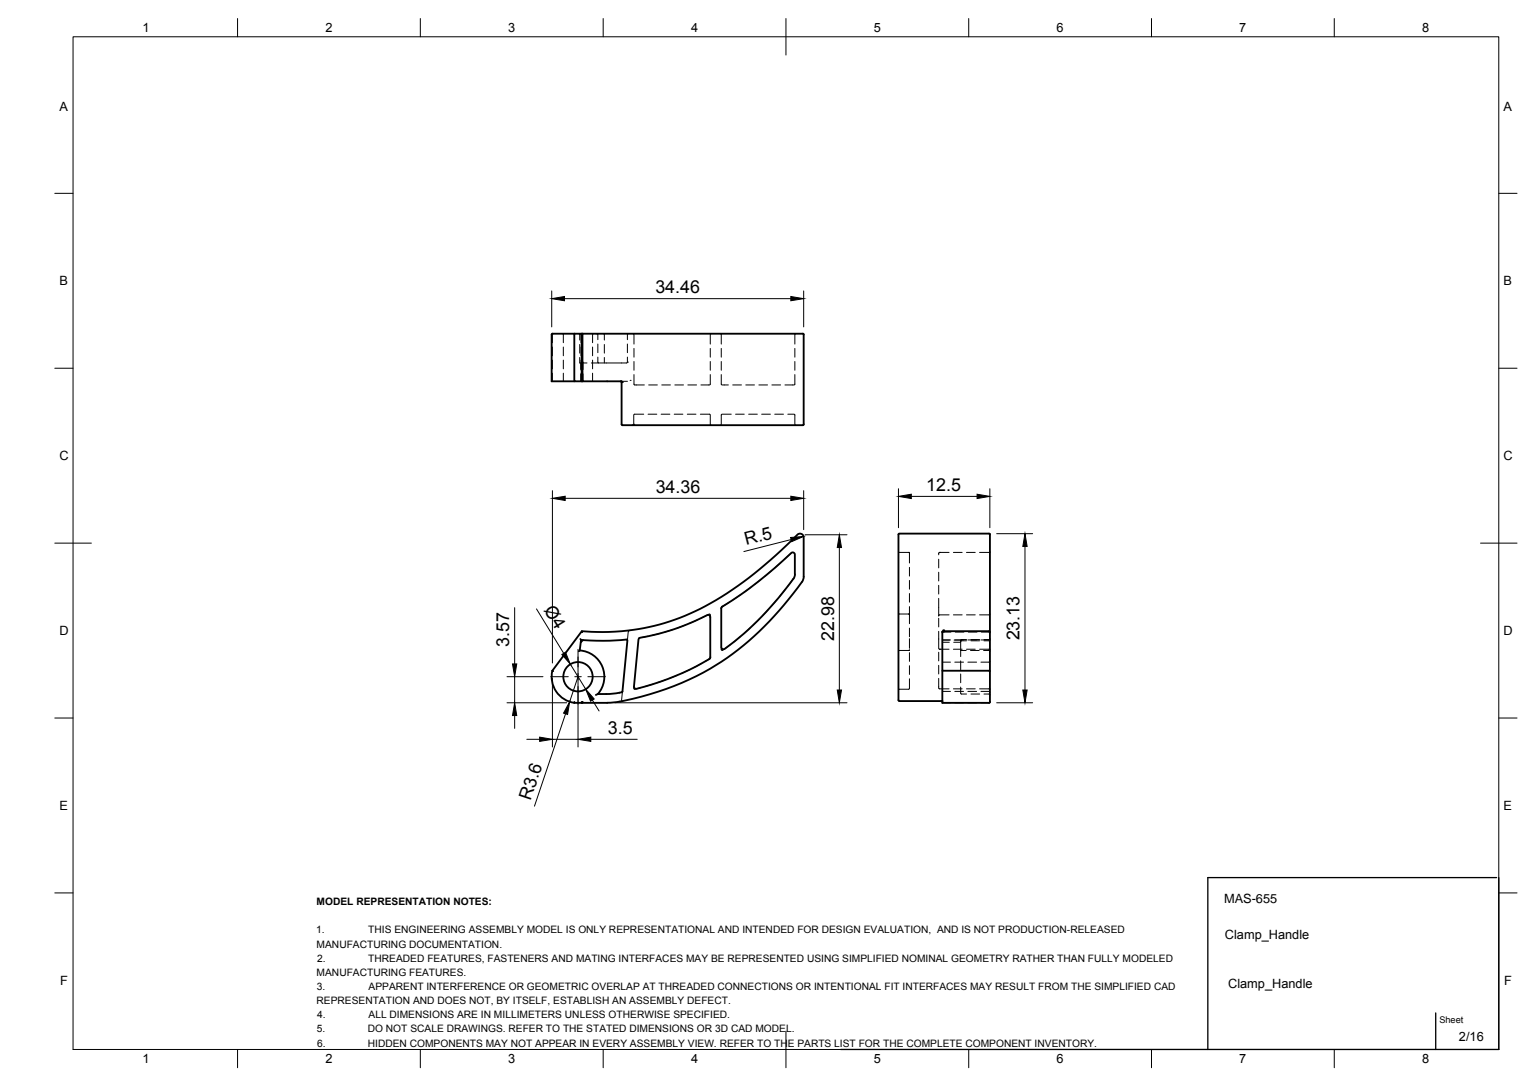
ISO-10303-21;
HEADER;
FILE_DESCRIPTION((''),'2;1');
FILE_NAME('Clamp_Handle.step','2026-10-09T11:34:15-07:00',(''),(''),'','','');
FILE_SCHEMA (('AUTOMOTIVE_DESIGN { 1 0 10303 214 3 1 1 }'));
ENDSEC;
DATA;
#10=MECHANICAL_DESIGN_GEOMETRIC_PRESENTATION_REPRESENTATION('',(#629),#117170);
#103=ELLIPSE('',#49876,30.621208525322,25.4809915026997) ;
#104=ELLIPSE('',#49877,31.5888201684124,25.5766704752798) ;
#105=ELLIPSE('',#49879,31.5675675201038,25.5487669653367) ;
#106=ELLIPSE('',#49885,0.87450775194086,0.752188335062039) ;
#107=ELLIPSE('',#49887,0.979448682193676,0.842450935309832) ;
#108=ELLIPSE('',#49892,0.26650610321202,0.226790790063564) ;
#109=ELLIPSE('',#49893,0.373108544497893,0.31750710609267) ;
#110=ELLIPSE('',#49894,0.874507751946099,0.752188335070988) ;
#111=ELLIPSE('',#49899,104.965032228634,60.1468662540866) ;
#112=ELLIPSE('',#49900,153.912764893179,72.1332927979209) ;
#113=ELLIPSE('',#49901,107.003369056671,53.394874735838) ;
#114=ELLIPSE('',#49903,0.944305135734821,0.812323833839972) ;
#115=ELLIPSE('',#49904,31.6658812357246,25.6468027651175) ;
#116=ELLIPSE('',#49905,33.3290082029849,26.9991094930833) ;
#117=ELLIPSE('',#49908,0.373067574458494,0.317497630618124) ;
#118=ELLIPSE('',#49909,87.539485717233,47.1288613191233) ;
#119=ELLIPSE('',#49910,28.9052201415572,24.2407648329214) ;
#120=ELLIPSE('',#49911,33.8387106683363,27.6581069858551) ;
#121=ELLIPSE('',#49912,32.4705877660237,26.389680540433) ;
#122=ELLIPSE('',#49913,119.941732153885,63.5628286542732) ;
#123=ELLIPSE('',#49920,0.266476838896091,0.226784021864154) ;
#124=ELLIPSE('',#49928,0.266476838896308,0.226784021864664) ;
#125=ELLIPSE('',#49936,0.120304939822837,0.120009764468753) ;
#126=ELLIPSE('',#49937,0.120304939823071,0.120009764469075) ;
#127=ELLIPSE('',#49944,32.9935493519598,26.6864661964081) ;
#128=ELLIPSE('',#49946,31.5675675494409,25.5487669922883) ;
#129=ELLIPSE('',#49953,1.04922792860613,0.902582037621626) ;
#130=ELLIPSE('',#49958,106.937521398911,53.4980353026644) ;
#131=ELLIPSE('',#49960,171.400384709509,76.7143149375333) ;
#132=ELLIPSE('',#49962,112.686599872101,62.8742365573781) ;
#133=ELLIPSE('',#49966,0.124835932303391,0.12) ;
#134=ELLIPSE('',#49972,106.937521398833,53.4980353026422) ;
#135=ELLIPSE('',#49973,26.7718235298462,13.2260955102084) ;
#136=ELLIPSE('',#49974,180.168079206207,78.5747283099703) ;
#137=ELLIPSE('',#49975,26.5629631306412,13.0416514063261) ;
#138=ELLIPSE('',#49997,34.0017819463872,27.818723289359) ;
#139=ELLIPSE('',#49999,33.6804890520093,27.5067870175508) ;
#140=ELLIPSE('',#50000,32.5228044782183,26.4447063399665) ;
#141=ELLIPSE('',#50001,32.6276108313175,26.5480371159551) ;
#142=ELLIPSE('',#50004,33.6121963166486,28.1464718973248) ;
#143=ELLIPSE('',#50007,34.1688903664586,27.9750858992831) ;
#144=ELLIPSE('',#50008,32.5764457907704,26.4940988115262) ;
#145=ELLIPSE('',#50009,121.638689200547,63.8567625922291) ;
#146=ELLIPSE('',#50011,133.068922302088,67.3695526852953) ;
#147=ELLIPSE('',#50017,110.759696058364,60.5332237301847) ;
#148=ELLIPSE('',#50022,26.0480895445502,18.516397692244) ;
#149=ELLIPSE('',#50026,112.783598469003,61.0762817351653) ;
#150=ELLIPSE('',#50031,89.0710500040395,47.3896547267835) ;
#151=ELLIPSE('',#50033,0.159886103339097,0.136070413122481) ;
#152=ELLIPSE('',#50037,29.4480227809696,24.8646228837011) ;
#153=ELLIPSE('',#50046,0.76956682169275,0.66192573483117) ;
#154=ELLIPSE('',#50052,0.159903661928928,0.13607447404265) ;
#155=ELLIPSE('',#50053,0.266506103215596,0.226790790070262) ;
#156=ELLIPSE('',#50061,0.129795981335339,0.124487164214877) ;
#157=ELLIPSE('',#50071,0.769566821716286,0.661925734873078) ;
#158=ELLIPSE('',#50073,0.874507751919452,0.75218833502354) ;
#159=ELLIPSE('',#50077,0.210854308776711,0.181549488975955) ;
#160=ELLIPSE('',#50081,0.874507751937288,0.752188335055131) ;
#161=ELLIPSE('',#50083,0.97944868220323,0.842450935327434) ;
#162=ELLIPSE('',#50090,160.893031132199,73.683653149258) ;
#163=ELLIPSE('',#50091,0.944305135733765,0.812323833838177) ;
#164=ELLIPSE('',#50093,107.003369056713,53.3948747358502) ;
#165=ELLIPSE('',#50103,0.129786651823771,0.12448808595579) ;
#166=ELLIPSE('',#50123,90.0915709695949,47.7382908134221) ;
#167=ELLIPSE('',#50124,89.6335580246405,47.7081104258241) ;
#168=ELLIPSE('',#50133,33.329008202931,26.9991094930345) ;
#169=ELLIPSE('',#50134,32.993549352048,26.6864661964888) ;
#170=ELLIPSE('',#50146,1.04922792859238,0.902582037596269) ;
#587=SHAPE_REPRESENTATION_RELATIONSHIP('SRR','None',#117242,#608) ;
#608=ADVANCED_BREP_SHAPE_REPRESENTATION('',(#650),#117150) ;
#629=STYLED_ITEM('',(#117355),#650) ;
#650=MANIFOLD_SOLID_BREP('Body1',#49058) ;
#671=FACE_BOUND('',#14121,.T.) ;
#672=FACE_BOUND('',#14122,.T.) ;
#673=FACE_BOUND('',#14123,.T.) ;
#674=FACE_BOUND('',#14124,.T.) ;
#675=FACE_BOUND('',#14239,.T.) ;
#676=FACE_BOUND('',#14240,.T.) ;
#677=FACE_BOUND('',#14304,.T.) ;
#678=FACE_BOUND('',#14305,.T.) ;
#895=B_SPLINE_CURVE_WITH_KNOTS('',3,(#75340,#75341,#75342,#75343),
 .UNSPECIFIED.,.F.,.F.,(4,4),(0.,0.0304960917345408),.UNSPECIFIED.) ;
#896=B_SPLINE_CURVE_WITH_KNOTS('',3,(#75345,#75346,#75347,#75348,#75349,
#75350),.UNSPECIFIED.,.F.,.F.,(4,2,4),(0.0304960917345408,0.0307213705840096,
0.0308468428281894),.UNSPECIFIED.) ;
#897=B_SPLINE_CURVE_WITH_KNOTS('',3,(#75351,#75352,#75353,#75354,#75355,
#75356),.UNSPECIFIED.,.F.,.F.,(4,2,4),(-0.0308468428281894,-0.0307213705840096,
0.),.UNSPECIFIED.) ;
#898=B_SPLINE_CURVE_WITH_KNOTS('',3,(#75428,#75429,#75430,#75431,#75432,
#75433,#75434,#75435,#75436,#75437),.UNSPECIFIED.,.F.,.F.,(4,2,2,2,4),(-9.50158063795107E-5,
-3.3802014536195E-10,0.0116383704253253,0.0168222452993766,0.0213033382245776),
 .UNSPECIFIED.) ;
#899=B_SPLINE_CURVE_WITH_KNOTS('',3,(#75438,#75439,#75440,#75441,#75442),
 .UNSPECIFIED.,.F.,.F.,(4,1,4),(0.0251851760390954,0.0320842381312984,0.0449179333838473),
 .UNSPECIFIED.) ;
#900=B_SPLINE_CURVE_WITH_KNOTS('',3,(#75443,#75444,#75445,#75446,#75447,
#75448),.UNSPECIFIED.,.F.,.F.,(4,1,1,4),(0.,0.5,0.714285714285714,1.),
 .UNSPECIFIED.) ;
#901=B_SPLINE_CURVE_WITH_KNOTS('',3,(#75474,#75475,#75476,#75477,#75478),
 .UNSPECIFIED.,.F.,.F.,(4,1,4),(-0.0228171701215865,-0.0097787952834712,
0.),.UNSPECIFIED.) ;
#902=B_SPLINE_CURVE_WITH_KNOTS('',3,(#75479,#75480,#75481,#75482,#75483,
#75484,#75485,#75486,#75487,#75488,#75489,#75490,#75491,#75492,#75493,#75494,
#75495,#75496,#75497),.UNSPECIFIED.,.F.,.F.,(4,3,3,3,3,3,4),(7.84710342600197E-9,
0.00635871960742978,0.00765411709399715,0.0097787952834712,0.0153829015724535,
0.0211032796709813,0.0228171889947661),.UNSPECIFIED.) ;
#903=B_SPLINE_CURVE_WITH_KNOTS('',3,(#75516,#75517,#75518,#75519,#75520),
 .UNSPECIFIED.,.F.,.F.,(4,1,4),(-1.,-0.571428571428571,0.),
 .UNSPECIFIED.) ;
#904=B_SPLINE_CURVE_WITH_KNOTS('',3,(#75589,#75590,#75591,#75592),
 .UNSPECIFIED.,.F.,.F.,(4,4),(-1.19261278278549,0.),.UNSPECIFIED.) ;
#905=B_SPLINE_CURVE_WITH_KNOTS('',3,(#75595,#75596,#75597,#75598),
 .UNSPECIFIED.,.F.,.F.,(4,4),(0.,1.19261278278549),.UNSPECIFIED.) ;
#906=B_SPLINE_CURVE_WITH_KNOTS('',3,(#75630,#75631,#75632,#75633,#75634,
#75635),.UNSPECIFIED.,.F.,.F.,(4,1,1,4),(-0.0977650255444303,-0.0698321611031645,
-0.0418992966618987,0.),.UNSPECIFIED.) ;
#907=B_SPLINE_CURVE_WITH_KNOTS('',3,(#75638,#75639,#75640,#75641,#75642,
#75643),.UNSPECIFIED.,.F.,.F.,(4,1,1,4),(0.,0.0418992966618987,0.0698321611031645,
0.0977650255444303),.UNSPECIFIED.) ;
#908=B_SPLINE_CURVE_WITH_KNOTS('',3,(#75698,#75699,#75700,#75701),
 .UNSPECIFIED.,.F.,.F.,(4,4),(-1.35181237759077,-5.11404103536248E-14),
 .UNSPECIFIED.) ;
#909=B_SPLINE_CURVE_WITH_KNOTS('',3,(#75702,#75703,#75704,#75705),
 .UNSPECIFIED.,.F.,.F.,(4,4),(5.11404103536248E-14,1.35181237759077),
 .UNSPECIFIED.) ;
#910=B_SPLINE_CURVE_WITH_KNOTS('',3,(#75737,#75738,#75739,#75740,#75741,
#75742),.UNSPECIFIED.,.F.,.F.,(4,1,1,4),(-0.0921161357255624,-0.0657972398039731,
-0.0394783438823839,0.),.UNSPECIFIED.) ;
#911=B_SPLINE_CURVE_WITH_KNOTS('',3,(#75745,#75746,#75747,#75748,#75749,
#75750),.UNSPECIFIED.,.F.,.F.,(4,1,1,4),(0.,0.0394783438823839,0.0657972398039731,
0.0921161357255624),.UNSPECIFIED.) ;
#912=B_SPLINE_CURVE_WITH_KNOTS('',3,(#75812,#75813,#75814,#75815,#75816,
#75817,#75818),.UNSPECIFIED.,.F.,.F.,(4,1,1,1,4),(-1.,-0.857142857142857,
-0.571428571428571,-0.285714285714286,0.),.UNSPECIFIED.) ;
#913=B_SPLINE_CURVE_WITH_KNOTS('',3,(#75829,#75830,#75831,#75832),
 .UNSPECIFIED.,.F.,.F.,(4,4),(-1.19778613661182,0.),.UNSPECIFIED.) ;
#914=B_SPLINE_CURVE_WITH_KNOTS('',3,(#75854,#75855,#75856,#75857,#75858),
 .UNSPECIFIED.,.F.,.F.,(4,1,4),(-1.5574419802933,-0.667475134411416,0.),
 .UNSPECIFIED.) ;
#915=B_SPLINE_CURVE_WITH_KNOTS('',3,(#75864,#75865,#75866,#75867,#75868,
#75869,#75870),.UNSPECIFIED.,.F.,.F.,(4,1,1,1,4),(3.75975382637766E-15,
0.0255939875922149,0.051187975184426,0.0639849689805315,0.0895789565727426),
 .UNSPECIFIED.) ;
#916=B_SPLINE_CURVE_WITH_KNOTS('',3,(#75872,#75873,#75874,#75875,#75876),
 .UNSPECIFIED.,.F.,.F.,(4,1,4),(-1.52552518986177,-0.653796509940758,0.),
 .UNSPECIFIED.) ;
#917=B_SPLINE_CURVE_WITH_KNOTS('',3,(#75878,#75879,#75880,#75881,#75882),
 .UNSPECIFIED.,.F.,.F.,(4,1,4),(-1.19232799652366,-0.510997712795854,0.),
 .UNSPECIFIED.) ;
#918=B_SPLINE_CURVE_WITH_KNOTS('',3,(#75900,#75901,#75902,#75903,#75904,
#75905),.UNSPECIFIED.,.F.,.F.,(4,1,1,4),(0.,0.0345437068826219,0.0575728448043699,
0.0806019827261179),.UNSPECIFIED.) ;
#919=B_SPLINE_CURVE_WITH_KNOTS('',3,(#75909,#75910,#75911,#75912,#75913),
 .UNSPECIFIED.,.F.,.F.,(4,1,4),(0.,0.0235485345716834,0.0549465806672613),
 .UNSPECIFIED.) ;
#920=B_SPLINE_CURVE_WITH_KNOTS('',3,(#75916,#75917,#75918,#75919,#75920,
#75921),.UNSPECIFIED.,.F.,.F.,(4,1,1,4),(4.3103929042364E-51,0.0368724376954248,
0.061454062825708,0.0860356879559912),.UNSPECIFIED.) ;
#921=B_SPLINE_CURVE_WITH_KNOTS('',3,(#75924,#75925,#75926,#75927,#75928,
#75929),.UNSPECIFIED.,.F.,.F.,(4,2,4),(-0.0257669909600073,0.,0.011519137396051),
 .UNSPECIFIED.) ;
#922=B_SPLINE_CURVE_WITH_KNOTS('',3,(#75935,#75936,#75937,#75938,#75939,
#75940,#75941),.UNSPECIFIED.,.F.,.F.,(4,1,1,1,4),(-0.0425072330863067,-0.030362309347362,
-0.0212536165431535,-0.00910869280420873,-1.83791533766654E-16),
 .UNSPECIFIED.) ;
#923=B_SPLINE_CURVE_WITH_KNOTS('',3,(#75945,#75946,#75947,#75948,#75949),
 .UNSPECIFIED.,.F.,.F.,(4,1,4),(-0.0304168573334205,-0.0130357960000373,
0.),.UNSPECIFIED.) ;
#924=B_SPLINE_CURVE_WITH_KNOTS('',3,(#76012,#76013,#76014,#76015),
 .UNSPECIFIED.,.F.,.F.,(4,4),(-0.465795144410571,-0.11054487910679),
 .UNSPECIFIED.) ;
#925=B_SPLINE_CURVE_WITH_KNOTS('',3,(#76047,#76048,#76049,#76050,#76051,
#76052),.UNSPECIFIED.,.F.,.F.,(4,1,1,4),(-0.0806019827261179,-0.0575728448043699,
-0.0345437068826219,0.),.UNSPECIFIED.) ;
#926=B_SPLINE_CURVE_WITH_KNOTS('',3,(#76084,#76085,#76086,#76087,#76088),
 .UNSPECIFIED.,.F.,.F.,(4,1,4),(-0.0549465806672613,-0.0235485345716834,
0.),.UNSPECIFIED.) ;
#927=B_SPLINE_CURVE_WITH_KNOTS('',3,(#76112,#76113,#76114,#76115),
 .UNSPECIFIED.,.F.,.F.,(4,4),(0.,0.963640330286854),.UNSPECIFIED.) ;
#928=B_SPLINE_CURVE_WITH_KNOTS('',3,(#76146,#76147,#76148,#76149,#76150,
#76151),.UNSPECIFIED.,.F.,.F.,(4,1,1,4),(-0.0860356879559912,-0.061454062825708,
-0.0368724376954248,-4.3103929042364E-51),.UNSPECIFIED.) ;
#929=B_SPLINE_CURVE_WITH_KNOTS('',3,(#76167,#76168,#76169,#76170,#76171,
#76172),.UNSPECIFIED.,.F.,.F.,(4,1,1,4),(0.,0.285714285714286,0.571428571428571,
1.),.UNSPECIFIED.) ;
#930=B_SPLINE_CURVE_WITH_KNOTS('',3,(#76184,#76185,#76186,#76187),
 .UNSPECIFIED.,.F.,.F.,(4,4),(0.11054487910679,0.465795144410571),
 .UNSPECIFIED.) ;
#931=B_SPLINE_CURVE_WITH_KNOTS('',3,(#76219,#76220,#76221,#76222,#76223,
#76224,#76225,#76226,#76227,#76228,#76229,#76230,#76231,#76232,#76233,#76234),
 .UNSPECIFIED.,.F.,.F.,(4,3,3,3,3,4),(-0.000158808056872058,0.,0.00496233024236406,
0.00971437347025351,0.0143645688442801,0.0189647476919275),
 .UNSPECIFIED.) ;
#932=B_SPLINE_CURVE_WITH_KNOTS('',3,(#76238,#76239,#76240,#76241,#76242,
#76243,#76244,#76245,#76246,#76247,#76248,#76249,#76250,#76251),
 .UNSPECIFIED.,.F.,.F.,(4,2,2,2,2,2,4),(-0.000100608577474137,3.68347560433932E-11,
0.00487642669195541,0.00843616962847088,0.0110941564927162,0.012526922262663,
0.0139424786869335),.UNSPECIFIED.) ;
#933=B_SPLINE_CURVE_WITH_KNOTS('',5,(#76349,#76350,#76351,#76352,#76353,
#76354,#76355,#76356,#76357),.UNSPECIFIED.,.F.,.F.,(6,1,1,1,6),(-0.568009935219888,
-0.5,-0.4,-0.3,-0.202504416334422),.UNSPECIFIED.) ;
#934=B_SPLINE_CURVE_WITH_KNOTS('',5,(#76385,#76386,#76387,#76388,#76389,
#76390,#76391,#76392,#76393,#76394),.UNSPECIFIED.,.F.,.F.,(6,1,1,1,1,6),
(-0.970637147863782,-0.9,-0.8,-0.7,-0.6,-0.568009935219903),
 .UNSPECIFIED.) ;
#935=B_SPLINE_CURVE_WITH_KNOTS('',3,(#76432,#76433,#76434,#76435,#76436,
#76437,#76438),.UNSPECIFIED.,.F.,.F.,(4,1,1,1,4),(-1.,-0.857142857142857,
-0.571428571428571,-0.285714285714286,0.),.UNSPECIFIED.) ;
#936=B_SPLINE_CURVE_WITH_KNOTS('',5,(#76493,#76494,#76495,#76496,#76497,
#76498,#76499,#76500,#76501,#76502),.UNSPECIFIED.,.F.,.F.,(6,1,1,1,1,6),
(0.504846387196225,0.6,0.7,0.8,0.9,0.98854312859838),.UNSPECIFIED.) ;
#937=B_SPLINE_CURVE_WITH_KNOTS('',3,(#76625,#76626,#76627,#76628,#76629,
#76630,#76631,#76632,#76633,#76634,#76635,#76636,#76637,#76638,#76639,#76640,
#76641,#76642,#76643,#76644,#76645,#76646,#76647,#76648,#76649),
 .UNSPECIFIED.,.F.,.F.,(4,3,3,3,3,3,3,3,4),(-0.000166044934212311,0.,0.00279435046699232,
0.00557076822786895,0.00922713992765633,0.0104440756657821,0.014060635831078,
0.0150050171466993,0.0194197313345285),.UNSPECIFIED.) ;
#938=B_SPLINE_CURVE_WITH_KNOTS('',3,(#76675,#76676,#76677,#76678,#76679),
 .UNSPECIFIED.,.F.,.F.,(4,1,4),(0.,0.66747373630185,1.55743871803765),
 .UNSPECIFIED.) ;
#939=B_SPLINE_CURVE_WITH_KNOTS('',3,(#76771,#76772,#76773,#76774,#76775,
#76776),.UNSPECIFIED.,.F.,.F.,(4,2,4),(0.,0.0885040710835739,0.177008142167353),
 .UNSPECIFIED.) ;
#940=B_SPLINE_CURVE_WITH_KNOTS('',3,(#76795,#76796,#76797,#76798,#76799,
#76800,#76801,#76802,#76803,#76804,#76805,#76806,#76807,#76808),
 .UNSPECIFIED.,.F.,.F.,(4,2,2,2,2,2,4),(-0.0904118247922396,-0.0900035304718211,
-0.0717391824762992,-0.0592522695262226,-0.052421636870123,-0.0483060494744438,
-0.0450017652359281),.UNSPECIFIED.) ;
#941=B_SPLINE_CURVE_WITH_KNOTS('',3,(#76811,#76812,#76813,#76814,#76815,
#76816,#76817,#76818,#76819,#76820,#76821,#76822,#76823,#76824),
 .UNSPECIFIED.,.F.,.F.,(4,2,2,2,2,2,4),(-0.000229805914918867,0.,0.0057259760846815,
0.0111063849697663,0.0162643432934294,0.0200672254121506,0.0233750704027966),
 .UNSPECIFIED.) ;
#942=B_SPLINE_CURVE_WITH_KNOTS('',3,(#76853,#76854,#76855,#76856,#76857),
 .UNSPECIFIED.,.F.,.F.,(4,1,4),(0.,0.571428571428571,1.),.UNSPECIFIED.) ;
#943=B_SPLINE_CURVE_WITH_KNOTS('',3,(#76916,#76917,#76918,#76919,#76920,
#76921),.UNSPECIFIED.,.F.,.F.,(4,1,1,4),(0.,0.285714285714286,0.571428571428571,
1.),.UNSPECIFIED.) ;
#944=B_SPLINE_CURVE_WITH_KNOTS('',3,(#77040,#77041,#77042,#77043,#77044,
#77045,#77046,#77047,#77048,#77049,#77050,#77051,#77052,#77053),
 .UNSPECIFIED.,.F.,.F.,(4,2,2,2,2,2,4),(-0.000109725029838064,0.,0.00573281981816143,
0.011229162404333,0.0168245500650057,0.0201739980781553,0.0234334300413515),
 .UNSPECIFIED.) ;
#945=B_SPLINE_CURVE_WITH_KNOTS('',3,(#77151,#77152,#77153,#77154,#77155,
#77156,#77157,#77158,#77159,#77160),.UNSPECIFIED.,.F.,.F.,(4,2,2,2,4),(-0.0827921863495745,
-0.0783024654164144,-0.0738127444832543,-0.0678611473372446,-0.061909550191235),
 .UNSPECIFIED.) ;
#946=B_SPLINE_CURVE_WITH_KNOTS('',3,(#77234,#77235,#77236,#77237,#77238,
#77239,#77240,#77241,#77242,#77243,#77244,#77245),.UNSPECIFIED.,.F.,.F.,
(4,2,2,2,2,4),(0.,0.00262343669493822,0.00608267202291995,0.0109373875288971,
0.016217047415382,0.021823180377612),.UNSPECIFIED.) ;
#947=B_SPLINE_CURVE_WITH_KNOTS('',3,(#77306,#77307,#77308,#77309,#77310),
 .UNSPECIFIED.,.F.,.F.,(4,1,4),(-0.0345437068826239,-0.017271853441312,
0.),.UNSPECIFIED.) ;
#948=B_SPLINE_CURVE_WITH_KNOTS('',3,(#77395,#77396,#77397,#77398,#77399,
#77400),.UNSPECIFIED.,.F.,.F.,(4,1,1,4),(-0.0368724376954292,-0.0263374554967351,
-0.0158024732980411,0.),.UNSPECIFIED.) ;
#949=B_SPLINE_CURVE_WITH_KNOTS('',3,(#77401,#77402,#77403,#77404,#77405,
#77406),.UNSPECIFIED.,.F.,.F.,(4,1,1,4),(0.,0.0158024732980411,0.0263374554967351,
0.0368724376954292),.UNSPECIFIED.) ;
#950=B_SPLINE_CURVE_WITH_KNOTS('',3,(#77431,#77432,#77433,#77434),
 .UNSPECIFIED.,.F.,.F.,(4,4),(0.,0.971129055990219),.UNSPECIFIED.) ;
#951=B_SPLINE_CURVE_WITH_KNOTS('',3,(#77463,#77464,#77465,#77466,#77467),
 .UNSPECIFIED.,.F.,.F.,(4,1,4),(-0.0235485345716821,-0.0100922291021495,
0.),.UNSPECIFIED.) ;
#952=B_SPLINE_CURVE_WITH_KNOTS('',3,(#77468,#77469,#77470,#77471,#77472),
 .UNSPECIFIED.,.F.,.F.,(4,1,4),(0.,0.0100922291021495,0.0235485345716821),
 .UNSPECIFIED.) ;
#953=B_SPLINE_CURVE_WITH_KNOTS('',3,(#77511,#77512,#77513,#77514,#77515,
#77516),.UNSPECIFIED.,.F.,.F.,(4,1,1,4),(-0.0394783438823839,-0.0225590536470765,
-0.0112795268235383,0.),.UNSPECIFIED.) ;
#954=B_SPLINE_CURVE_WITH_KNOTS('',3,(#77519,#77520,#77521,#77522,#77523,
#77524),.UNSPECIFIED.,.F.,.F.,(4,1,1,4),(0.,0.0112795268235383,0.0225590536470765,
0.0394783438823839),.UNSPECIFIED.) ;
#955=B_SPLINE_CURVE_WITH_KNOTS('',3,(#77545,#77546,#77547,#77548),
 .UNSPECIFIED.,.F.,.F.,(4,4),(-1.34425818567182,0.),.UNSPECIFIED.) ;
#956=B_SPLINE_CURVE_WITH_KNOTS('',3,(#77551,#77552,#77553,#77554),
 .UNSPECIFIED.,.F.,.F.,(4,4),(0.,1.34425818567182),.UNSPECIFIED.) ;
#957=B_SPLINE_CURVE_WITH_KNOTS('',3,(#77619,#77620,#77621,#77622,#77623,
#77624,#77625),.UNSPECIFIED.,.F.,.F.,(4,1,1,1,4),(-0.0418992966619001,-0.0359136828530572,
-0.0239424552353715,-0.0119712276176857,0.),.UNSPECIFIED.) ;
#958=B_SPLINE_CURVE_WITH_KNOTS('',3,(#77648,#77649,#77650,#77651),
 .UNSPECIFIED.,.F.,.F.,(4,4),(0.,1.19778613661182),.UNSPECIFIED.) ;
#959=B_SPLINE_CURVE_WITH_KNOTS('',3,(#77748,#77749,#77750,#77751,#77752),
 .UNSPECIFIED.,.F.,.F.,(4,1,4),(-0.0247639318112814,-0.0106131136334063,
0.),.UNSPECIFIED.) ;
#960=B_SPLINE_CURVE_WITH_KNOTS('',3,(#77798,#77799,#77800,#77801),
 .UNSPECIFIED.,.F.,.F.,(4,4),(0.0229372865431325,1.40205259514116),
 .UNSPECIFIED.) ;
#961=B_SPLINE_CURVE_WITH_KNOTS('',3,(#77804,#77805,#77806,#77807,#77808,
#77809,#77810),.UNSPECIFIED.,.F.,.F.,(4,3,4),(-0.978678731718532,-0.545479769376514,
-0.539016918864981),.UNSPECIFIED.) ;
#962=B_SPLINE_CURVE_WITH_KNOTS('',3,(#77878,#77879,#77880,#77881,#77882,
#77883,#77884),.UNSPECIFIED.,.F.,.F.,(4,1,1,1,4),(-0.0418992966619021,-0.0299280690442158,
-0.0179568414265295,-0.00598561380884316,0.),.UNSPECIFIED.) ;
#963=B_SPLINE_CURVE_WITH_KNOTS('',3,(#77887,#77888,#77889,#77890,#77891,
#77892,#77893),.UNSPECIFIED.,.F.,.F.,(4,1,1,1,4),(0.,0.285714285714286,
0.571428571428571,0.857142857142857,1.),.UNSPECIFIED.) ;
#964=B_SPLINE_CURVE_WITH_KNOTS('',3,(#77914,#77915,#77916,#77917),
 .UNSPECIFIED.,.F.,.F.,(4,4),(-1.20789221798527,0.),.UNSPECIFIED.) ;
#965=B_SPLINE_CURVE_WITH_KNOTS('',3,(#77918,#77919,#77920,#77921),
 .UNSPECIFIED.,.F.,.F.,(4,4),(0.,1.20789221798527),.UNSPECIFIED.) ;
#966=B_SPLINE_CURVE_WITH_KNOTS('',3,(#77961,#77962,#77963,#77964,#77965,
#77966),.UNSPECIFIED.,.F.,.F.,(4,1,1,4),(-0.0251311022767196,-0.0224490289603943,
-0.0149660193069295,0.),.UNSPECIFIED.) ;
#967=B_SPLINE_CURVE_WITH_KNOTS('',3,(#77970,#77971,#77972,#77973,#77974,
#77975,#77976),.UNSPECIFIED.,.F.,.F.,(4,1,1,1,4),(-1.,-0.785714285714286,
-0.5,-0.285714285714286,0.),.UNSPECIFIED.) ;
#968=B_SPLINE_CURVE_WITH_KNOTS('',3,(#77979,#77980,#77981,#77982,#77983),
 .UNSPECIFIED.,.F.,.F.,(4,1,4),(-0.0523810675742533,-0.0374150482673238,
-0.027172373910007),.UNSPECIFIED.) ;
#969=B_SPLINE_CURVE_WITH_KNOTS('',3,(#78021,#78022,#78023,#78024),
 .UNSPECIFIED.,.F.,.F.,(4,4),(0.0231068825027873,1.41003451675495),
 .UNSPECIFIED.) ;
#970=B_SPLINE_CURVE_WITH_KNOTS('',3,(#78027,#78028,#78029,#78030),
 .UNSPECIFIED.,.F.,.F.,(4,4),(-1.41003451675495,-0.0231068825027873),
 .UNSPECIFIED.) ;
#971=B_SPLINE_CURVE_WITH_KNOTS('',3,(#78093,#78094,#78095,#78096,#78097,
#78098),.UNSPECIFIED.,.F.,.F.,(4,1,1,4),(-0.0977650255444333,-0.0698321611031666,
-0.0418992966619,0.),.UNSPECIFIED.) ;
#972=B_SPLINE_CURVE_WITH_KNOTS('',3,(#78101,#78102,#78103,#78104,#78105,
#78106),.UNSPECIFIED.,.F.,.F.,(4,1,1,4),(0.,0.0418992966619,0.0698321611031666,
0.0977650255444333),.UNSPECIFIED.) ;
#973=B_SPLINE_CURVE_WITH_KNOTS('',3,(#78127,#78128,#78129,#78130),
 .UNSPECIFIED.,.F.,.F.,(4,4),(-1.20265740584169,0.),.UNSPECIFIED.) ;
#974=B_SPLINE_CURVE_WITH_KNOTS('',3,(#78131,#78132,#78133,#78134),
 .UNSPECIFIED.,.F.,.F.,(4,4),(0.,1.20265740584169),.UNSPECIFIED.) ;
#975=B_SPLINE_CURVE_WITH_KNOTS('',3,(#78186,#78187,#78188,#78189,#78190),
 .UNSPECIFIED.,.F.,.F.,(4,1,4),(0.,0.0104089910116412,0.0242876456938294),
 .UNSPECIFIED.) ;
#976=B_SPLINE_CURVE_WITH_KNOTS('',3,(#78192,#78193,#78194,#78195,#78196),
 .UNSPECIFIED.,.F.,.F.,(4,1,4),(-1.16825744734596,-0.500681763148267,0.),
 .UNSPECIFIED.) ;
#977=B_SPLINE_CURVE_WITH_KNOTS('',3,(#78198,#78199,#78200,#78201,#78202),
 .UNSPECIFIED.,.F.,.F.,(4,1,4),(-1.52552518986177,-0.653796509940757,0.),
 .UNSPECIFIED.) ;
#978=B_SPLINE_CURVE_WITH_KNOTS('',3,(#78204,#78205,#78206,#78207,#78208,
#78209,#78210),.UNSPECIFIED.,.F.,.F.,(4,1,1,1,4),(0.,0.0255939875922127,
0.038390981388319,0.0639849689805316,0.0895789565727443),.UNSPECIFIED.) ;
#979=B_SPLINE_CURVE_WITH_KNOTS('',3,(#78216,#78217,#78218,#78219,#78220),
 .UNSPECIFIED.,.F.,.F.,(4,1,4),(-1.55743871803765,-0.66747373630185,0.),
 .UNSPECIFIED.) ;
#980=B_SPLINE_CURVE_WITH_KNOTS('',3,(#78226,#78227,#78228,#78229,#78230,
#78231,#78232),.UNSPECIFIED.,.F.,.F.,(4,1,1,1,4),(-0.0459218921195416,-0.0328013515139583,
-0.0229609460597708,-0.00984040545418749,0.),.UNSPECIFIED.) ;
#981=B_SPLINE_CURVE_WITH_KNOTS('',3,(#78234,#78235,#78236,#78237),
 .UNSPECIFIED.,.F.,.F.,(4,4),(-1.13243225761785,-0.0170557641123888),
 .UNSPECIFIED.) ;
#982=B_SPLINE_CURVE_WITH_KNOTS('',3,(#78239,#78240,#78241,#78242,#78243),
 .UNSPECIFIED.,.F.,.F.,(4,1,4),(-0.0245704597956453,-0.0105301970552765,
0.),.UNSPECIFIED.) ;
#983=B_SPLINE_CURVE_WITH_KNOTS('',3,(#78247,#78248,#78249,#78250,#78251,
#78252,#78253),.UNSPECIFIED.,.F.,.F.,(4,1,1,1,4),(-0.0493631644051633,-0.0352594031465452,
-0.0211556418879271,-0.0141037612586181,0.),.UNSPECIFIED.) ;
#984=B_SPLINE_CURVE_WITH_KNOTS('',3,(#78255,#78256,#78257,#78258),
 .UNSPECIFIED.,.F.,.F.,(4,4),(-1.02674783308136,-0.019875255616694),
 .UNSPECIFIED.) ;
#985=B_SPLINE_CURVE_WITH_KNOTS('',3,(#78260,#78261,#78262,#78263,#78264),
 .UNSPECIFIED.,.F.,.F.,(4,1,4),(-0.0315062771267664,-0.0180035869295808,
0.),.UNSPECIFIED.) ;
#986=B_SPLINE_CURVE_WITH_KNOTS('',3,(#78306,#78307,#78308,#78309,#78310,
#78311,#78312),.UNSPECIFIED.,.F.,.F.,(4,1,1,1,4),(0.,0.285714285714286,
0.5,0.785714285714286,1.),.UNSPECIFIED.) ;
#987=B_SPLINE_CURVE_WITH_KNOTS('',3,(#78395,#78396,#78397,#78398,#78399),
 .UNSPECIFIED.,.F.,.F.,(4,1,4),(-1.,-0.571428571428571,0.),
 .UNSPECIFIED.) ;
#988=B_SPLINE_CURVE_WITH_KNOTS('',3,(#78445,#78446,#78447,#78448),
 .UNSPECIFIED.,.F.,.F.,(4,4),(-1.03467847166523,-0.020008660331873),
 .UNSPECIFIED.) ;
#989=B_SPLINE_CURVE_WITH_KNOTS('',3,(#78449,#78450,#78451,#78452),
 .UNSPECIFIED.,.F.,.F.,(4,4),(0.020008660331873,1.03467846891799),
 .UNSPECIFIED.) ;
#990=B_SPLINE_CURVE_WITH_KNOTS('',3,(#78491,#78492,#78493,#78494,#78495,
#78496,#78497),.UNSPECIFIED.,.F.,.F.,(4,1,1,1,4),(0.,0.00984040545418749,
0.0229609460597708,0.0328013515139583,0.0459218921195416),.UNSPECIFIED.) ;
#991=B_SPLINE_CURVE_WITH_KNOTS('',3,(#78547,#78548,#78549,#78550),
 .UNSPECIFIED.,.F.,.F.,(4,4),(-1.12511677037933,-0.0169663179244005),
 .UNSPECIFIED.) ;
#992=B_SPLINE_CURVE_WITH_KNOTS('',3,(#78610,#78611,#78612,#78613),
 .UNSPECIFIED.,.F.,.F.,(4,4),(0.019875255616694,1.02674783308136),
 .UNSPECIFIED.) ;
#993=B_SPLINE_CURVE_WITH_KNOTS('',3,(#78678,#78679,#78680,#78681,#78682,
#78683,#78684,#78685,#78686,#78687,#78688,#78689),.UNSPECIFIED.,.F.,.F.,
(4,2,2,2,2,4),(-0.0228953324052163,-0.0161953944372489,-0.0102387878782572,
-0.00528256227931829,-0.00262036469686939,0.),.UNSPECIFIED.) ;
#994=B_SPLINE_CURVE_WITH_KNOTS('',3,(#78694,#78695,#78696,#78697,#78698,
#78699),.UNSPECIFIED.,.F.,.F.,(4,2,4),(-0.129892307653464,0.,0.00748019188171517),
 .UNSPECIFIED.) ;
#995=B_SPLINE_CURVE_WITH_KNOTS('',3,(#78941,#78942,#78943,#78944,#78945,
#78946,#78947),.UNSPECIFIED.,.F.,.F.,(4,1,1,1,4),(0.,0.285714285714286,
0.571428571428571,0.857142857142857,1.),.UNSPECIFIED.) ;
#996=B_SPLINE_CURVE_WITH_KNOTS('',5,(#78975,#78976,#78977,#78978,#78979,
#78980,#78981,#78982,#78983,#78984),.UNSPECIFIED.,.F.,.F.,(6,1,1,1,1,6),
(0.568009935219903,0.6,0.7,0.8,0.9,0.970637147863782),.UNSPECIFIED.) ;
#997=B_SPLINE_CURVE_WITH_KNOTS('',3,(#79011,#79012,#79013,#79014,#79015),
 .UNSPECIFIED.,.F.,.F.,(4,1,4),(0.,0.500681763148267,1.16825744734596),
 .UNSPECIFIED.) ;
#1789=B_SPLINE_SURFACE_WITH_KNOTS('',3,3,((#75312,#75313,#75314,#75315,
#75316,#75317),(#75318,#75319,#75320,#75321,#75322,#75323),(#75324,#75325,
#75326,#75327,#75328,#75329),(#75330,#75331,#75332,#75333,#75334,#75335)),
 .UNSPECIFIED.,.F.,.F.,.F.,(4,4),(4,2,4),(0.,1.),(-0.0308468428281894,-0.0307213705840096,
0.),.UNSPECIFIED.) ;
#1790=B_SPLINE_SURFACE_WITH_KNOTS('',3,3,((#75357,#75358,#75359,#75360),
(#75361,#75362,#75363,#75364),(#75365,#75366,#75367,#75368),(#75369,#75370,
#75371,#75372),(#75373,#75374,#75375,#75376)),.UNSPECIFIED.,.F.,.F.,.F.,
(4,1,4),(4,4),(0.,0.571428571428571,1.),(0.,0.00956620372314311),
 .UNSPECIFIED.) ;
#1791=B_SPLINE_SURFACE_WITH_KNOTS('',3,3,((#75391,#75392,#75393,#75394,
#75395,#75396,#75397),(#75398,#75399,#75400,#75401,#75402,#75403,#75404),
(#75405,#75406,#75407,#75408,#75409,#75410,#75411),(#75412,#75413,#75414,
#75415,#75416,#75417,#75418),(#75419,#75420,#75421,#75422,#75423,#75424,
#75425)),.UNSPECIFIED.,.F.,.F.,.F.,(4,1,4),(4,1,1,1,4),(0.,0.571428571428571,
1.),(-7.39408534400354E-14,0.00962527143933775,0.0224589666918867,0.0320842381312984,
0.0449179333838473),.UNSPECIFIED.) ;
#1792=B_SPLINE_SURFACE_WITH_KNOTS('',3,3,((#75449,#75450,#75451,#75452,
#75453),(#75454,#75455,#75456,#75457,#75458),(#75459,#75460,#75461,#75462,
#75463),(#75464,#75465,#75466,#75467,#75468),(#75469,#75470,#75471,#75472,
#75473)),.UNSPECIFIED.,.F.,.F.,.F.,(4,1,4),(4,1,4),(0.,0.571428571428571,
1.),(0.,0.0097787952834712,0.0228171889947661),.UNSPECIFIED.) ;
#1793=B_SPLINE_SURFACE_WITH_KNOTS('',3,1,((#75504,#75505),(#75506,#75507),
(#75508,#75509),(#75510,#75511),(#75512,#75513)),.UNSPECIFIED.,.F.,.F.,
 .F.,(4,1,4),(2,2),(0.,0.571428571428571,1.),(0.,0.72),.UNSPECIFIED.) ;
#1794=B_SPLINE_SURFACE_WITH_KNOTS('',3,3,((#75521,#75522,#75523,#75524),
(#75525,#75526,#75527,#75528),(#75529,#75530,#75531,#75532),(#75533,#75534,
#75535,#75536)),.UNSPECIFIED.,.F.,.F.,.F.,(4,4),(4,4),(0.,0.520585033056564),
(0.,0.0240718680289287),.UNSPECIFIED.) ;
#1795=B_SPLINE_SURFACE_WITH_KNOTS('',3,3,((#75540,#75541,#75542,#75543),
(#75544,#75545,#75546,#75547),(#75548,#75549,#75550,#75551),(#75552,#75553,
#75554,#75555),(#75556,#75557,#75558,#75559)),.UNSPECIFIED.,.F.,.F.,.F.,
(4,1,4),(4,4),(0.,0.571428571428571,1.),(0.,0.276406121061607),
 .UNSPECIFIED.) ;
#1796=B_SPLINE_SURFACE_WITH_KNOTS('',3,3,((#75565,#75566,#75567,#75568),
(#75569,#75570,#75571,#75572),(#75573,#75574,#75575,#75576),(#75577,#75578,
#75579,#75580),(#75581,#75582,#75583,#75584)),.UNSPECIFIED.,.F.,.F.,.F.,
(4,1,4),(4,4),(0.,0.571428571428571,1.),(0.,1.19261278278549),
 .UNSPECIFIED.) ;
#1797=B_SPLINE_SURFACE_WITH_KNOTS('',3,3,((#75599,#75600,#75601,#75602,
#75603,#75604),(#75605,#75606,#75607,#75608,#75609,#75610),(#75611,#75612,
#75613,#75614,#75615,#75616),(#75617,#75618,#75619,#75620,#75621,#75622),
(#75623,#75624,#75625,#75626,#75627,#75628)),.UNSPECIFIED.,.F.,.F.,.F.,
(4,1,4),(4,1,1,4),(0.,0.571428571428571,1.),(0.,0.0418992966618987,0.0698321611031645,
0.0977650255444303),.UNSPECIFIED.) ;
#1798=B_SPLINE_SURFACE_WITH_KNOTS('',3,3,((#75650,#75651,#75652,#75653),
(#75654,#75655,#75656,#75657),(#75658,#75659,#75660,#75661),(#75662,#75663,
#75664,#75665),(#75666,#75667,#75668,#75669)),.UNSPECIFIED.,.F.,.F.,.F.,
(4,1,4),(4,4),(0.,0.571428571428571,1.),(0.,0.0709441843098362),
 .UNSPECIFIED.) ;
#1799=B_SPLINE_SURFACE_WITH_KNOTS('',3,3,((#75675,#75676,#75677,#75678),
(#75679,#75680,#75681,#75682),(#75683,#75684,#75685,#75686),(#75687,#75688,
#75689,#75690),(#75691,#75692,#75693,#75694)),.UNSPECIFIED.,.F.,.F.,.F.,
(4,1,4),(4,4),(0.,0.571428571428571,1.),(5.11404103536248E-14,1.35181237759077),
 .UNSPECIFIED.) ;
#1800=B_SPLINE_SURFACE_WITH_KNOTS('',3,3,((#75706,#75707,#75708,#75709,
#75710,#75711),(#75712,#75713,#75714,#75715,#75716,#75717),(#75718,#75719,
#75720,#75721,#75722,#75723),(#75724,#75725,#75726,#75727,#75728,#75729),
(#75730,#75731,#75732,#75733,#75734,#75735)),.UNSPECIFIED.,.F.,.F.,.F.,
(4,1,4),(4,1,1,4),(0.,0.571428571428571,1.),(0.,0.0394783438823839,0.0657972398039731,
0.0921161357255624),.UNSPECIFIED.) ;
#1801=B_SPLINE_SURFACE_WITH_KNOTS('',3,3,((#75757,#75758,#75759,#75760),
(#75761,#75762,#75763,#75764),(#75765,#75766,#75767,#75768),(#75769,#75770,
#75771,#75772),(#75773,#75774,#75775,#75776)),.UNSPECIFIED.,.F.,.F.,.F.,
(4,1,4),(4,4),(-8.29172718649439E-5,0.571428571428571,1.),(-8.29172718649439E-5,
0.0433131895212127),.UNSPECIFIED.) ;
#1802=B_SPLINE_SURFACE_WITH_KNOTS('',3,1,((#75779,#75780),(#75781,#75782),
(#75783,#75784),(#75785,#75786)),.UNSPECIFIED.,.F.,.F.,.F.,(4,4),(2,2),
(0.,1.),(0.,0.8112),.UNSPECIFIED.) ;
#1803=B_SPLINE_SURFACE_WITH_KNOTS('',3,1,((#75796,#75797),(#75798,#75799),
(#75800,#75801),(#75802,#75803),(#75804,#75805),(#75806,#75807),(#75808,
#75809)),.UNSPECIFIED.,.F.,.F.,.F.,(4,1,1,1,4),(2,2),(0.,0.285714285714286,
0.571428571428571,0.857142857142857,1.),(0.,0.8112),.UNSPECIFIED.) ;
#1804=B_SPLINE_SURFACE_WITH_KNOTS('',3,1,((#75819,#75820),(#75821,#75822),
(#75823,#75824),(#75825,#75826)),.UNSPECIFIED.,.F.,.F.,.F.,(4,4),(2,2),
(0.597473964327042,0.930240743465184),(0.,1.50203770750399),
 .UNSPECIFIED.) ;
#1805=B_SPLINE_SURFACE_WITH_KNOTS('',3,3,((#75967,#75968,#75969,#75970),
(#75971,#75972,#75973,#75974),(#75975,#75976,#75977,#75978),(#75979,#75980,
#75981,#75982),(#75983,#75984,#75985,#75986)),.UNSPECIFIED.,.F.,.F.,.F.,
(4,1,4),(4,4),(-8.18731696806902E-5,0.571428571428571,1.),(-8.18731696802306E-5,
0.0432139508227142),.UNSPECIFIED.) ;
#1806=B_SPLINE_SURFACE_WITH_KNOTS('',3,3,((#75990,#75991,#75992,#75993),
(#75994,#75995,#75996,#75997),(#75998,#75999,#76000,#76001),(#76002,#76003,
#76004,#76005),(#76006,#76007,#76008,#76009)),.UNSPECIFIED.,.F.,.F.,.F.,
(4,1,4),(4,4),(0.,0.571428571428571,1.),(2.25690506700109E-10,1.07931701789601),
 .UNSPECIFIED.) ;
#1807=B_SPLINE_SURFACE_WITH_KNOTS('',3,3,((#76016,#76017,#76018,#76019,
#76020,#76021),(#76022,#76023,#76024,#76025,#76026,#76027),(#76028,#76029,
#76030,#76031,#76032,#76033),(#76034,#76035,#76036,#76037,#76038,#76039),
(#76040,#76041,#76042,#76043,#76044,#76045)),.UNSPECIFIED.,.F.,.F.,.F.,
(4,1,4),(4,1,1,4),(0.,0.571428571428571,1.),(0.,0.0345437068826219,0.0575728448043699,
0.0806019827261179),.UNSPECIFIED.) ;
#1808=B_SPLINE_SURFACE_WITH_KNOTS('',3,3,((#76058,#76059,#76060,#76061,
#76062),(#76063,#76064,#76065,#76066,#76067),(#76068,#76069,#76070,#76071,
#76072),(#76073,#76074,#76075,#76076,#76077),(#76078,#76079,#76080,#76081,
#76082)),.UNSPECIFIED.,.F.,.F.,.F.,(4,1,4),(4,1,4),(0.,0.571428571428571,
1.),(0.,0.0235485345716834,0.0549465806672613),.UNSPECIFIED.) ;
#1809=B_SPLINE_SURFACE_WITH_KNOTS('',3,3,((#76090,#76091,#76092,#76093),
(#76094,#76095,#76096,#76097),(#76098,#76099,#76100,#76101),(#76102,#76103,
#76104,#76105),(#76106,#76107,#76108,#76109)),.UNSPECIFIED.,.F.,.F.,.F.,
(4,1,4),(4,4),(0.,0.571428571428571,1.),(0.,0.963640330286854),
 .UNSPECIFIED.) ;
#1810=B_SPLINE_SURFACE_WITH_KNOTS('',3,3,((#76116,#76117,#76118,#76119,
#76120,#76121),(#76122,#76123,#76124,#76125,#76126,#76127),(#76128,#76129,
#76130,#76131,#76132,#76133),(#76134,#76135,#76136,#76137,#76138,#76139),
(#76140,#76141,#76142,#76143,#76144,#76145)),.UNSPECIFIED.,.F.,.F.,.F.,
(4,1,4),(4,1,1,4),(0.,0.571428571428571,1.),(4.3103929042364E-51,0.0368724376954248,
0.061454062825708,0.0860356879559912),.UNSPECIFIED.) ;
#1811=B_SPLINE_SURFACE_WITH_KNOTS('',3,1,((#76152,#76153),(#76154,#76155),
(#76156,#76157),(#76158,#76159),(#76160,#76161),(#76162,#76163)),
 .UNSPECIFIED.,.F.,.F.,.F.,(4,1,1,4),(2,2),(0.,0.285714285714286,0.571428571428571,
1.),(0.,0.8112),.UNSPECIFIED.) ;
#1812=B_SPLINE_SURFACE_WITH_KNOTS('',3,1,((#76174,#76175),(#76176,#76177),
(#76178,#76179),(#76180,#76181)),.UNSPECIFIED.,.F.,.F.,.F.,(4,4),(2,2),
(-0.471465822587465,-0.0968327577708928),(0.,1.50198816647678),
 .UNSPECIFIED.) ;
#1813=B_SPLINE_SURFACE_WITH_KNOTS('',3,1,((#76188,#76189),(#76190,#76191),
(#76192,#76193),(#76194,#76195)),.UNSPECIFIED.,.F.,.F.,.F.,(4,4),(2,2),
(0.,1.),(0.,0.8112),.UNSPECIFIED.) ;
#1814=B_SPLINE_SURFACE_WITH_KNOTS('',3,3,((#76253,#76254,#76255,#76256),
(#76257,#76258,#76259,#76260),(#76261,#76262,#76263,#76264),(#76265,#76266,
#76267,#76268),(#76269,#76270,#76271,#76272)),.UNSPECIFIED.,.F.,.F.,.F.,
(4,1,4),(4,4),(0.,0.571428571428571,1.),(0.,0.12989230765349),
 .UNSPECIFIED.) ;
#1815=B_SPLINE_SURFACE_WITH_KNOTS('',3,3,((#76276,#76277,#76278,#76279),
(#76280,#76281,#76282,#76283),(#76284,#76285,#76286,#76287),(#76288,#76289,
#76290,#76291),(#76292,#76293,#76294,#76295)),.UNSPECIFIED.,.F.,.F.,.F.,
(4,1,4),(4,4),(0.,0.571428571428571,1.),(0.,0.233629810933348),
 .UNSPECIFIED.) ;
#1816=B_SPLINE_SURFACE_WITH_KNOTS('',3,3,((#76299,#76300,#76301,#76302),
(#76303,#76304,#76305,#76306),(#76307,#76308,#76309,#76310),(#76311,#76312,
#76313,#76314),(#76315,#76316,#76317,#76318)),.UNSPECIFIED.,.F.,.F.,.F.,
(4,1,4),(4,4),(0.,0.571428571428571,1.),(0.,0.27640612106161),
 .UNSPECIFIED.) ;
#1817=B_SPLINE_SURFACE_WITH_KNOTS('',3,3,((#76322,#76323,#76324,#76325,
#76326),(#76327,#76328,#76329,#76330,#76331),(#76332,#76333,#76334,#76335,
#76336),(#76337,#76338,#76339,#76340,#76341),(#76342,#76343,#76344,#76345,
#76346)),.UNSPECIFIED.,.F.,.F.,.F.,(4,1,4),(4,1,4),(0.,0.571428571428571,
1.),(0.,0.510997712795854,1.19232799652366),.UNSPECIFIED.) ;
#1818=B_SPLINE_SURFACE_WITH_KNOTS('',3,3,((#76358,#76359,#76360,#76361,
#76362),(#76363,#76364,#76365,#76366,#76367),(#76368,#76369,#76370,#76371,
#76372),(#76373,#76374,#76375,#76376,#76377),(#76378,#76379,#76380,#76381,
#76382)),.UNSPECIFIED.,.F.,.F.,.F.,(4,1,4),(4,1,4),(0.,0.571428571428571,
1.),(0.,0.653796509940758,1.52552518986177),.UNSPECIFIED.) ;
#1819=B_SPLINE_SURFACE_WITH_KNOTS('',3,3,((#76395,#76396,#76397,#76398,
#76399,#76400,#76401),(#76402,#76403,#76404,#76405,#76406,#76407,#76408),
(#76409,#76410,#76411,#76412,#76413,#76414,#76415),(#76416,#76417,#76418,
#76419,#76420,#76421,#76422),(#76423,#76424,#76425,#76426,#76427,#76428,
#76429)),.UNSPECIFIED.,.F.,.F.,.F.,(4,1,4),(4,1,1,1,4),(0.,0.571428571428571,
1.),(3.75975382637766E-15,0.0255939875922149,0.051187975184426,0.0639849689805315,
0.0895789565727426),.UNSPECIFIED.) ;
#1820=B_SPLINE_SURFACE_WITH_KNOTS('',3,3,((#76443,#76444,#76445,#76446),
(#76447,#76448,#76449,#76450),(#76451,#76452,#76453,#76454),(#76455,#76456,
#76457,#76458),(#76459,#76460,#76461,#76462)),.UNSPECIFIED.,.F.,.F.,.F.,
(4,1,4),(4,4),(0.,0.571428571428571,1.),(0.,0.0677899888308747),
 .UNSPECIFIED.) ;
#1821=B_SPLINE_SURFACE_WITH_KNOTS('',3,3,((#76466,#76467,#76468,#76469,
#76470),(#76471,#76472,#76473,#76474,#76475),(#76476,#76477,#76478,#76479,
#76480),(#76481,#76482,#76483,#76484,#76485),(#76486,#76487,#76488,#76489,
#76490)),.UNSPECIFIED.,.F.,.F.,.F.,(4,1,4),(4,1,4),(0.,0.571428571428571,
1.),(0.,0.667475134411416,1.5574419802933),.UNSPECIFIED.) ;
#1822=B_SPLINE_SURFACE_WITH_KNOTS('',3,3,((#76503,#76504,#76505,#76506),
(#76507,#76508,#76509,#76510),(#76511,#76512,#76513,#76514),(#76515,#76516,
#76517,#76518),(#76519,#76520,#76521,#76522)),.UNSPECIFIED.,.F.,.F.,.F.,
(4,1,4),(4,4),(0.,0.571428571428571,1.),(0.,0.175732724220852),
 .UNSPECIFIED.) ;
#1823=B_SPLINE_SURFACE_WITH_KNOTS('',3,3,((#76526,#76527,#76528,#76529),
(#76530,#76531,#76532,#76533),(#76534,#76535,#76536,#76537),(#76538,#76539,
#76540,#76541),(#76542,#76543,#76544,#76545)),.UNSPECIFIED.,.F.,.F.,.F.,
(4,1,4),(4,4),(0.,0.571428571428571,1.),(0.,1.13812857775824),
 .UNSPECIFIED.) ;
#1824=B_SPLINE_SURFACE_WITH_KNOTS('',3,3,((#76549,#76550,#76551,#76552),
(#76553,#76554,#76555,#76556),(#76557,#76558,#76559,#76560),(#76561,#76562,
#76563,#76564),(#76565,#76566,#76567,#76568)),.UNSPECIFIED.,.F.,.F.,.F.,
(4,1,4),(4,4),(0.,0.571428571428571,1.),(0.,0.157312634644266),
 .UNSPECIFIED.) ;
#1825=B_SPLINE_SURFACE_WITH_KNOTS('',3,3,((#76572,#76573,#76574,#76575),
(#76576,#76577,#76578,#76579),(#76580,#76581,#76582,#76583),(#76584,#76585,
#76586,#76587),(#76588,#76589,#76590,#76591)),.UNSPECIFIED.,.F.,.F.,.F.,
(4,1,4),(4,4),(0.,0.571428571428571,1.),(0.,0.0204003555763695),
 .UNSPECIFIED.) ;
#1826=B_SPLINE_SURFACE_WITH_KNOTS('',3,3,((#76595,#76596,#76597,#76598),
(#76599,#76600,#76601,#76602),(#76603,#76604,#76605,#76606),(#76607,#76608,
#76609,#76610),(#76611,#76612,#76613,#76614)),.UNSPECIFIED.,.F.,.F.,.F.,
(4,1,4),(4,4),(0.,0.571428571428571,1.),(1.90971081540989E-15,0.17464806736394),
 .UNSPECIFIED.) ;
#1827=B_SPLINE_SURFACE_WITH_KNOTS('',5,1,((#76652,#76653),(#76654,#76655),
(#76656,#76657),(#76658,#76659),(#76660,#76661),(#76662,#76663),(#76664,
#76665),(#76666,#76667),(#76668,#76669),(#76670,#76671)),.UNSPECIFIED.,
 .F.,.F.,.F.,(6,1,1,1,1,6),(2,2),(0.504846387196225,0.6,0.7,0.8,0.9,1.),
(0.,1.5),.UNSPECIFIED.) ;
#1828=B_SPLINE_SURFACE_WITH_KNOTS('',5,1,((#76685,#76686),(#76687,#76688),
(#76689,#76690),(#76691,#76692),(#76693,#76694),(#76695,#76696),(#76697,
#76698),(#76699,#76700),(#76701,#76702),(#76703,#76704)),.UNSPECIFIED.,
 .F.,.F.,.F.,(6,1,1,1,1,6),(2,2),(0.0836762789821565,0.1,0.2,0.3,0.4,0.447897819536537),
(0.,1.5),.UNSPECIFIED.) ;
#1829=B_SPLINE_SURFACE_WITH_KNOTS('',5,1,((#76708,#76709),(#76710,#76711),
(#76712,#76713),(#76714,#76715),(#76716,#76717),(#76718,#76719)),
 .UNSPECIFIED.,.F.,.F.,.F.,(6,6),(2,2),(0.0348574618790549,0.0836762789809161),
(0.,1.5),.UNSPECIFIED.) ;
#1830=B_SPLINE_SURFACE_WITH_KNOTS('',5,1,((#76728,#76729),(#76730,#76731),
(#76732,#76733),(#76734,#76735),(#76736,#76737),(#76738,#76739),(#76740,
#76741),(#76742,#76743),(#76744,#76745),(#76746,#76747),(#76748,#76749),
(#76750,#76751),(#76752,#76753),(#76754,#76755),(#76756,#76757)),
 .UNSPECIFIED.,.F.,.F.,.F.,(6,1,1,1,1,1,1,1,1,1,6),(2,2),(0.,0.1,0.2,0.3,
0.4,0.5,0.6,0.7,0.8,0.9,1.),(0.,0.83184),.UNSPECIFIED.) ;
#1831=B_SPLINE_SURFACE_WITH_KNOTS('',3,1,((#76761,#76762),(#76763,#76764),
(#76765,#76766),(#76767,#76768)),.UNSPECIFIED.,.F.,.F.,.F.,(4,4),(2,2),
(0.,1.),(0.,0.7656),.UNSPECIFIED.) ;
#1832=B_SPLINE_SURFACE_WITH_KNOTS('',3,3,((#76825,#76826,#76827,#76828,
#76829),(#76830,#76831,#76832,#76833,#76834),(#76835,#76836,#76837,#76838,
#76839),(#76840,#76841,#76842,#76843,#76844),(#76845,#76846,#76847,#76848,
#76849)),.UNSPECIFIED.,.F.,.F.,.F.,(4,1,4),(4,1,4),(0.,0.571428571428571,
1.),(0.,0.0130357960000373,0.0304168573334205),.UNSPECIFIED.) ;
#1833=B_SPLINE_SURFACE_WITH_KNOTS('',3,1,((#76866,#76867),(#76868,#76869),
(#76870,#76871),(#76872,#76873),(#76874,#76875)),.UNSPECIFIED.,.F.,.F.,
 .F.,(4,1,4),(2,2),(0.,0.571428571428571,1.),(0.,0.451200000000012),
 .UNSPECIFIED.) ;
#1834=B_SPLINE_SURFACE_WITH_KNOTS('',3,3,((#76878,#76879,#76880,#76881,
#76882,#76883,#76884),(#76885,#76886,#76887,#76888,#76889,#76890,#76891),
(#76892,#76893,#76894,#76895,#76896,#76897,#76898),(#76899,#76900,#76901,
#76902,#76903,#76904,#76905),(#76906,#76907,#76908,#76909,#76910,#76911,
#76912)),.UNSPECIFIED.,.F.,.F.,.F.,(4,1,4),(4,1,1,1,4),(0.,0.571428571428571,
1.),(1.83791533766654E-16,0.00910869280420873,0.0212536165431535,0.030362309347362,
0.0425072330863067),.UNSPECIFIED.) ;
#1835=B_SPLINE_SURFACE_WITH_KNOTS('',3,1,((#76932,#76933),(#76934,#76935),
(#76936,#76937),(#76938,#76939),(#76940,#76941),(#76942,#76943)),
 .UNSPECIFIED.,.F.,.F.,.F.,(4,1,1,4),(2,2),(0.,0.285714285714286,0.571428571428571,
1.),(0.,0.4512),.UNSPECIFIED.) ;
#1836=B_SPLINE_SURFACE_WITH_KNOTS('',3,3,((#76946,#76947,#76948,#76949),
(#76950,#76951,#76952,#76953),(#76954,#76955,#76956,#76957),(#76958,#76959,
#76960,#76961),(#76962,#76963,#76964,#76965)),.UNSPECIFIED.,.F.,.F.,.F.,
(4,1,4),(4,4),(0.,0.571428571428571,1.),(-6.93889390390723E-18,0.369059935722116),
 .UNSPECIFIED.) ;
#1837=B_SPLINE_SURFACE_WITH_KNOTS('',3,3,((#76974,#76975,#76976,#76977),
(#76978,#76979,#76980,#76981),(#76982,#76983,#76984,#76985),(#76986,#76987,
#76988,#76989),(#76990,#76991,#76992,#76993)),.UNSPECIFIED.,.F.,.F.,.F.,
(4,1,4),(4,4),(0.,0.571428571428571,1.),(0.,0.228081359096226),
 .UNSPECIFIED.) ;
#1838=B_SPLINE_SURFACE_WITH_KNOTS('',3,3,((#77001,#77002,#77003,#77004,
#77005,#77006,#77007),(#77008,#77009,#77010,#77011,#77012,#77013,#77014),
(#77015,#77016,#77017,#77018,#77019,#77020,#77021),(#77022,#77023,#77024,
#77025,#77026,#77027,#77028),(#77029,#77030,#77031,#77032,#77033,#77034,
#77035)),.UNSPECIFIED.,.F.,.F.,.F.,(4,1,4),(4,3,4),(0.,0.571428571428571,
1.),(-0.011519137396051,0.,0.0257669909600073),.UNSPECIFIED.) ;
#1839=B_SPLINE_SURFACE_WITH_KNOTS('',3,3,((#77054,#77055,#77056,#77057),
(#77058,#77059,#77060,#77061),(#77062,#77063,#77064,#77065),(#77066,#77067,
#77068,#77069),(#77070,#77071,#77072,#77073)),.UNSPECIFIED.,.F.,.F.,.F.,
(4,1,4),(4,4),(0.,0.571428571428571,1.),(0.,0.366454031313985),
 .UNSPECIFIED.) ;
#1840=B_SPLINE_SURFACE_WITH_KNOTS('',3,3,((#77077,#77078,#77079,#77080),
(#77081,#77082,#77083,#77084),(#77085,#77086,#77087,#77088),(#77089,#77090,
#77091,#77092),(#77093,#77094,#77095,#77096)),.UNSPECIFIED.,.F.,.F.,.F.,
(4,1,4),(4,4),(0.,0.571428571428571,1.),(0.,0.226379744484658),
 .UNSPECIFIED.) ;
#1841=B_SPLINE_SURFACE_WITH_KNOTS('',3,3,((#77098,#77099,#77100,#77101),
(#77102,#77103,#77104,#77105),(#77106,#77107,#77108,#77109),(#77110,#77111,
#77112,#77113),(#77114,#77115,#77116,#77117)),.UNSPECIFIED.,.F.,.F.,.F.,
(4,1,4),(4,4),(0.,0.571428571428571,1.),(0.00879814959602052,0.042272992561856),
 .UNSPECIFIED.) ;
#1842=B_SPLINE_SURFACE_WITH_KNOTS('',3,3,((#77123,#77124,#77125,#77126),
(#77127,#77128,#77129,#77130),(#77131,#77132,#77133,#77134),(#77135,#77136,
#77137,#77138),(#77139,#77140,#77141,#77142)),.UNSPECIFIED.,.F.,.F.,.F.,
(4,1,4),(4,4),(0.,0.571428571428571,1.),(2.80806131699996E-14,0.177284657271612),
 .UNSPECIFIED.) ;
#1843=B_SPLINE_SURFACE_WITH_KNOTS('',3,3,((#77165,#77166,#77167,#77168),
(#77169,#77170,#77171,#77172),(#77173,#77174,#77175,#77176),(#77177,#77178,
#77179,#77180),(#77181,#77182,#77183,#77184)),.UNSPECIFIED.,.F.,.F.,.F.,
(4,1,4),(4,4),(0.,0.571428571428571,1.),(0.0088422414876098,0.0424839045660454),
 .UNSPECIFIED.) ;
#1844=B_SPLINE_SURFACE_WITH_KNOTS('',3,3,((#77188,#77189,#77190,#77191),
(#77192,#77193,#77194,#77195),(#77196,#77197,#77198,#77199),(#77200,#77201,
#77202,#77203),(#77204,#77205,#77206,#77207)),.UNSPECIFIED.,.F.,.F.,.F.,
(4,1,4),(4,4),(0.,0.571428571428571,1.),(0.,0.182076134495141),
 .UNSPECIFIED.) ;
#1845=B_SPLINE_SURFACE_WITH_KNOTS('',3,3,((#77213,#77214,#77215,#77216),
(#77217,#77218,#77219,#77220),(#77221,#77222,#77223,#77224),(#77225,#77226,
#77227,#77228),(#77229,#77230,#77231,#77232)),.UNSPECIFIED.,.F.,.F.,.F.,
(4,1,4),(4,4),(0.,0.571428571428571,1.),(0.,0.0102916147937805),
 .UNSPECIFIED.) ;
#1846=B_SPLINE_SURFACE_WITH_KNOTS('',3,1,((#77253,#77254),(#77255,#77256),
(#77257,#77258),(#77259,#77260)),.UNSPECIFIED.,.F.,.F.,.F.,(4,4),(2,2),
(0.120318448480489,0.194542293717003),(0.,0.78),.UNSPECIFIED.) ;
#1847=B_SPLINE_SURFACE_WITH_KNOTS('',3,1,((#77262,#77263),(#77264,#77265),
(#77266,#77267),(#77268,#77269)),.UNSPECIFIED.,.F.,.F.,.F.,(4,4),(2,2),
(0.00785988716405027,0.120318448346505),(0.,0.78),.UNSPECIFIED.) ;
#1848=B_SPLINE_SURFACE_WITH_KNOTS('',3,3,((#77278,#77279,#77280,#77281,
#77282),(#77283,#77284,#77285,#77286,#77287),(#77288,#77289,#77290,#77291,
#77292),(#77293,#77294,#77295,#77296,#77297),(#77298,#77299,#77300,#77301,
#77302)),.UNSPECIFIED.,.F.,.F.,.F.,(4,1,4),(4,1,4),(0.,0.571428571428571,
1.),(0.,0.017271853441312,0.0345437068826239),.UNSPECIFIED.) ;
#1849=B_SPLINE_SURFACE_WITH_KNOTS('',3,3,((#77312,#77313,#77314,#77315),
(#77316,#77317,#77318,#77319),(#77320,#77321,#77322,#77323),(#77324,#77325,
#77326,#77327),(#77328,#77329,#77330,#77331)),.UNSPECIFIED.,.F.,.F.,.F.,
(4,1,4),(4,4),(0.,0.571428571428571,1.),(0.,1.07230437897721),
 .UNSPECIFIED.) ;
#1850=B_SPLINE_SURFACE_WITH_KNOTS('',3,3,((#77335,#77336,#77337,#77338),
(#77339,#77340,#77341,#77342),(#77343,#77344,#77345,#77346),(#77347,#77348,
#77349,#77350),(#77351,#77352,#77353,#77354)),.UNSPECIFIED.,.F.,.F.,.F.,
(4,1,4),(4,4),(0.,0.571428571428571,1.),(0.,0.0184851761370125),
 .UNSPECIFIED.) ;
#1851=B_SPLINE_SURFACE_WITH_KNOTS('',3,3,((#77362,#77363,#77364,#77365,
#77366,#77367),(#77368,#77369,#77370,#77371,#77372,#77373),(#77374,#77375,
#77376,#77377,#77378,#77379),(#77380,#77381,#77382,#77383,#77384,#77385),
(#77386,#77387,#77388,#77389,#77390,#77391)),.UNSPECIFIED.,.F.,.F.,.F.,
(4,1,4),(4,1,1,4),(0.,0.571428571428571,1.),(0.,0.0158024732980411,0.0263374554967351,
0.0368724376954292),.UNSPECIFIED.) ;
#1852=B_SPLINE_SURFACE_WITH_KNOTS('',3,3,((#77407,#77408,#77409,#77410),
(#77411,#77412,#77413,#77414),(#77415,#77416,#77417,#77418),(#77419,#77420,
#77421,#77422),(#77423,#77424,#77425,#77426)),.UNSPECIFIED.,.F.,.F.,.F.,
(4,1,4),(4,4),(0.,0.571428571428571,1.),(0.,0.971129055990219),
 .UNSPECIFIED.) ;
#1853=B_SPLINE_SURFACE_WITH_KNOTS('',3,3,((#77435,#77436,#77437,#77438,
#77439),(#77440,#77441,#77442,#77443,#77444),(#77445,#77446,#77447,#77448,
#77449),(#77450,#77451,#77452,#77453,#77454),(#77455,#77456,#77457,#77458,
#77459)),.UNSPECIFIED.,.F.,.F.,.F.,(4,1,4),(4,1,4),(0.,0.571428571428571,
1.),(0.,0.0100922291021495,0.0235485345716821),.UNSPECIFIED.) ;
#1854=B_SPLINE_SURFACE_WITH_KNOTS('',3,3,((#77477,#77478,#77479,#77480,
#77481,#77482),(#77483,#77484,#77485,#77486,#77487,#77488),(#77489,#77490,
#77491,#77492,#77493,#77494),(#77495,#77496,#77497,#77498,#77499,#77500),
(#77501,#77502,#77503,#77504,#77505,#77506)),.UNSPECIFIED.,.F.,.F.,.F.,
(4,1,4),(4,1,1,4),(0.,0.571428571428571,1.),(0.,0.0112795268235383,0.0225590536470765,
0.0394783438823839),.UNSPECIFIED.) ;
#1855=B_SPLINE_SURFACE_WITH_KNOTS('',3,3,((#77525,#77526,#77527,#77528),
(#77529,#77530,#77531,#77532),(#77533,#77534,#77535,#77536),(#77537,#77538,
#77539,#77540),(#77541,#77542,#77543,#77544)),.UNSPECIFIED.,.F.,.F.,.F.,
(4,1,4),(4,4),(0.,0.571428571428571,1.),(0.,1.34425818567182),
 .UNSPECIFIED.) ;
#1856=B_SPLINE_SURFACE_WITH_KNOTS('',3,3,((#77555,#77556,#77557,#77558),
(#77559,#77560,#77561,#77562),(#77563,#77564,#77565,#77566),(#77567,#77568,
#77569,#77570),(#77571,#77572,#77573,#77574)),.UNSPECIFIED.,.F.,.F.,.F.,
(4,1,4),(4,4),(0.,0.571428571428571,1.),(0.,0.0557418591005873),
 .UNSPECIFIED.) ;
#1857=B_SPLINE_SURFACE_WITH_KNOTS('',3,3,((#77582,#77583,#77584,#77585,
#77586,#77587,#77588),(#77589,#77590,#77591,#77592,#77593,#77594,#77595),
(#77596,#77597,#77598,#77599,#77600,#77601,#77602),(#77603,#77604,#77605,
#77606,#77607,#77608,#77609),(#77610,#77611,#77612,#77613,#77614,#77615,
#77616)),.UNSPECIFIED.,.F.,.F.,.F.,(4,1,4),(4,1,1,1,4),(0.,0.571428571428571,
1.),(0.,0.0119712276176857,0.0239424552353715,0.0359136828530572,0.0418992966619001),
 .UNSPECIFIED.) ;
#1858=B_SPLINE_SURFACE_WITH_KNOTS('',3,3,((#77626,#77627,#77628,#77629),
(#77630,#77631,#77632,#77633),(#77634,#77635,#77636,#77637),(#77638,#77639,
#77640,#77641),(#77642,#77643,#77644,#77645)),.UNSPECIFIED.,.F.,.F.,.F.,
(4,1,4),(4,4),(0.,0.571428571428571,1.),(0.,1.19778613661182),
 .UNSPECIFIED.) ;
#1859=B_SPLINE_SURFACE_WITH_KNOTS('',3,3,((#77652,#77653,#77654,#77655),
(#77656,#77657,#77658,#77659),(#77660,#77661,#77662,#77663),(#77664,#77665,
#77666,#77667),(#77668,#77669,#77670,#77671)),.UNSPECIFIED.,.F.,.F.,.F.,
(4,1,4),(4,4),(0.,0.571428571428571,1.),(0.,0.0185272595354357),
 .UNSPECIFIED.) ;
#1860=B_SPLINE_SURFACE_WITH_KNOTS('',3,1,((#77680,#77681),(#77682,#77683),
(#77684,#77685),(#77686,#77687),(#77688,#77689),(#77690,#77691),(#77692,
#77693)),.UNSPECIFIED.,.F.,.F.,.F.,(4,3,4),(2,2),(-0.988543128598371,-0.545479769376514,
-0.531340881080732),(0.,1.50198816647678),.UNSPECIFIED.) ;
#1861=B_SPLINE_SURFACE_WITH_KNOTS('',3,1,((#77695,#77696),(#77697,#77698),
(#77699,#77700),(#77701,#77702),(#77703,#77704),(#77705,#77706)),
 .UNSPECIFIED.,.F.,.F.,.F.,(4,1,1,4),(2,2),(0.,0.285714285714286,0.571428571428571,
1.),(0.,0.8112),.UNSPECIFIED.) ;
#1862=B_SPLINE_SURFACE_WITH_KNOTS('',3,3,((#77716,#77717,#77718,#77719,
#77720),(#77721,#77722,#77723,#77724,#77725),(#77726,#77727,#77728,#77729,
#77730),(#77731,#77732,#77733,#77734,#77735),(#77736,#77737,#77738,#77739,
#77740)),.UNSPECIFIED.,.F.,.F.,.F.,(4,1,4),(4,1,4),(0.,0.571428571428571,
1.),(0.,0.0106131136334063,0.0247639318112814),.UNSPECIFIED.) ;
#1863=B_SPLINE_SURFACE_WITH_KNOTS('',3,1,((#77753,#77754),(#77755,#77756),
(#77757,#77758),(#77759,#77760)),.UNSPECIFIED.,.F.,.F.,.F.,(4,4),(2,2),
(0.,1.),(0.,0.1512),.UNSPECIFIED.) ;
#1864=B_SPLINE_SURFACE_WITH_KNOTS('',3,3,((#77777,#77778,#77779,#77780),
(#77781,#77782,#77783,#77784),(#77785,#77786,#77787,#77788),(#77789,#77790,
#77791,#77792),(#77793,#77794,#77795,#77796)),.UNSPECIFIED.,.F.,.F.,.F.,
(4,1,4),(4,4),(0.,0.571428571428571,1.),(0.0229372865431325,1.40205259514116),
 .UNSPECIFIED.) ;
#1865=B_SPLINE_SURFACE_WITH_KNOTS('',3,3,((#77811,#77812,#77813,#77814),
(#77815,#77816,#77817,#77818),(#77819,#77820,#77821,#77822),(#77823,#77824,
#77825,#77826),(#77827,#77828,#77829,#77830)),.UNSPECIFIED.,.F.,.F.,.F.,
(4,1,4),(4,4),(0.,0.571428571428571,1.),(0.,0.0557418591005868),
 .UNSPECIFIED.) ;
#1866=B_SPLINE_SURFACE_WITH_KNOTS('',3,3,((#77842,#77843,#77844,#77845,
#77846,#77847,#77848),(#77849,#77850,#77851,#77852,#77853,#77854,#77855),
(#77856,#77857,#77858,#77859,#77860,#77861,#77862),(#77863,#77864,#77865,
#77866,#77867,#77868,#77869),(#77870,#77871,#77872,#77873,#77874,#77875,
#77876)),.UNSPECIFIED.,.F.,.F.,.F.,(4,1,4),(4,1,1,1,4),(0.,0.571428571428571,
1.),(0.,0.00598561380884316,0.0179568414265295,0.0299280690442158,0.0418992966619021),
 .UNSPECIFIED.) ;
#1867=B_SPLINE_SURFACE_WITH_KNOTS('',3,3,((#77894,#77895,#77896,#77897),
(#77898,#77899,#77900,#77901),(#77902,#77903,#77904,#77905),(#77906,#77907,
#77908,#77909),(#77910,#77911,#77912,#77913)),.UNSPECIFIED.,.F.,.F.,.F.,
(4,1,4),(4,4),(0.,0.571428571428571,1.),(0.,1.20789221798527),
 .UNSPECIFIED.) ;
#1868=B_SPLINE_SURFACE_WITH_KNOTS('',3,3,((#77922,#77923,#77924,#77925,
#77926,#77927,#77928),(#77929,#77930,#77931,#77932,#77933,#77934,#77935),
(#77936,#77937,#77938,#77939,#77940,#77941,#77942),(#77943,#77944,#77945,
#77946,#77947,#77948,#77949),(#77950,#77951,#77952,#77953,#77954,#77955,
#77956)),.UNSPECIFIED.,.F.,.F.,.F.,(4,1,4),(4,1,1,1,4),(0.,0.571428571428571,
1.),(0.,0.0149660193069295,0.0224490289603943,0.0374150482673238,0.0523810675742533),
 .UNSPECIFIED.) ;
#1869=B_SPLINE_SURFACE_WITH_KNOTS('',3,1,((#77984,#77985),(#77986,#77987),
(#77988,#77989),(#77990,#77991),(#77992,#77993),(#77994,#77995),(#77996,
#77997)),.UNSPECIFIED.,.F.,.F.,.F.,(4,1,1,1,4),(2,2),(0.,0.285714285714286,
0.5,0.785714285714286,1.),(0.,0.1512),.UNSPECIFIED.) ;
#1870=B_SPLINE_SURFACE_WITH_KNOTS('',3,3,((#78000,#78001,#78002,#78003),
(#78004,#78005,#78006,#78007),(#78008,#78009,#78010,#78011),(#78012,#78013,
#78014,#78015),(#78016,#78017,#78018,#78019)),.UNSPECIFIED.,.F.,.F.,.F.,
(4,1,4),(4,4),(0.,0.571428571428571,1.),(0.0231068825027873,1.41003451675495),
 .UNSPECIFIED.) ;
#1871=B_SPLINE_SURFACE_WITH_KNOTS('',3,3,((#78031,#78032,#78033,#78034),
(#78035,#78036,#78037,#78038),(#78039,#78040,#78041,#78042),(#78043,#78044,
#78045,#78046),(#78047,#78048,#78049,#78050)),.UNSPECIFIED.,.F.,.F.,.F.,
(4,1,4),(4,4),(0.,0.571428571428571,1.),(0.,0.0709441843098284),
 .UNSPECIFIED.) ;
#1872=B_SPLINE_SURFACE_WITH_KNOTS('',3,3,((#78062,#78063,#78064,#78065,
#78066,#78067),(#78068,#78069,#78070,#78071,#78072,#78073),(#78074,#78075,
#78076,#78077,#78078,#78079),(#78080,#78081,#78082,#78083,#78084,#78085),
(#78086,#78087,#78088,#78089,#78090,#78091)),.UNSPECIFIED.,.F.,.F.,.F.,
(4,1,4),(4,1,1,4),(0.,0.571428571428571,1.),(0.,0.0418992966619,0.0698321611031666,
0.0977650255444333),.UNSPECIFIED.) ;
#1873=B_SPLINE_SURFACE_WITH_KNOTS('',3,3,((#78107,#78108,#78109,#78110),
(#78111,#78112,#78113,#78114),(#78115,#78116,#78117,#78118),(#78119,#78120,
#78121,#78122),(#78123,#78124,#78125,#78126)),.UNSPECIFIED.,.F.,.F.,.F.,
(4,1,4),(4,4),(0.,0.571428571428571,1.),(0.,1.20265740584169),
 .UNSPECIFIED.) ;
#1874=B_SPLINE_SURFACE_WITH_KNOTS('',3,1,((#78138,#78139),(#78140,#78141),
(#78142,#78143),(#78144,#78145),(#78146,#78147),(#78148,#78149),(#78150,
#78151)),.UNSPECIFIED.,.F.,.F.,.F.,(4,1,1,1,4),(2,2),(0.,0.285714285714286,
0.571428571428571,0.857142857142857,1.),(0.,0.1512),.UNSPECIFIED.) ;
#1875=B_SPLINE_SURFACE_WITH_KNOTS('',3,1,((#78154,#78155),(#78156,#78157),
(#78158,#78159),(#78160,#78161),(#78162,#78163),(#78164,#78165),(#78166,
#78167)),.UNSPECIFIED.,.F.,.F.,.F.,(4,3,4),(2,2),(-0.988543128598371,-0.545479769376514,
-0.531340881080732),(0.,1.50198816647678),.UNSPECIFIED.) ;
#1876=B_SPLINE_SURFACE_WITH_KNOTS('',3,1,((#78171,#78172),(#78173,#78174),
(#78175,#78176),(#78177,#78178)),.UNSPECIFIED.,.F.,.F.,.F.,(4,4),(2,2),
(0.,1.),(0.,0.1512),.UNSPECIFIED.) ;
#1877=B_SPLINE_SURFACE_WITH_KNOTS('',3,3,((#78268,#78269,#78270,#78271,
#78272,#78273,#78274),(#78275,#78276,#78277,#78278,#78279,#78280,#78281),
(#78282,#78283,#78284,#78285,#78286,#78287,#78288),(#78289,#78290,#78291,
#78292,#78293,#78294,#78295),(#78296,#78297,#78298,#78299,#78300,#78301,
#78302)),.UNSPECIFIED.,.F.,.F.,.F.,(4,1,4),(4,1,1,1,4),(0.,0.571428571428571,
1.),(0.,0.0141037612586181,0.0211556418879271,0.0352594031465452,0.0493631644051633),
 .UNSPECIFIED.) ;
#1878=B_SPLINE_SURFACE_WITH_KNOTS('',3,1,((#78321,#78322),(#78323,#78324),
(#78325,#78326),(#78327,#78328),(#78329,#78330),(#78331,#78332),(#78333,
#78334)),.UNSPECIFIED.,.F.,.F.,.F.,(4,1,1,1,4),(2,2),(0.,0.285714285714286,
0.5,0.785714285714286,1.),(0.,0.1512),.UNSPECIFIED.) ;
#1879=B_SPLINE_SURFACE_WITH_KNOTS('',3,3,((#78337,#78338,#78339,#78340,
#78341),(#78342,#78343,#78344,#78345,#78346),(#78347,#78348,#78349,#78350,
#78351),(#78352,#78353,#78354,#78355,#78356),(#78357,#78358,#78359,#78360,
#78361)),.UNSPECIFIED.,.F.,.F.,.F.,(4,1,4),(4,1,4),(0.,0.571428571428571,
1.),(0.,0.0105301970552765,0.0245704597956453),.UNSPECIFIED.) ;
#1880=B_SPLINE_SURFACE_WITH_KNOTS('',3,3,((#78367,#78368,#78369,#78370,
#78371),(#78372,#78373,#78374,#78375,#78376),(#78377,#78378,#78379,#78380,
#78381),(#78382,#78383,#78384,#78385,#78386),(#78387,#78388,#78389,#78390,
#78391)),.UNSPECIFIED.,.F.,.F.,.F.,(4,1,4),(4,1,4),(0.,0.571428571428571,
1.),(0.,0.0180035869295808,0.0315062771267664),.UNSPECIFIED.) ;
#1881=B_SPLINE_SURFACE_WITH_KNOTS('',3,1,((#78408,#78409),(#78410,#78411),
(#78412,#78413),(#78414,#78415)),.UNSPECIFIED.,.F.,.F.,.F.,(4,4),(2,2),
(0.,1.),(0.,0.1512),.UNSPECIFIED.) ;
#1882=B_SPLINE_SURFACE_WITH_KNOTS('',3,3,((#78425,#78426,#78427,#78428),
(#78429,#78430,#78431,#78432),(#78433,#78434,#78435,#78436),(#78437,#78438,
#78439,#78440),(#78441,#78442,#78443,#78444)),.UNSPECIFIED.,.F.,.F.,.F.,
(4,1,4),(4,4),(0.,0.571428571428571,1.),(0.020008660331873,1.03467847166523),
 .UNSPECIFIED.) ;
#1883=B_SPLINE_SURFACE_WITH_KNOTS('',3,3,((#78453,#78454,#78455,#78456,
#78457,#78458,#78459),(#78460,#78461,#78462,#78463,#78464,#78465,#78466),
(#78467,#78468,#78469,#78470,#78471,#78472,#78473),(#78474,#78475,#78476,
#78477,#78478,#78479,#78480),(#78481,#78482,#78483,#78484,#78485,#78486,
#78487)),.UNSPECIFIED.,.F.,.F.,.F.,(4,1,4),(4,1,1,1,4),(0.,0.571428571428571,
1.),(0.,0.00984040545418749,0.0229609460597708,0.0328013515139583,0.0459218921195416),
 .UNSPECIFIED.) ;
#1884=B_SPLINE_SURFACE_WITH_KNOTS('',3,1,((#78508,#78509),(#78510,#78511),
(#78512,#78513),(#78514,#78515),(#78516,#78517),(#78518,#78519),(#78520,
#78521)),.UNSPECIFIED.,.F.,.F.,.F.,(4,1,1,1,4),(2,2),(0.,0.285714285714286,
0.5,0.714285714285714,1.),(0.,0.1512),.UNSPECIFIED.) ;
#1885=B_SPLINE_SURFACE_WITH_KNOTS('',3,3,((#78527,#78528,#78529,#78530),
(#78531,#78532,#78533,#78534),(#78535,#78536,#78537,#78538),(#78539,#78540,
#78541,#78542),(#78543,#78544,#78545,#78546)),.UNSPECIFIED.,.F.,.F.,.F.,
(4,1,4),(4,4),(0.,0.571428571428571,1.),(0.0169663179244005,1.12511677037933),
 .UNSPECIFIED.) ;
#1886=B_SPLINE_SURFACE_WITH_KNOTS('',3,3,((#78552,#78553,#78554,#78555),
(#78556,#78557,#78558,#78559),(#78560,#78561,#78562,#78563),(#78564,#78565,
#78566,#78567),(#78568,#78569,#78570,#78571)),.UNSPECIFIED.,.F.,.F.,.F.,
(4,1,4),(4,4),(0.,0.571428571428571,1.),(0.0170557641123888,1.13243225761785),
 .UNSPECIFIED.) ;
#1887=B_SPLINE_SURFACE_WITH_KNOTS('',3,1,((#78575,#78576),(#78577,#78578),
(#78579,#78580),(#78581,#78582),(#78583,#78584)),.UNSPECIFIED.,.F.,.F.,
 .F.,(4,1,4),(2,2),(0.,0.571428571428571,1.),(0.,0.1512),.UNSPECIFIED.) ;
#1888=B_SPLINE_SURFACE_WITH_KNOTS('',3,3,((#78590,#78591,#78592,#78593),
(#78594,#78595,#78596,#78597),(#78598,#78599,#78600,#78601),(#78602,#78603,
#78604,#78605),(#78606,#78607,#78608,#78609)),.UNSPECIFIED.,.F.,.F.,.F.,
(4,1,4),(4,4),(0.,0.571428571428571,1.),(0.019875255616694,1.02674783308136),
 .UNSPECIFIED.) ;
#1889=B_SPLINE_SURFACE_WITH_KNOTS('',3,1,((#78616,#78617),(#78618,#78619),
(#78620,#78621),(#78622,#78623),(#78624,#78625),(#78626,#78627),(#78628,
#78629)),.UNSPECIFIED.,.F.,.F.,.F.,(4,3,4),(2,2),(0.241689284630679,0.500017400470172,
0.549213097360471),(0.,1.50203770750399),.UNSPECIFIED.) ;
#1890=B_SPLINE_SURFACE_WITH_KNOTS('',3,1,((#78632,#78633),(#78634,#78635),
(#78636,#78637),(#78638,#78639)),.UNSPECIFIED.,.F.,.F.,.F.,(4,4),(2,2),
(-0.471465822587465,-0.0968327577708928),(0.,1.50198816647678),
 .UNSPECIFIED.) ;
#1891=B_SPLINE_SURFACE_WITH_KNOTS('',3,3,((#78641,#78642,#78643,#78644,
#78645,#78646,#78647),(#78648,#78649,#78650,#78651,#78652,#78653,#78654),
(#78655,#78656,#78657,#78658,#78659,#78660,#78661),(#78662,#78663,#78664,
#78665,#78666,#78667,#78668),(#78669,#78670,#78671,#78672,#78673,#78674,
#78675)),.UNSPECIFIED.,.F.,.F.,.F.,(4,1,4),(4,3,4),(0.,0.571428571428571,
1.),(-0.00748019188171517,0.,0.129892307653464),.UNSPECIFIED.) ;
#1892=B_SPLINE_SURFACE_WITH_KNOTS('',3,3,((#78700,#78701,#78702,#78703),
(#78704,#78705,#78706,#78707),(#78708,#78709,#78710,#78711),(#78712,#78713,
#78714,#78715),(#78716,#78717,#78718,#78719)),.UNSPECIFIED.,.F.,.F.,.F.,
(4,1,4),(4,4),(0.,0.571428571428571,1.),(0.,0.233629810933348),
 .UNSPECIFIED.) ;
#1893=B_SPLINE_SURFACE_WITH_KNOTS('',5,1,((#78722,#78723),(#78724,#78725),
(#78726,#78727),(#78728,#78729),(#78730,#78731),(#78732,#78733),(#78734,
#78735)),.UNSPECIFIED.,.F.,.F.,.F.,(6,1,6),(2,2),(-0.202504416334417,-0.2,
-0.114745808067944),(0.,0.78),.UNSPECIFIED.) ;
#1894=B_SPLINE_SURFACE_WITH_KNOTS('',5,1,((#78738,#78739),(#78740,#78741),
(#78742,#78743),(#78744,#78745),(#78746,#78747),(#78748,#78749),(#78750,
#78751)),.UNSPECIFIED.,.F.,.F.,.F.,(6,1,6),(2,2),(-0.114745808067916,-0.1,
-0.040837741884948),(0.,0.78),.UNSPECIFIED.) ;
#1895=B_SPLINE_SURFACE_WITH_KNOTS('',5,1,((#78753,#78754),(#78755,#78756),
(#78757,#78758),(#78759,#78760),(#78761,#78762),(#78763,#78764)),
 .UNSPECIFIED.,.F.,.F.,.F.,(6,6),(2,2),(-0.0408377418849424,0.),(0.,0.78),
 .UNSPECIFIED.) ;
#1896=B_SPLINE_SURFACE_WITH_KNOTS('',3,1,((#78776,#78777),(#78778,#78779),
(#78780,#78781),(#78782,#78783),(#78784,#78785),(#78786,#78787)),
 .UNSPECIFIED.,.F.,.F.,.F.,(4,1,1,4),(2,2),(0.,0.5,0.714285714285714,1.),
(0.,0.6912),.UNSPECIFIED.) ;
#1897=B_SPLINE_SURFACE_WITH_KNOTS('',3,3,((#78788,#78789,#78790,#78791),
(#78792,#78793,#78794,#78795),(#78796,#78797,#78798,#78799),(#78800,#78801,
#78802,#78803),(#78804,#78805,#78806,#78807)),.UNSPECIFIED.,.F.,.F.,.F.,
(4,1,4),(4,4),(0.,0.571428571428571,1.),(0.,0.141072567236982),
 .UNSPECIFIED.) ;
#1898=B_SPLINE_SURFACE_WITH_KNOTS('',3,3,((#78809,#78810,#78811,#78812),
(#78813,#78814,#78815,#78816),(#78817,#78818,#78819,#78820),(#78821,#78822,
#78823,#78824),(#78825,#78826,#78827,#78828)),.UNSPECIFIED.,.F.,.F.,.F.,
(4,1,4),(4,4),(0.,0.571428571428571,1.),(0.,1.13812857775824),
 .UNSPECIFIED.) ;
#1899=B_SPLINE_SURFACE_WITH_KNOTS('',3,3,((#78830,#78831,#78832,#78833),
(#78834,#78835,#78836,#78837),(#78838,#78839,#78840,#78841),(#78842,#78843,
#78844,#78845),(#78846,#78847,#78848,#78849)),.UNSPECIFIED.,.F.,.F.,.F.,
(4,1,4),(4,4),(0.,0.571428571428571,1.),(0.,0.175732724220853),
 .UNSPECIFIED.) ;
#1900=B_SPLINE_SURFACE_WITH_KNOTS('',3,3,((#78851,#78852,#78853,#78854,
#78855),(#78856,#78857,#78858,#78859,#78860),(#78861,#78862,#78863,#78864,
#78865),(#78866,#78867,#78868,#78869,#78870),(#78871,#78872,#78873,#78874,
#78875)),.UNSPECIFIED.,.F.,.F.,.F.,(4,1,4),(4,1,4),(0.,0.571428571428571,
1.),(0.,0.66747373630185,1.55743871803765),.UNSPECIFIED.) ;
#1901=B_SPLINE_SURFACE_WITH_KNOTS('',3,3,((#78877,#78878,#78879,#78880),
(#78881,#78882,#78883,#78884),(#78885,#78886,#78887,#78888),(#78889,#78890,
#78891,#78892),(#78893,#78894,#78895,#78896)),.UNSPECIFIED.,.F.,.F.,.F.,
(4,1,4),(4,4),(0.,0.571428571428571,1.),(0.,0.0677899888308747),
 .UNSPECIFIED.) ;
#1902=B_SPLINE_SURFACE_WITH_KNOTS('',3,3,((#78904,#78905,#78906,#78907,
#78908,#78909,#78910),(#78911,#78912,#78913,#78914,#78915,#78916,#78917),
(#78918,#78919,#78920,#78921,#78922,#78923,#78924),(#78925,#78926,#78927,
#78928,#78929,#78930,#78931),(#78932,#78933,#78934,#78935,#78936,#78937,
#78938)),.UNSPECIFIED.,.F.,.F.,.F.,(4,1,4),(4,1,1,1,4),(0.,0.571428571428571,
1.),(0.,0.0255939875922127,0.038390981388319,0.0639849689805316,0.0895789565727443),
 .UNSPECIFIED.) ;
#1903=B_SPLINE_SURFACE_WITH_KNOTS('',3,3,((#78948,#78949,#78950,#78951,
#78952),(#78953,#78954,#78955,#78956,#78957),(#78958,#78959,#78960,#78961,
#78962),(#78963,#78964,#78965,#78966,#78967),(#78968,#78969,#78970,#78971,
#78972)),.UNSPECIFIED.,.F.,.F.,.F.,(4,1,4),(4,1,4),(0.,0.571428571428571,
1.),(0.,0.653796509940757,1.52552518986177),.UNSPECIFIED.) ;
#1904=B_SPLINE_SURFACE_WITH_KNOTS('',3,3,((#78985,#78986,#78987,#78988,
#78989),(#78990,#78991,#78992,#78993,#78994),(#78995,#78996,#78997,#78998,
#78999),(#79000,#79001,#79002,#79003,#79004),(#79005,#79006,#79007,#79008,
#79009)),.UNSPECIFIED.,.F.,.F.,.F.,(4,1,4),(4,1,4),(0.,0.571428571428571,
1.),(0.,0.500681763148267,1.16825744734596),.UNSPECIFIED.) ;
#1905=B_SPLINE_SURFACE_WITH_KNOTS('',3,3,((#79016,#79017,#79018,#79019,
#79020),(#79021,#79022,#79023,#79024,#79025),(#79026,#79027,#79028,#79029,
#79030),(#79031,#79032,#79033,#79034,#79035),(#79036,#79037,#79038,#79039,
#79040)),.UNSPECIFIED.,.F.,.F.,.F.,(4,1,4),(4,1,4),(0.,0.571428571428571,
1.),(0.,0.0104089910116412,0.0242876456938294),.UNSPECIFIED.) ;
#1906=B_SPLINE_SURFACE_WITH_KNOTS('',3,1,((#79046,#79047),(#79048,#79049),
(#79050,#79051),(#79052,#79053),(#79054,#79055),(#79056,#79057),(#79058,
#79059)),.UNSPECIFIED.,.F.,.F.,.F.,(4,1,1,1,4),(2,2),(0.,0.285714285714286,
0.571428571428571,0.857142857142857,1.),(0.,1.4712),.UNSPECIFIED.) ;
#1907=B_SPLINE_SURFACE_WITH_KNOTS('',5,1,((#79061,#79062),(#79063,#79064),
(#79065,#79066),(#79067,#79068),(#79069,#79070),(#79071,#79072),(#79073,
#79074),(#79075,#79076),(#79077,#79078),(#79079,#79080)),.UNSPECIFIED.,
 .F.,.F.,.F.,(6,1,1,1,1,6),(2,2),(-1.,-0.9,-0.8,-0.7,-0.6,-0.568009935219903),
(0.,1.5),.UNSPECIFIED.) ;
#1908=B_SPLINE_SURFACE_WITH_KNOTS('',5,1,((#79082,#79083),(#79084,#79085),
(#79086,#79087),(#79088,#79089),(#79090,#79091),(#79092,#79093),(#79094,
#79095),(#79096,#79097),(#79098,#79099)),.UNSPECIFIED.,.F.,.F.,.F.,(6,1,
1,1,6),(2,2),(-0.568009935219888,-0.5,-0.4,-0.3,-0.202504416334422),(0.,
1.5),.UNSPECIFIED.) ;
#1909=B_SPLINE_SURFACE_WITH_KNOTS('',3,1,((#79104,#79105),(#79106,#79107),
(#79108,#79109),(#79110,#79111)),.UNSPECIFIED.,.F.,.F.,.F.,(4,4),(2,2),
(-0.0465039596324731,-0.00333818885951975),(0.,0.78),.UNSPECIFIED.) ;
#1910=B_SPLINE_SURFACE_WITH_KNOTS('',3,1,((#79113,#79114),(#79115,#79116),
(#79117,#79118),(#79119,#79120)),.UNSPECIFIED.,.F.,.F.,.F.,(4,4),(2,2),
(0.,1.),(0.,0.4512),.UNSPECIFIED.) ;
#1911=B_SPLINE_SURFACE_WITH_KNOTS('',3,1,((#79122,#79123),(#79124,#79125),
(#79126,#79127),(#79128,#79129),(#79130,#79131)),.UNSPECIFIED.,.F.,.F.,
 .F.,(4,1,4),(2,2),(0.,0.571428571428571,1.),(0.,0.8112),.UNSPECIFIED.) ;
#1912=B_SPLINE_SURFACE_WITH_KNOTS('',3,1,((#79135,#79136),(#79137,#79138),
(#79139,#79140),(#79141,#79142),(#79143,#79144),(#79145,#79146)),
 .UNSPECIFIED.,.F.,.F.,.F.,(4,1,1,4),(2,2),(0.,0.285714285714286,0.571428571428571,
1.),(0.,0.8112),.UNSPECIFIED.) ;
#1913=B_SPLINE_SURFACE_WITH_KNOTS('',3,1,((#79148,#79149),(#79150,#79151),
(#79152,#79153),(#79154,#79155)),.UNSPECIFIED.,.F.,.F.,.F.,(4,4),(2,2),
(0.,1.),(0.,0.8112),.UNSPECIFIED.) ;
#1914=B_SPLINE_SURFACE_WITH_KNOTS('',3,1,((#79157,#79158),(#79159,#79160),
(#79161,#79162),(#79163,#79164)),.UNSPECIFIED.,.F.,.F.,.F.,(4,4),(2,2),
(0.,1.),(0.,1.4712),.UNSPECIFIED.) ;
#1915=B_SPLINE_SURFACE_WITH_KNOTS('',3,1,((#79165,#79166),(#79167,#79168),
(#79169,#79170),(#79171,#79172)),.UNSPECIFIED.,.F.,.F.,.F.,(4,4),(2,2),
(0.597473964327042,0.930240743465184),(0.,1.50203770750399),
 .UNSPECIFIED.) ;
#1916=B_SPLINE_SURFACE_WITH_KNOTS('',3,1,((#79174,#79175),(#79176,#79177),
(#79178,#79179),(#79180,#79181),(#79182,#79183),(#79184,#79185),(#79186,
#79187)),.UNSPECIFIED.,.F.,.F.,.F.,(4,3,4),(2,2),(0.241689284630679,0.500017400470172,
0.549213097360471),(0.,1.50203770750399),.UNSPECIFIED.) ;
#2167=SPHERICAL_SURFACE('',#49985,0.119999999999985) ;
#2168=SPHERICAL_SURFACE('',#49991,0.119999999999999) ;
#2169=SPHERICAL_SURFACE('',#50056,0.120000000000007) ;
#2170=SPHERICAL_SURFACE('',#50063,0.12) ;
#2171=SPHERICAL_SURFACE('',#50098,0.120000000000005) ;
#2172=SPHERICAL_SURFACE('',#50107,0.12) ;
#2173=SPHERICAL_SURFACE('',#50111,0.12) ;
#2174=SPHERICAL_SURFACE('',#50117,0.120000000000021) ;
#2175=SPHERICAL_SURFACE('',#50136,0.119999999999985) ;
#2251=PLANE('',#49874) ;
#2252=PLANE('',#49895) ;
#2253=PLANE('',#49896) ;
#2254=PLANE('',#49929) ;
#2255=PLANE('',#49976) ;
#2256=PLANE('',#49977) ;
#2257=PLANE('',#49980) ;
#2258=PLANE('',#50023) ;
#2259=PLANE('',#50027) ;
#2260=PLANE('',#50041) ;
#2261=PLANE('',#50055) ;
#2262=PLANE('',#50088) ;
#2263=PLANE('',#50089) ;
#2264=PLANE('',#50094) ;
#2265=PLANE('',#50095) ;
#2266=PLANE('',#50128) ;
#2267=PLANE('',#50129) ;
#2268=PLANE('',#50130) ;
#2269=PLANE('',#50135) ;
#2270=PLANE('',#50154) ;
#2271=PLANE('',#50155) ;
#2272=PLANE('',#50156) ;
#2273=PLANE('',#50157) ;
#2274=PLANE('',#50158) ;
#2275=PLANE('',#50159) ;
#2276=PLANE('',#50161) ;
#3186=LINE('',#75389,#6400) ;
#3187=LINE('',#75390,#6401) ;
#3188=LINE('',#75500,#6402) ;
#3189=LINE('',#75502,#6403) ;
#3190=LINE('',#75503,#6404) ;
#3191=LINE('',#75515,#6405) ;
#3192=LINE('',#75648,#6406) ;
#3193=LINE('',#75649,#6407) ;
#3194=LINE('',#75755,#6408) ;
#3195=LINE('',#75756,#6409) ;
#3196=LINE('',#75788,#6410) ;
#3197=LINE('',#75791,#6411) ;
#3198=LINE('',#75794,#6412) ;
#3199=LINE('',#75795,#6413) ;
#3200=LINE('',#75811,#6414) ;
#3201=LINE('',#75828,#6415) ;
#3202=LINE('',#75836,#6416) ;
#3203=LINE('',#75840,#6417) ;
#3204=LINE('',#75842,#6418) ;
#3205=LINE('',#75862,#6419) ;
#3206=LINE('',#75890,#6420) ;
#3207=LINE('',#75894,#6421) ;
#3208=LINE('',#75907,#6422) ;
#3209=LINE('',#75943,#6423) ;
#3210=LINE('',#75955,#6424) ;
#3211=LINE('',#75958,#6425) ;
#3212=LINE('',#75965,#6426) ;
#3213=LINE('',#76057,#6427) ;
#3214=LINE('',#76165,#6428) ;
#3215=LINE('',#76173,#6429) ;
#3216=LINE('',#76183,#6430) ;
#3217=LINE('',#76197,#6431) ;
#3218=LINE('',#76201,#6432) ;
#3219=LINE('',#76202,#6433) ;
#3220=LINE('',#76210,#6434) ;
#3221=LINE('',#76215,#6435) ;
#3222=LINE('',#76252,#6436) ;
#3223=LINE('',#76442,#6437) ;
#3224=LINE('',#76620,#6438) ;
#3225=LINE('',#76624,#6439) ;
#3226=LINE('',#76673,#6440) ;
#3227=LINE('',#76680,#6441) ;
#3228=LINE('',#76683,#6442) ;
#3229=LINE('',#76706,#6443) ;
#3230=LINE('',#76721,#6444) ;
#3231=LINE('',#76724,#6445) ;
#3232=LINE('',#76726,#6446) ;
#3233=LINE('',#76759,#6447) ;
#3234=LINE('',#76770,#6448) ;
#3235=LINE('',#76779,#6449) ;
#3236=LINE('',#76780,#6450) ;
#3237=LINE('',#76783,#6451) ;
#3238=LINE('',#76784,#6452) ;
#3239=LINE('',#76787,#6453) ;
#3240=LINE('',#76791,#6454) ;
#3241=LINE('',#76792,#6455) ;
#3242=LINE('',#76876,#6456) ;
#3243=LINE('',#76877,#6457) ;
#3244=LINE('',#76944,#6458) ;
#3245=LINE('',#76945,#6459) ;
#3246=LINE('',#76997,#6460) ;
#3247=LINE('',#76998,#6461) ;
#3248=LINE('',#77000,#6462) ;
#3249=LINE('',#77161,#6463) ;
#3250=LINE('',#77162,#6464) ;
#3251=LINE('',#77164,#6465) ;
#3252=LINE('',#77212,#6466) ;
#3253=LINE('',#77249,#6467) ;
#3254=LINE('',#77251,#6468) ;
#3255=LINE('',#77261,#6469) ;
#3256=LINE('',#77270,#6470) ;
#3257=LINE('',#77273,#6471) ;
#3258=LINE('',#77276,#6472) ;
#3259=LINE('',#77361,#6473) ;
#3260=LINE('',#77474,#6474) ;
#3261=LINE('',#77475,#6475) ;
#3262=LINE('',#77581,#6476) ;
#3263=LINE('',#77678,#6477) ;
#3264=LINE('',#77679,#6478) ;
#3265=LINE('',#77694,#6479) ;
#3266=LINE('',#77707,#6480) ;
#3267=LINE('',#77761,#6481) ;
#3268=LINE('',#77762,#6482) ;
#3269=LINE('',#77775,#6483) ;
#3270=LINE('',#77776,#6484) ;
#3271=LINE('',#77840,#6485) ;
#3272=LINE('',#77841,#6486) ;
#3273=LINE('',#77998,#6487) ;
#3274=LINE('',#77999,#6488) ;
#3275=LINE('',#78060,#6489) ;
#3276=LINE('',#78061,#6490) ;
#3277=LINE('',#78136,#6491) ;
#3278=LINE('',#78137,#6492) ;
#3279=LINE('',#78152,#6493) ;
#3280=LINE('',#78153,#6494) ;
#3281=LINE('',#78168,#6495) ;
#3282=LINE('',#78170,#6496) ;
#3283=LINE('',#78184,#6497) ;
#3284=LINE('',#78212,#6498) ;
#3285=LINE('',#78245,#6499) ;
#3286=LINE('',#78265,#6500) ;
#3287=LINE('',#78335,#6501) ;
#3288=LINE('',#78336,#6502) ;
#3289=LINE('',#78416,#6503) ;
#3290=LINE('',#78417,#6504) ;
#3291=LINE('',#78522,#6505) ;
#3292=LINE('',#78523,#6506) ;
#3293=LINE('',#78525,#6507) ;
#3294=LINE('',#78526,#6508) ;
#3295=LINE('',#78574,#6509) ;
#3296=LINE('',#78585,#6510) ;
#3297=LINE('',#78586,#6511) ;
#3298=LINE('',#78588,#6512) ;
#3299=LINE('',#78589,#6513) ;
#3300=LINE('',#78615,#6514) ;
#3301=LINE('',#78736,#6515) ;
#3302=LINE('',#78737,#6516) ;
#3303=LINE('',#78752,#6517) ;
#3304=LINE('',#78765,#6518) ;
#3305=LINE('',#78768,#6519) ;
#3306=LINE('',#78769,#6520) ;
#3307=LINE('',#78903,#6521) ;
#3308=LINE('',#79044,#6522) ;
#3309=LINE('',#79045,#6523) ;
#3310=LINE('',#79060,#6524) ;
#3311=LINE('',#79081,#6525) ;
#3312=LINE('',#79102,#6526) ;
#3313=LINE('',#79103,#6527) ;
#3314=LINE('',#79112,#6528) ;
#3315=LINE('',#79121,#6529) ;
#3316=LINE('',#79132,#6530) ;
#3317=LINE('',#79133,#6531) ;
#3318=LINE('',#79147,#6532) ;
#3319=LINE('',#79156,#6533) ;
#3320=LINE('',#79189,#6534) ;
#3321=LINE('',#79192,#6535) ;
#3322=LINE('',#79194,#6536) ;
#6400=VECTOR('',#56379,10.) ;
#6401=VECTOR('',#56380,10.) ;
#6402=VECTOR('',#56383,10.) ;
#6403=VECTOR('',#56384,10.) ;
#6404=VECTOR('',#56385,10.) ;
#6405=VECTOR('',#56386,10.) ;
#6406=VECTOR('',#56407,10.) ;
#6407=VECTOR('',#56408,10.) ;
#6408=VECTOR('',#56423,10.) ;
#6409=VECTOR('',#56424,10.) ;
#6410=VECTOR('',#56429,10.) ;
#6411=VECTOR('',#56432,10.) ;
#6412=VECTOR('',#56435,10.) ;
#6413=VECTOR('',#56436,10.) ;
#6414=VECTOR('',#56437,10.) ;
#6415=VECTOR('',#56438,10.) ;
#6416=VECTOR('',#56441,10.) ;
#6417=VECTOR('',#56444,10.) ;
#6418=VECTOR('',#56445,10.) ;
#6419=VECTOR('',#56458,10.) ;
#6420=VECTOR('',#56465,10.) ;
#6421=VECTOR('',#56468,10.) ;
#6422=VECTOR('',#56473,10.) ;
#6423=VECTOR('',#56480,10.) ;
#6424=VECTOR('',#56485,10.) ;
#6425=VECTOR('',#56488,10.) ;
#6426=VECTOR('',#56495,10.) ;
#6427=VECTOR('',#56510,10.) ;
#6428=VECTOR('',#56515,10.) ;
#6429=VECTOR('',#56516,10.) ;
#6430=VECTOR('',#56517,10.) ;
#6431=VECTOR('',#56518,10.) ;
#6432=VECTOR('',#56523,10.) ;
#6433=VECTOR('',#56524,10.) ;
#6434=VECTOR('',#56535,2.) ;
#6435=VECTOR('',#56540,10.) ;
#6436=VECTOR('',#56549,10.) ;
#6437=VECTOR('',#56572,10.) ;
#6438=VECTOR('',#56601,10.) ;
#6439=VECTOR('',#56606,10.) ;
#6440=VECTOR('',#56611,10.) ;
#6441=VECTOR('',#56612,10.) ;
#6442=VECTOR('',#56615,10.) ;
#6443=VECTOR('',#56618,10.) ;
#6444=VECTOR('',#56621,10.) ;
#6445=VECTOR('',#56624,10.) ;
#6446=VECTOR('',#56625,10.) ;
#6447=VECTOR('',#56628,10.) ;
#6448=VECTOR('',#56631,10.) ;
#6449=VECTOR('',#56634,10.) ;
#6450=VECTOR('',#56635,10.) ;
#6451=VECTOR('',#56638,10.) ;
#6452=VECTOR('',#56639,10.) ;
#6453=VECTOR('',#56642,10.) ;
#6454=VECTOR('',#56647,10.) ;
#6455=VECTOR('',#56648,10.) ;
#6456=VECTOR('',#56665,10.) ;
#6457=VECTOR('',#56666,10.) ;
#6458=VECTOR('',#56681,10.) ;
#6459=VECTOR('',#56682,10.) ;
#6460=VECTOR('',#56697,10.) ;
#6461=VECTOR('',#56698,10.) ;
#6462=VECTOR('',#56701,10.) ;
#6463=VECTOR('',#56726,10.) ;
#6464=VECTOR('',#56727,10.) ;
#6465=VECTOR('',#56730,10.) ;
#6466=VECTOR('',#56741,10.) ;
#6467=VECTOR('',#56746,10.) ;
#6468=VECTOR('',#56747,10.) ;
#6469=VECTOR('',#56750,10.) ;
#6470=VECTOR('',#56751,10.) ;
#6471=VECTOR('',#56754,10.) ;
#6472=VECTOR('',#56757,10.) ;
#6473=VECTOR('',#56776,10.) ;
#6474=VECTOR('',#56787,10.) ;
#6475=VECTOR('',#56788,10.) ;
#6476=VECTOR('',#56805,10.) ;
#6477=VECTOR('',#56818,10.) ;
#6478=VECTOR('',#56819,10.) ;
#6479=VECTOR('',#56820,10.) ;
#6480=VECTOR('',#56821,10.) ;
#6481=VECTOR('',#56838,10.) ;
#6482=VECTOR('',#56839,10.) ;
#6483=VECTOR('',#56854,10.) ;
#6484=VECTOR('',#56855,10.) ;
#6485=VECTOR('',#56868,10.) ;
#6486=VECTOR('',#56869,10.) ;
#6487=VECTOR('',#56878,10.) ;
#6488=VECTOR('',#56879,10.) ;
#6489=VECTOR('',#56892,10.) ;
#6490=VECTOR('',#56893,10.) ;
#6491=VECTOR('',#56898,10.) ;
#6492=VECTOR('',#56899,10.) ;
#6493=VECTOR('',#56900,10.) ;
#6494=VECTOR('',#56901,10.) ;
#6495=VECTOR('',#56902,10.) ;
#6496=VECTOR('',#56905,10.) ;
#6497=VECTOR('',#56910,10.) ;
#6498=VECTOR('',#56911,10.) ;
#6499=VECTOR('',#56918,10.) ;
#6500=VECTOR('',#56919,10.) ;
#6501=VECTOR('',#56936,10.) ;
#6502=VECTOR('',#56937,10.) ;
#6503=VECTOR('',#56956,10.) ;
#6504=VECTOR('',#56957,10.) ;
#6505=VECTOR('',#56980,10.) ;
#6506=VECTOR('',#56981,10.) ;
#6507=VECTOR('',#56984,10.) ;
#6508=VECTOR('',#56985,10.) ;
#6509=VECTOR('',#56992,10.) ;
#6510=VECTOR('',#56993,10.) ;
#6511=VECTOR('',#56994,10.) ;
#6512=VECTOR('',#56997,10.) ;
#6513=VECTOR('',#56998,10.) ;
#6514=VECTOR('',#57001,10.) ;
#6515=VECTOR('',#57016,10.) ;
#6516=VECTOR('',#57017,10.) ;
#6517=VECTOR('',#57018,10.) ;
#6518=VECTOR('',#57019,10.) ;
#6519=VECTOR('',#57022,10.) ;
#6520=VECTOR('',#57023,10.) ;
#6521=VECTOR('',#57050,10.) ;
#6522=VECTOR('',#57063,10.) ;
#6523=VECTOR('',#57064,10.) ;
#6524=VECTOR('',#57065,10.) ;
#6525=VECTOR('',#57066,10.) ;
#6526=VECTOR('',#57069,10.) ;
#6527=VECTOR('',#57070,10.) ;
#6528=VECTOR('',#57071,10.) ;
#6529=VECTOR('',#57072,10.) ;
#6530=VECTOR('',#57073,10.) ;
#6531=VECTOR('',#57074,10.) ;
#6532=VECTOR('',#57077,10.) ;
#6533=VECTOR('',#57078,10.) ;
#6534=VECTOR('',#57083,10.) ;
#6535=VECTOR('',#57088,10.) ;
#6536=VECTOR('',#57091,10.) ;
#9557=CYLINDRICAL_SURFACE('',#49872,0.12) ;
#9558=CYLINDRICAL_SURFACE('',#49883,0.12) ;
#9559=CYLINDRICAL_SURFACE('',#49890,0.12) ;
#9560=CYLINDRICAL_SURFACE('',#49917,0.12) ;
#9561=CYLINDRICAL_SURFACE('',#49924,0.12) ;
#9562=CYLINDRICAL_SURFACE('',#49933,2.) ;
#9563=CYLINDRICAL_SURFACE('',#49935,0.12) ;
#9564=CYLINDRICAL_SURFACE('',#49940,0.12) ;
#9565=CYLINDRICAL_SURFACE('',#49950,0.12) ;
#9566=CYLINDRICAL_SURFACE('',#49965,0.12) ;
#9567=CYLINDRICAL_SURFACE('',#49967,0.12) ;
#9568=CYLINDRICAL_SURFACE('',#49970,33.2107853000911) ;
#9569=CYLINDRICAL_SURFACE('',#49978,3.6) ;
#9570=CYLINDRICAL_SURFACE('',#50002,0.12) ;
#9571=CYLINDRICAL_SURFACE('',#50003,0.12) ;
#9572=CYLINDRICAL_SURFACE('',#50015,0.12) ;
#9573=CYLINDRICAL_SURFACE('',#50016,0.12) ;
#9574=CYLINDRICAL_SURFACE('',#50021,0.12) ;
#9575=CYLINDRICAL_SURFACE('',#50025,34.9868507372267) ;
#9576=CYLINDRICAL_SURFACE('',#50034,0.12) ;
#9577=CYLINDRICAL_SURFACE('',#50040,0.12) ;
#9578=CYLINDRICAL_SURFACE('',#50047,0.12) ;
#9579=CYLINDRICAL_SURFACE('',#50054,0.12) ;
#9580=CYLINDRICAL_SURFACE('',#50069,0.12) ;
#9581=CYLINDRICAL_SURFACE('',#50074,0.12) ;
#9582=CYLINDRICAL_SURFACE('',#50084,0.12) ;
#9583=CYLINDRICAL_SURFACE('',#50087,0.12) ;
#9584=CYLINDRICAL_SURFACE('',#50122,0.12) ;
#9585=CYLINDRICAL_SURFACE('',#50125,0.12) ;
#9586=CYLINDRICAL_SURFACE('',#50126,0.12) ;
#9587=CYLINDRICAL_SURFACE('',#50127,0.12) ;
#9588=CYLINDRICAL_SURFACE('',#50147,0.12) ;
#9589=CYLINDRICAL_SURFACE('',#50153,0.12) ;
#9590=CYLINDRICAL_SURFACE('',#50162,3.6) ;
#9591=CYLINDRICAL_SURFACE('',#50163,3.6) ;
#11006=FACE_OUTER_BOUND('',#14099,.T.) ;
#11007=FACE_OUTER_BOUND('',#14100,.T.) ;
#11008=FACE_OUTER_BOUND('',#14101,.T.) ;
#11009=FACE_OUTER_BOUND('',#14102,.T.) ;
#11010=FACE_OUTER_BOUND('',#14103,.T.) ;
#11011=FACE_OUTER_BOUND('',#14104,.T.) ;
#11012=FACE_OUTER_BOUND('',#14105,.T.) ;
#11013=FACE_OUTER_BOUND('',#14106,.T.) ;
#11014=FACE_OUTER_BOUND('',#14107,.T.) ;
#11015=FACE_OUTER_BOUND('',#14108,.T.) ;
#11016=FACE_OUTER_BOUND('',#14109,.T.) ;
#11017=FACE_OUTER_BOUND('',#14110,.T.) ;
#11018=FACE_OUTER_BOUND('',#14111,.T.) ;
#11019=FACE_OUTER_BOUND('',#14112,.T.) ;
#11020=FACE_OUTER_BOUND('',#14113,.T.) ;
#11021=FACE_OUTER_BOUND('',#14114,.T.) ;
#11022=FACE_OUTER_BOUND('',#14115,.T.) ;
#11023=FACE_OUTER_BOUND('',#14116,.T.) ;
#11024=FACE_OUTER_BOUND('',#14117,.T.) ;
#11025=FACE_OUTER_BOUND('',#14118,.T.) ;
#11026=FACE_OUTER_BOUND('',#14119,.T.) ;
#11027=FACE_OUTER_BOUND('',#14120,.T.) ;
#11028=FACE_OUTER_BOUND('',#14125,.T.) ;
#11029=FACE_OUTER_BOUND('',#14126,.T.) ;
#11030=FACE_OUTER_BOUND('',#14127,.T.) ;
#11031=FACE_OUTER_BOUND('',#14128,.T.) ;
#11032=FACE_OUTER_BOUND('',#14129,.T.) ;
#11033=FACE_OUTER_BOUND('',#14130,.T.) ;
#11034=FACE_OUTER_BOUND('',#14131,.T.) ;
#11035=FACE_OUTER_BOUND('',#14132,.T.) ;
#11036=FACE_OUTER_BOUND('',#14133,.T.) ;
#11037=FACE_OUTER_BOUND('',#14134,.T.) ;
#11038=FACE_OUTER_BOUND('',#14135,.T.) ;
#11039=FACE_OUTER_BOUND('',#14136,.T.) ;
#11040=FACE_OUTER_BOUND('',#14137,.T.) ;
#11041=FACE_OUTER_BOUND('',#14138,.T.) ;
#11042=FACE_OUTER_BOUND('',#14139,.T.) ;
#11043=FACE_OUTER_BOUND('',#14140,.T.) ;
#11044=FACE_OUTER_BOUND('',#14141,.T.) ;
#11045=FACE_OUTER_BOUND('',#14142,.T.) ;
#11046=FACE_OUTER_BOUND('',#14143,.T.) ;
#11047=FACE_OUTER_BOUND('',#14144,.T.) ;
#11048=FACE_OUTER_BOUND('',#14145,.T.) ;
#11049=FACE_OUTER_BOUND('',#14146,.T.) ;
#11050=FACE_OUTER_BOUND('',#14147,.T.) ;
#11051=FACE_OUTER_BOUND('',#14148,.T.) ;
#11052=FACE_OUTER_BOUND('',#14149,.T.) ;
#11053=FACE_OUTER_BOUND('',#14150,.T.) ;
#11054=FACE_OUTER_BOUND('',#14151,.T.) ;
#11055=FACE_OUTER_BOUND('',#14152,.T.) ;
#11056=FACE_OUTER_BOUND('',#14153,.T.) ;
#11057=FACE_OUTER_BOUND('',#14154,.T.) ;
#11058=FACE_OUTER_BOUND('',#14155,.T.) ;
#11059=FACE_OUTER_BOUND('',#14156,.T.) ;
#11060=FACE_OUTER_BOUND('',#14157,.T.) ;
#11061=FACE_OUTER_BOUND('',#14158,.T.) ;
#11062=FACE_OUTER_BOUND('',#14159,.T.) ;
#11063=FACE_OUTER_BOUND('',#14160,.T.) ;
#11064=FACE_OUTER_BOUND('',#14161,.T.) ;
#11065=FACE_OUTER_BOUND('',#14162,.T.) ;
#11066=FACE_OUTER_BOUND('',#14163,.T.) ;
#11067=FACE_OUTER_BOUND('',#14164,.T.) ;
#11068=FACE_OUTER_BOUND('',#14165,.T.) ;
#11069=FACE_OUTER_BOUND('',#14166,.T.) ;
#11070=FACE_OUTER_BOUND('',#14167,.T.) ;
#11071=FACE_OUTER_BOUND('',#14168,.T.) ;
#11072=FACE_OUTER_BOUND('',#14169,.T.) ;
#11073=FACE_OUTER_BOUND('',#14170,.T.) ;
#11074=FACE_OUTER_BOUND('',#14171,.T.) ;
#11075=FACE_OUTER_BOUND('',#14172,.T.) ;
#11076=FACE_OUTER_BOUND('',#14173,.T.) ;
#11077=FACE_OUTER_BOUND('',#14174,.T.) ;
#11078=FACE_OUTER_BOUND('',#14175,.T.) ;
#11079=FACE_OUTER_BOUND('',#14176,.T.) ;
#11080=FACE_OUTER_BOUND('',#14177,.T.) ;
#11081=FACE_OUTER_BOUND('',#14178,.T.) ;
#11082=FACE_OUTER_BOUND('',#14179,.T.) ;
#11083=FACE_OUTER_BOUND('',#14180,.T.) ;
#11084=FACE_OUTER_BOUND('',#14181,.T.) ;
#11085=FACE_OUTER_BOUND('',#14182,.T.) ;
#11086=FACE_OUTER_BOUND('',#14183,.T.) ;
#11087=FACE_OUTER_BOUND('',#14184,.T.) ;
#11088=FACE_OUTER_BOUND('',#14185,.T.) ;
#11089=FACE_OUTER_BOUND('',#14186,.T.) ;
#11090=FACE_OUTER_BOUND('',#14187,.T.) ;
#11091=FACE_OUTER_BOUND('',#14188,.T.) ;
#11092=FACE_OUTER_BOUND('',#14189,.T.) ;
#11093=FACE_OUTER_BOUND('',#14190,.T.) ;
#11094=FACE_OUTER_BOUND('',#14191,.T.) ;
#11095=FACE_OUTER_BOUND('',#14192,.T.) ;
#11096=FACE_OUTER_BOUND('',#14193,.T.) ;
#11097=FACE_OUTER_BOUND('',#14194,.T.) ;
#11098=FACE_OUTER_BOUND('',#14195,.T.) ;
#11099=FACE_OUTER_BOUND('',#14196,.T.) ;
#11100=FACE_OUTER_BOUND('',#14197,.T.) ;
#11101=FACE_OUTER_BOUND('',#14198,.T.) ;
#11102=FACE_OUTER_BOUND('',#14199,.T.) ;
#11103=FACE_OUTER_BOUND('',#14200,.T.) ;
#11104=FACE_OUTER_BOUND('',#14201,.T.) ;
#11105=FACE_OUTER_BOUND('',#14202,.T.) ;
#11106=FACE_OUTER_BOUND('',#14203,.T.) ;
#11107=FACE_OUTER_BOUND('',#14204,.T.) ;
#11108=FACE_OUTER_BOUND('',#14205,.T.) ;
#11109=FACE_OUTER_BOUND('',#14206,.T.) ;
#11110=FACE_OUTER_BOUND('',#14207,.T.) ;
#11111=FACE_OUTER_BOUND('',#14208,.T.) ;
#11112=FACE_OUTER_BOUND('',#14209,.T.) ;
#11113=FACE_OUTER_BOUND('',#14210,.T.) ;
#11114=FACE_OUTER_BOUND('',#14211,.T.) ;
#11115=FACE_OUTER_BOUND('',#14212,.T.) ;
#11116=FACE_OUTER_BOUND('',#14213,.T.) ;
#11117=FACE_OUTER_BOUND('',#14214,.T.) ;
#11118=FACE_OUTER_BOUND('',#14215,.T.) ;
#11119=FACE_OUTER_BOUND('',#14216,.T.) ;
#11120=FACE_OUTER_BOUND('',#14217,.T.) ;
#11121=FACE_OUTER_BOUND('',#14218,.T.) ;
#11122=FACE_OUTER_BOUND('',#14219,.T.) ;
#11123=FACE_OUTER_BOUND('',#14220,.T.) ;
#11124=FACE_OUTER_BOUND('',#14221,.T.) ;
#11125=FACE_OUTER_BOUND('',#14222,.T.) ;
#11126=FACE_OUTER_BOUND('',#14223,.T.) ;
#11127=FACE_OUTER_BOUND('',#14224,.T.) ;
#11128=FACE_OUTER_BOUND('',#14225,.T.) ;
#11129=FACE_OUTER_BOUND('',#14226,.T.) ;
#11130=FACE_OUTER_BOUND('',#14227,.T.) ;
#11131=FACE_OUTER_BOUND('',#14228,.T.) ;
#11132=FACE_OUTER_BOUND('',#14229,.T.) ;
#11133=FACE_OUTER_BOUND('',#14230,.T.) ;
#11134=FACE_OUTER_BOUND('',#14231,.T.) ;
#11135=FACE_OUTER_BOUND('',#14232,.T.) ;
#11136=FACE_OUTER_BOUND('',#14233,.T.) ;
#11137=FACE_OUTER_BOUND('',#14234,.T.) ;
#11138=FACE_OUTER_BOUND('',#14235,.T.) ;
#11139=FACE_OUTER_BOUND('',#14236,.T.) ;
#11140=FACE_OUTER_BOUND('',#14237,.T.) ;
#11141=FACE_OUTER_BOUND('',#14238,.T.) ;
#11142=FACE_OUTER_BOUND('',#14241,.T.) ;
#11143=FACE_OUTER_BOUND('',#14242,.T.) ;
#11144=FACE_OUTER_BOUND('',#14243,.T.) ;
#11145=FACE_OUTER_BOUND('',#14244,.T.) ;
#11146=FACE_OUTER_BOUND('',#14245,.T.) ;
#11147=FACE_OUTER_BOUND('',#14246,.T.) ;
#11148=FACE_OUTER_BOUND('',#14247,.T.) ;
#11149=FACE_OUTER_BOUND('',#14248,.T.) ;
#11150=FACE_OUTER_BOUND('',#14249,.T.) ;
#11151=FACE_OUTER_BOUND('',#14250,.T.) ;
#11152=FACE_OUTER_BOUND('',#14251,.T.) ;
#11153=FACE_OUTER_BOUND('',#14252,.T.) ;
#11154=FACE_OUTER_BOUND('',#14253,.T.) ;
#11155=FACE_OUTER_BOUND('',#14254,.T.) ;
#11156=FACE_OUTER_BOUND('',#14255,.T.) ;
#11157=FACE_OUTER_BOUND('',#14256,.T.) ;
#11158=FACE_OUTER_BOUND('',#14257,.T.) ;
#11159=FACE_OUTER_BOUND('',#14258,.T.) ;
#11160=FACE_OUTER_BOUND('',#14259,.T.) ;
#11161=FACE_OUTER_BOUND('',#14260,.T.) ;
#11162=FACE_OUTER_BOUND('',#14261,.T.) ;
#11163=FACE_OUTER_BOUND('',#14262,.T.) ;
#11164=FACE_OUTER_BOUND('',#14263,.T.) ;
#11165=FACE_OUTER_BOUND('',#14264,.T.) ;
#11166=FACE_OUTER_BOUND('',#14265,.T.) ;
#11167=FACE_OUTER_BOUND('',#14266,.T.) ;
#11168=FACE_OUTER_BOUND('',#14267,.T.) ;
#11169=FACE_OUTER_BOUND('',#14268,.T.) ;
#11170=FACE_OUTER_BOUND('',#14269,.T.) ;
#11171=FACE_OUTER_BOUND('',#14270,.T.) ;
#11172=FACE_OUTER_BOUND('',#14271,.T.) ;
#11173=FACE_OUTER_BOUND('',#14272,.T.) ;
#11174=FACE_OUTER_BOUND('',#14273,.T.) ;
#11175=FACE_OUTER_BOUND('',#14274,.T.) ;
#11176=FACE_OUTER_BOUND('',#14275,.T.) ;
#11177=FACE_OUTER_BOUND('',#14276,.T.) ;
#11178=FACE_OUTER_BOUND('',#14277,.T.) ;
#11179=FACE_OUTER_BOUND('',#14278,.T.) ;
#11180=FACE_OUTER_BOUND('',#14279,.T.) ;
#11181=FACE_OUTER_BOUND('',#14280,.T.) ;
#11182=FACE_OUTER_BOUND('',#14281,.T.) ;
#11183=FACE_OUTER_BOUND('',#14282,.T.) ;
#11184=FACE_OUTER_BOUND('',#14283,.T.) ;
#11185=FACE_OUTER_BOUND('',#14284,.T.) ;
#11186=FACE_OUTER_BOUND('',#14285,.T.) ;
#11187=FACE_OUTER_BOUND('',#14286,.T.) ;
#11188=FACE_OUTER_BOUND('',#14287,.T.) ;
#11189=FACE_OUTER_BOUND('',#14288,.T.) ;
#11190=FACE_OUTER_BOUND('',#14289,.T.) ;
#11191=FACE_OUTER_BOUND('',#14290,.T.) ;
#11192=FACE_OUTER_BOUND('',#14291,.T.) ;
#11193=FACE_OUTER_BOUND('',#14292,.T.) ;
#11194=FACE_OUTER_BOUND('',#14293,.T.) ;
#11195=FACE_OUTER_BOUND('',#14294,.T.) ;
#11196=FACE_OUTER_BOUND('',#14295,.T.) ;
#11197=FACE_OUTER_BOUND('',#14296,.T.) ;
#11198=FACE_OUTER_BOUND('',#14297,.T.) ;
#11199=FACE_OUTER_BOUND('',#14298,.T.) ;
#11200=FACE_OUTER_BOUND('',#14299,.T.) ;
#11201=FACE_OUTER_BOUND('',#14300,.T.) ;
#11202=FACE_OUTER_BOUND('',#14301,.T.) ;
#11203=FACE_OUTER_BOUND('',#14302,.T.) ;
#11204=FACE_OUTER_BOUND('',#14303,.T.) ;
#11205=FACE_OUTER_BOUND('',#14306,.T.) ;
#11206=FACE_OUTER_BOUND('',#14307,.T.) ;
#11207=FACE_OUTER_BOUND('',#14308,.T.) ;
#14099=EDGE_LOOP('',(#32174,#32175,#32176,#32177)) ;
#14100=EDGE_LOOP('',(#32178,#32179,#32180,#32181)) ;
#14101=EDGE_LOOP('',(#32182,#32183,#32184,#32185)) ;
#14102=EDGE_LOOP('',(#32186,#32187,#32188,#32189)) ;
#14103=EDGE_LOOP('',(#32190,#32191,#32192,#32193)) ;
#14104=EDGE_LOOP('',(#32194,#32195,#32196,#32197)) ;
#14105=EDGE_LOOP('',(#32198,#32199,#32200,#32201,#32202,#32203)) ;
#14106=EDGE_LOOP('',(#32204,#32205,#32206,#32207)) ;
#14107=EDGE_LOOP('',(#32208,#32209,#32210,#32211,#32212)) ;
#14108=EDGE_LOOP('',(#32213,#32214,#32215,#32216)) ;
#14109=EDGE_LOOP('',(#32217,#32218,#32219,#32220)) ;
#14110=EDGE_LOOP('',(#32221,#32222,#32223,#32224)) ;
#14111=EDGE_LOOP('',(#32225,#32226,#32227,#32228)) ;
#14112=EDGE_LOOP('',(#32229,#32230,#32231,#32232)) ;
#14113=EDGE_LOOP('',(#32233,#32234,#32235,#32236)) ;
#14114=EDGE_LOOP('',(#32237,#32238,#32239,#32240)) ;
#14115=EDGE_LOOP('',(#32241,#32242,#32243,#32244)) ;
#14116=EDGE_LOOP('',(#32245,#32246,#32247,#32248)) ;
#14117=EDGE_LOOP('',(#32249,#32250,#32251,#32252)) ;
#14118=EDGE_LOOP('',(#32253,#32254,#32255,#32256)) ;
#14119=EDGE_LOOP('',(#32257,#32258,#32259,#32260)) ;
#14120=EDGE_LOOP('',(#32261,#32262,#32263,#32264,#32265,#32266,#32267,#32268,
#32269,#32270,#32271,#32272,#32273,#32274,#32275,#32276,#32277,#32278,#32279,
#32280)) ;
#14121=EDGE_LOOP('',(#32281,#32282,#32283,#32284,#32285,#32286,#32287,#32288)) ;
#14122=EDGE_LOOP('',(#32289,#32290,#32291,#32292,#32293,#32294,#32295,#32296,
#32297,#32298,#32299)) ;
#14123=EDGE_LOOP('',(#32300)) ;
#14124=EDGE_LOOP('',(#32301,#32302,#32303,#32304,#32305,#32306,#32307,#32308)) ;
#14125=EDGE_LOOP('',(#32309,#32310,#32311,#32312)) ;
#14126=EDGE_LOOP('',(#32313,#32314,#32315,#32316)) ;
#14127=EDGE_LOOP('',(#32317,#32318,#32319,#32320)) ;
#14128=EDGE_LOOP('',(#32321,#32322,#32323,#32324)) ;
#14129=EDGE_LOOP('',(#32325,#32326,#32327,#32328)) ;
#14130=EDGE_LOOP('',(#32329,#32330,#32331,#32332)) ;
#14131=EDGE_LOOP('',(#32333,#32334,#32335,#32336)) ;
#14132=EDGE_LOOP('',(#32337,#32338,#32339,#32340)) ;
#14133=EDGE_LOOP('',(#32341,#32342,#32343,#32344)) ;
#14134=EDGE_LOOP('',(#32345,#32346,#32347,#32348)) ;
#14135=EDGE_LOOP('',(#32349,#32350,#32351,#32352)) ;
#14136=EDGE_LOOP('',(#32353,#32354,#32355,#32356)) ;
#14137=EDGE_LOOP('',(#32357,#32358,#32359,#32360)) ;
#14138=EDGE_LOOP('',(#32361,#32362,#32363,#32364)) ;
#14139=EDGE_LOOP('',(#32365,#32366,#32367,#32368)) ;
#14140=EDGE_LOOP('',(#32369,#32370,#32371,#32372)) ;
#14141=EDGE_LOOP('',(#32373,#32374,#32375,#32376)) ;
#14142=EDGE_LOOP('',(#32377,#32378,#32379,#32380)) ;
#14143=EDGE_LOOP('',(#32381,#32382,#32383,#32384)) ;
#14144=EDGE_LOOP('',(#32385,#32386,#32387,#32388)) ;
#14145=EDGE_LOOP('',(#32389,#32390,#32391,#32392)) ;
#14146=EDGE_LOOP('',(#32393,#32394,#32395,#32396)) ;
#14147=EDGE_LOOP('',(#32397,#32398,#32399,#32400)) ;
#14148=EDGE_LOOP('',(#32401,#32402,#32403,#32404)) ;
#14149=EDGE_LOOP('',(#32405,#32406,#32407,#32408)) ;
#14150=EDGE_LOOP('',(#32409,#32410,#32411,#32412)) ;
#14151=EDGE_LOOP('',(#32413,#32414,#32415,#32416)) ;
#14152=EDGE_LOOP('',(#32417,#32418,#32419,#32420)) ;
#14153=EDGE_LOOP('',(#32421,#32422,#32423,#32424)) ;
#14154=EDGE_LOOP('',(#32425,#32426,#32427,#32428)) ;
#14155=EDGE_LOOP('',(#32429,#32430,#32431,#32432)) ;
#14156=EDGE_LOOP('',(#32433,#32434,#32435,#32436)) ;
#14157=EDGE_LOOP('',(#32437,#32438,#32439,#32440)) ;
#14158=EDGE_LOOP('',(#32441,#32442,#32443,#32444)) ;
#14159=EDGE_LOOP('',(#32445,#32446,#32447,#32448)) ;
#14160=EDGE_LOOP('',(#32449,#32450,#32451,#32452)) ;
#14161=EDGE_LOOP('',(#32453,#32454,#32455,#32456)) ;
#14162=EDGE_LOOP('',(#32457,#32458,#32459,#32460,#32461,#32462,#32463)) ;
#14163=EDGE_LOOP('',(#32464,#32465,#32466,#32467,#32468,#32469,#32470)) ;
#14164=EDGE_LOOP('',(#32471,#32472,#32473,#32474)) ;
#14165=EDGE_LOOP('',(#32475,#32476,#32477,#32478)) ;
#14166=EDGE_LOOP('',(#32479,#32480,#32481,#32482)) ;
#14167=EDGE_LOOP('',(#32483,#32484,#32485,#32486)) ;
#14168=EDGE_LOOP('',(#32487,#32488,#32489,#32490)) ;
#14169=EDGE_LOOP('',(#32491,#32492,#32493,#32494)) ;
#14170=EDGE_LOOP('',(#32495,#32496,#32497,#32498)) ;
#14171=EDGE_LOOP('',(#32499,#32500,#32501)) ;
#14172=EDGE_LOOP('',(#32502,#32503,#32504,#32505)) ;
#14173=EDGE_LOOP('',(#32506,#32507,#32508,#32509)) ;
#14174=EDGE_LOOP('',(#32510,#32511,#32512,#32513)) ;
#14175=EDGE_LOOP('',(#32514,#32515,#32516,#32517,#32518)) ;
#14176=EDGE_LOOP('',(#32519,#32520,#32521,#32522)) ;
#14177=EDGE_LOOP('',(#32523,#32524,#32525,#32526)) ;
#14178=EDGE_LOOP('',(#32527,#32528,#32529,#32530)) ;
#14179=EDGE_LOOP('',(#32531,#32532,#32533,#32534)) ;
#14180=EDGE_LOOP('',(#32535,#32536,#32537,#32538)) ;
#14181=EDGE_LOOP('',(#32539,#32540,#32541,#32542)) ;
#14182=EDGE_LOOP('',(#32543,#32544,#32545,#32546)) ;
#14183=EDGE_LOOP('',(#32547,#32548,#32549,#32550)) ;
#14184=EDGE_LOOP('',(#32551,#32552,#32553,#32554)) ;
#14185=EDGE_LOOP('',(#32555,#32556,#32557,#32558)) ;
#14186=EDGE_LOOP('',(#32559,#32560,#32561,#32562)) ;
#14187=EDGE_LOOP('',(#32563,#32564,#32565,#32566)) ;
#14188=EDGE_LOOP('',(#32567,#32568,#32569,#32570)) ;
#14189=EDGE_LOOP('',(#32571,#32572,#32573,#32574)) ;
#14190=EDGE_LOOP('',(#32575,#32576,#32577)) ;
#14191=EDGE_LOOP('',(#32578,#32579,#32580,#32581,#32582,#32583,#32584,#32585,
#32586,#32587)) ;
#14192=EDGE_LOOP('',(#32588,#32589,#32590,#32591)) ;
#14193=EDGE_LOOP('',(#32592,#32593,#32594,#32595)) ;
#14194=EDGE_LOOP('',(#32596,#32597,#32598,#32599,#32600)) ;
#14195=EDGE_LOOP('',(#32601,#32602,#32603,#32604)) ;
#14196=EDGE_LOOP('',(#32605,#32606,#32607,#32608)) ;
#14197=EDGE_LOOP('',(#32609,#32610,#32611,#32612)) ;
#14198=EDGE_LOOP('',(#32613,#32614,#32615,#32616)) ;
#14199=EDGE_LOOP('',(#32617,#32618,#32619,#32620)) ;
#14200=EDGE_LOOP('',(#32621,#32622,#32623,#32624)) ;
#14201=EDGE_LOOP('',(#32625,#32626,#32627,#32628)) ;
#14202=EDGE_LOOP('',(#32629,#32630,#32631,#32632)) ;
#14203=EDGE_LOOP('',(#32633,#32634,#32635,#32636)) ;
#14204=EDGE_LOOP('',(#32637,#32638,#32639,#32640,#32641,#32642,#32643,#32644)) ;
#14205=EDGE_LOOP('',(#32645,#32646,#32647,#32648)) ;
#14206=EDGE_LOOP('',(#32649,#32650,#32651,#32652)) ;
#14207=EDGE_LOOP('',(#32653,#32654,#32655,#32656)) ;
#14208=EDGE_LOOP('',(#32657,#32658,#32659,#32660)) ;
#14209=EDGE_LOOP('',(#32661,#32662,#32663,#32664)) ;
#14210=EDGE_LOOP('',(#32665,#32666,#32667,#32668)) ;
#14211=EDGE_LOOP('',(#32669,#32670,#32671,#32672)) ;
#14212=EDGE_LOOP('',(#32673,#32674,#32675,#32676)) ;
#14213=EDGE_LOOP('',(#32677,#32678,#32679,#32680)) ;
#14214=EDGE_LOOP('',(#32681,#32682,#32683,#32684)) ;
#14215=EDGE_LOOP('',(#32685,#32686,#32687,#32688,#32689,#32690,#32691,#32692)) ;
#14216=EDGE_LOOP('',(#32693,#32694,#32695)) ;
#14217=EDGE_LOOP('',(#32696,#32697,#32698,#32699)) ;
#14218=EDGE_LOOP('',(#32700,#32701,#32702,#32703)) ;
#14219=EDGE_LOOP('',(#32704,#32705,#32706,#32707,#32708)) ;
#14220=EDGE_LOOP('',(#32709,#32710,#32711,#32712)) ;
#14221=EDGE_LOOP('',(#32713,#32714,#32715,#32716)) ;
#14222=EDGE_LOOP('',(#32717,#32718,#32719,#32720)) ;
#14223=EDGE_LOOP('',(#32721,#32722,#32723,#32724)) ;
#14224=EDGE_LOOP('',(#32725,#32726,#32727,#32728)) ;
#14225=EDGE_LOOP('',(#32729,#32730,#32731,#32732)) ;
#14226=EDGE_LOOP('',(#32733,#32734,#32735,#32736,#32737,#32738)) ;
#14227=EDGE_LOOP('',(#32739,#32740,#32741,#32742,#32743,#32744)) ;
#14228=EDGE_LOOP('',(#32745,#32746,#32747,#32748)) ;
#14229=EDGE_LOOP('',(#32749,#32750,#32751,#32752)) ;
#14230=EDGE_LOOP('',(#32753,#32754,#32755,#32756)) ;
#14231=EDGE_LOOP('',(#32757,#32758,#32759,#32760)) ;
#14232=EDGE_LOOP('',(#32761,#32762,#32763,#32764)) ;
#14233=EDGE_LOOP('',(#32765,#32766,#32767,#32768)) ;
#14234=EDGE_LOOP('',(#32769,#32770,#32771,#32772)) ;
#14235=EDGE_LOOP('',(#32773,#32774,#32775,#32776)) ;
#14236=EDGE_LOOP('',(#32777,#32778,#32779,#32780)) ;
#14237=EDGE_LOOP('',(#32781,#32782,#32783,#32784)) ;
#14238=EDGE_LOOP('',(#32785,#32786,#32787,#32788,#32789,#32790,#32791,#32792,
#32793,#32794,#32795)) ;
#14239=EDGE_LOOP('',(#32796,#32797,#32798,#32799,#32800,#32801,#32802,#32803)) ;
#14240=EDGE_LOOP('',(#32804,#32805,#32806,#32807,#32808,#32809,#32810,#32811,
#32812,#32813)) ;
#14241=EDGE_LOOP('',(#32814,#32815,#32816,#32817)) ;
#14242=EDGE_LOOP('',(#32818,#32819,#32820,#32821,#32822,#32823)) ;
#14243=EDGE_LOOP('',(#32824,#32825,#32826,#32827)) ;
#14244=EDGE_LOOP('',(#32828,#32829,#32830)) ;
#14245=EDGE_LOOP('',(#32831,#32832,#32833,#32834)) ;
#14246=EDGE_LOOP('',(#32835,#32836,#32837,#32838)) ;
#14247=EDGE_LOOP('',(#32839,#32840,#32841,#32842)) ;
#14248=EDGE_LOOP('',(#32843,#32844,#32845)) ;
#14249=EDGE_LOOP('',(#32846,#32847,#32848,#32849)) ;
#14250=EDGE_LOOP('',(#32850,#32851,#32852)) ;
#14251=EDGE_LOOP('',(#32853,#32854,#32855,#32856)) ;
#14252=EDGE_LOOP('',(#32857,#32858,#32859,#32860)) ;
#14253=EDGE_LOOP('',(#32861,#32862,#32863,#32864)) ;
#14254=EDGE_LOOP('',(#32865,#32866,#32867,#32868,#32869)) ;
#14255=EDGE_LOOP('',(#32870,#32871,#32872,#32873)) ;
#14256=EDGE_LOOP('',(#32874,#32875,#32876,#32877)) ;
#14257=EDGE_LOOP('',(#32878,#32879,#32880,#32881)) ;
#14258=EDGE_LOOP('',(#32882,#32883,#32884,#32885)) ;
#14259=EDGE_LOOP('',(#32886,#32887,#32888,#32889)) ;
#14260=EDGE_LOOP('',(#32890,#32891,#32892,#32893)) ;
#14261=EDGE_LOOP('',(#32894,#32895,#32896,#32897)) ;
#14262=EDGE_LOOP('',(#32898,#32899,#32900,#32901)) ;
#14263=EDGE_LOOP('',(#32902,#32903,#32904,#32905)) ;
#14264=EDGE_LOOP('',(#32906,#32907,#32908,#32909)) ;
#14265=EDGE_LOOP('',(#32910,#32911,#32912,#32913)) ;
#14266=EDGE_LOOP('',(#32914,#32915,#32916,#32917)) ;
#14267=EDGE_LOOP('',(#32918,#32919,#32920,#32921)) ;
#14268=EDGE_LOOP('',(#32922,#32923,#32924,#32925)) ;
#14269=EDGE_LOOP('',(#32926,#32927,#32928,#32929)) ;
#14270=EDGE_LOOP('',(#32930,#32931,#32932,#32933)) ;
#14271=EDGE_LOOP('',(#32934,#32935,#32936,#32937)) ;
#14272=EDGE_LOOP('',(#32938,#32939,#32940,#32941)) ;
#14273=EDGE_LOOP('',(#32942,#32943,#32944,#32945,#32946)) ;
#14274=EDGE_LOOP('',(#32947,#32948,#32949,#32950)) ;
#14275=EDGE_LOOP('',(#32951,#32952,#32953,#32954,#32955)) ;
#14276=EDGE_LOOP('',(#32956,#32957,#32958,#32959)) ;
#14277=EDGE_LOOP('',(#32960,#32961,#32962,#32963)) ;
#14278=EDGE_LOOP('',(#32964,#32965,#32966,#32967)) ;
#14279=EDGE_LOOP('',(#32968,#32969,#32970,#32971)) ;
#14280=EDGE_LOOP('',(#32972,#32973,#32974,#32975)) ;
#14281=EDGE_LOOP('',(#32976,#32977,#32978,#32979)) ;
#14282=EDGE_LOOP('',(#32980,#32981,#32982,#32983)) ;
#14283=EDGE_LOOP('',(#32984,#32985,#32986,#32987)) ;
#14284=EDGE_LOOP('',(#32988,#32989,#32990,#32991)) ;
#14285=EDGE_LOOP('',(#32992,#32993,#32994,#32995)) ;
#14286=EDGE_LOOP('',(#32996,#32997,#32998,#32999)) ;
#14287=EDGE_LOOP('',(#33000,#33001,#33002,#33003)) ;
#14288=EDGE_LOOP('',(#33004,#33005,#33006,#33007)) ;
#14289=EDGE_LOOP('',(#33008,#33009,#33010,#33011)) ;
#14290=EDGE_LOOP('',(#33012,#33013,#33014,#33015,#33016,#33017)) ;
#14291=EDGE_LOOP('',(#33018,#33019,#33020,#33021,#33022)) ;
#14292=EDGE_LOOP('',(#33023,#33024,#33025,#33026)) ;
#14293=EDGE_LOOP('',(#33027,#33028,#33029,#33030)) ;
#14294=EDGE_LOOP('',(#33031,#33032,#33033,#33034)) ;
#14295=EDGE_LOOP('',(#33035,#33036,#33037,#33038)) ;
#14296=EDGE_LOOP('',(#33039,#33040,#33041,#33042)) ;
#14297=EDGE_LOOP('',(#33043,#33044,#33045,#33046)) ;
#14298=EDGE_LOOP('',(#33047,#33048,#33049,#33050)) ;
#14299=EDGE_LOOP('',(#33051,#33052,#33053,#33054)) ;
#14300=EDGE_LOOP('',(#33055,#33056,#33057,#33058)) ;
#14301=EDGE_LOOP('',(#33059,#33060,#33061,#33062)) ;
#14302=EDGE_LOOP('',(#33063,#33064,#33065,#33066)) ;
#14303=EDGE_LOOP('',(#33067,#33068,#33069,#33070,#33071,#33072,#33073,#33074,
#33075,#33076,#33077,#33078,#33079,#33080)) ;
#14304=EDGE_LOOP('',(#33081,#33082,#33083)) ;
#14305=EDGE_LOOP('',(#33084)) ;
#14306=EDGE_LOOP('',(#33085,#33086,#33087,#33088,#33089,#33090)) ;
#14307=EDGE_LOOP('',(#33091,#33092,#33093,#33094,#33095)) ;
#14308=EDGE_LOOP('',(#33096,#33097,#33098,#33099)) ;
#17349=CIRCLE('',#49867,0.119999999999978) ;
#17350=CIRCLE('',#49868,0.119999999999985) ;
#17351=CIRCLE('',#49869,0.420453920364715) ;
#17352=CIRCLE('',#49870,0.12) ;
#17353=CIRCLE('',#49871,0.300324228815928) ;
#17354=CIRCLE('',#49873,0.119999999999985) ;
#17355=CIRCLE('',#49875,0.12000000000001) ;
#17356=CIRCLE('',#49878,0.120000000000005) ;
#17357=CIRCLE('',#49880,0.120000000000011) ;
#17358=CIRCLE('',#49881,0.12) ;
#17359=CIRCLE('',#49882,0.120000000000005) ;
#17360=CIRCLE('',#49884,0.120000000000005) ;
#17361=CIRCLE('',#49886,0.120000000000023) ;
#17362=CIRCLE('',#49888,0.120000000000006) ;
#17363=CIRCLE('',#49889,0.12000000000004) ;
#17364=CIRCLE('',#49891,0.120000000000005) ;
#17365=CIRCLE('',#49897,3.48) ;
#17366=CIRCLE('',#49898,8.88713010990353) ;
#17367=CIRCLE('',#49902,33.1299448717372) ;
#17368=CIRCLE('',#49906,33.6004676577322) ;
#17369=CIRCLE('',#49907,3.48) ;
#17370=CIRCLE('',#49914,9.12754474878259) ;
#17371=CIRCLE('',#49915,3.48) ;
#17372=CIRCLE('',#49916,2.12) ;
#17373=CIRCLE('',#49918,0.12) ;
#17374=CIRCLE('',#49919,0.120000000000005) ;
#17375=CIRCLE('',#49921,0.119999999999995) ;
#17376=CIRCLE('',#49922,0.120000000000007) ;
#17377=CIRCLE('',#49923,0.119999999999985) ;
#17378=CIRCLE('',#49925,0.119999999999985) ;
#17379=CIRCLE('',#49926,0.11999999999998) ;
#17380=CIRCLE('',#49927,0.120000000000006) ;
#17381=CIRCLE('',#49931,0.12) ;
#17382=CIRCLE('',#49932,2.) ;
#17383=CIRCLE('',#49934,2.) ;
#17384=CIRCLE('',#49939,3.6) ;
#17385=CIRCLE('',#49941,0.12) ;
#17386=CIRCLE('',#49942,33.4983398799233) ;
#17387=CIRCLE('',#49943,0.12) ;
#17388=CIRCLE('',#49945,0.12) ;
#17389=CIRCLE('',#49947,0.12) ;
#17390=CIRCLE('',#49948,0.12) ;
#17391=CIRCLE('',#49949,0.12) ;
#17392=CIRCLE('',#49951,0.12) ;
#17393=CIRCLE('',#49952,0.12) ;
#17394=CIRCLE('',#49954,0.12) ;
#17395=CIRCLE('',#49955,0.12) ;
#17396=CIRCLE('',#49956,33.2502644468207) ;
#17397=CIRCLE('',#49957,0.12) ;
#17398=CIRCLE('',#49959,0.12) ;
#17399=CIRCLE('',#49961,0.12) ;
#17400=CIRCLE('',#49963,0.12) ;
#17401=CIRCLE('',#49964,9.00722646272021) ;
#17402=CIRCLE('',#49969,3.6) ;
#17403=CIRCLE('',#49971,33.2502644469926) ;
#17404=CIRCLE('',#49979,3.6) ;
#17405=CIRCLE('',#49982,3.6) ;
#17406=CIRCLE('',#49983,0.119999999999985) ;
#17407=CIRCLE('',#49984,0.12) ;
#17408=CIRCLE('',#49986,0.120000000000048) ;
#17409=CIRCLE('',#49987,0.119999999999985) ;
#17410=CIRCLE('',#49988,0.12) ;
#17411=CIRCLE('',#49989,0.119999999999999) ;
#17412=CIRCLE('',#49990,0.12) ;
#17413=CIRCLE('',#49992,0.119999999999985) ;
#17414=CIRCLE('',#49993,0.119999999999999) ;
#17415=CIRCLE('',#49994,0.119999999999999) ;
#17416=CIRCLE('',#49995,0.12) ;
#17417=CIRCLE('',#49996,0.120000000000005) ;
#17418=CIRCLE('',#49998,0.12) ;
#17419=CIRCLE('',#50005,0.119999999999992) ;
#17420=CIRCLE('',#50006,0.120000000000003) ;
#17421=CIRCLE('',#50010,0.12) ;
#17422=CIRCLE('',#50012,0.12) ;
#17423=CIRCLE('',#50013,9.00744547576183) ;
#17424=CIRCLE('',#50014,8.88734620275781) ;
#17425=CIRCLE('',#50018,0.120000000000011) ;
#17426=CIRCLE('',#50019,9.00744547576355) ;
#17427=CIRCLE('',#50020,0.120000000000005) ;
#17428=CIRCLE('',#50024,3.6) ;
#17429=CIRCLE('',#50028,0.11999999999999) ;
#17430=CIRCLE('',#50029,0.120000000000005) ;
#17431=CIRCLE('',#50030,0.120000000000003) ;
#17432=CIRCLE('',#50032,0.119999999999969) ;
#17433=CIRCLE('',#50035,0.120000000000005) ;
#17434=CIRCLE('',#50036,0.120000000000038) ;
#17435=CIRCLE('',#50038,0.119999999999997) ;
#17436=CIRCLE('',#50039,0.119999999999985) ;
#17437=CIRCLE('',#50042,0.120000000000006) ;
#17438=CIRCLE('',#50043,0.12) ;
#17439=CIRCLE('',#50044,0.120000000000007) ;
#17440=CIRCLE('',#50045,0.120000000000005) ;
#17441=CIRCLE('',#50048,0.120000000000005) ;
#17442=CIRCLE('',#50049,0.119999999999998) ;
#17443=CIRCLE('',#50050,0.120000000000008) ;
#17444=CIRCLE('',#50051,0.119999999999969) ;
#17445=CIRCLE('',#50057,0.120000000000005) ;
#17446=CIRCLE('',#50058,0.120000000000007) ;
#17447=CIRCLE('',#50059,0.12) ;
#17448=CIRCLE('',#50060,0.119999999999989) ;
#17449=CIRCLE('',#50062,0.12) ;
#17450=CIRCLE('',#50064,0.120000000000005) ;
#17451=CIRCLE('',#50065,0.12) ;
#17452=CIRCLE('',#50066,0.11999999999999) ;
#17453=CIRCLE('',#50067,0.120000000000005) ;
#17454=CIRCLE('',#50068,0.120000000000005) ;
#17455=CIRCLE('',#50070,0.12) ;
#17456=CIRCLE('',#50072,0.12) ;
#17457=CIRCLE('',#50075,0.12) ;
#17458=CIRCLE('',#50076,0.12) ;
#17459=CIRCLE('',#50078,0.120000000000005) ;
#17460=CIRCLE('',#50079,0.12) ;
#17461=CIRCLE('',#50080,0.120000000000002) ;
#17462=CIRCLE('',#50082,0.120000000000005) ;
#17463=CIRCLE('',#50085,0.120000000000005) ;
#17464=CIRCLE('',#50086,0.119999999999998) ;
#17465=CIRCLE('',#50092,33.129944871325) ;
#17466=CIRCLE('',#50096,0.120000000000005) ;
#17467=CIRCLE('',#50097,0.12) ;
#17468=CIRCLE('',#50099,0.120000000000001) ;
#17469=CIRCLE('',#50100,0.120000000000005) ;
#17470=CIRCLE('',#50101,0.12) ;
#17471=CIRCLE('',#50102,0.12) ;
#17472=CIRCLE('',#50104,0.12) ;
#17473=CIRCLE('',#50105,0.119999999999996) ;
#17474=CIRCLE('',#50106,0.12) ;
#17475=CIRCLE('',#50108,0.120000000000005) ;
#17476=CIRCLE('',#50109,0.12) ;
#17477=CIRCLE('',#50110,0.12) ;
#17478=CIRCLE('',#50112,0.119999999999996) ;
#17479=CIRCLE('',#50113,0.12) ;
#17480=CIRCLE('',#50114,0.119999999999985) ;
#17481=CIRCLE('',#50115,0.119999999999985) ;
#17482=CIRCLE('',#50116,0.12) ;
#17483=CIRCLE('',#50118,0.120000000000003) ;
#17484=CIRCLE('',#50119,0.120000000000021) ;
#17485=CIRCLE('',#50120,0.120000000000021) ;
#17486=CIRCLE('',#50121,0.12) ;
#17487=CIRCLE('',#50131,33.4983398800573) ;
#17488=CIRCLE('',#50132,0.120000000000003) ;
#17489=CIRCLE('',#50137,0.119999999999997) ;
#17490=CIRCLE('',#50138,0.119999999999985) ;
#17491=CIRCLE('',#50139,0.119999999999985) ;
#17492=CIRCLE('',#50140,0.12) ;
#17493=CIRCLE('',#50141,0.12) ;
#17494=CIRCLE('',#50142,0.12) ;
#17495=CIRCLE('',#50143,0.12) ;
#17496=CIRCLE('',#50144,0.12) ;
#17497=CIRCLE('',#50145,0.12) ;
#17498=CIRCLE('',#50148,0.12) ;
#17499=CIRCLE('',#50149,0.12) ;
#17500=CIRCLE('',#50150,0.12) ;
#17501=CIRCLE('',#50151,0.12) ;
#17502=CIRCLE('',#50152,0.12) ;
#17503=CIRCLE('',#50160,3.6) ;
#19895=VERTEX_POINT('',#75336) ;
#19896=VERTEX_POINT('',#75337) ;
#19897=VERTEX_POINT('',#75339) ;
#19898=VERTEX_POINT('',#75344) ;
#19899=VERTEX_POINT('',#75377) ;
#19900=VERTEX_POINT('',#75378) ;
#19901=VERTEX_POINT('',#75380) ;
#19902=VERTEX_POINT('',#75382) ;
#19903=VERTEX_POINT('',#75386) ;
#19904=VERTEX_POINT('',#75387) ;
#19905=VERTEX_POINT('',#75426) ;
#19906=VERTEX_POINT('',#75427) ;
#19907=VERTEX_POINT('',#75499) ;
#19908=VERTEX_POINT('',#75501) ;
#19909=VERTEX_POINT('',#75514) ;
#19910=VERTEX_POINT('',#75537) ;
#19911=VERTEX_POINT('',#75560) ;
#19912=VERTEX_POINT('',#75562) ;
#19913=VERTEX_POINT('',#75585) ;
#19914=VERTEX_POINT('',#75586) ;
#19915=VERTEX_POINT('',#75588) ;
#19916=VERTEX_POINT('',#75593) ;
#19917=VERTEX_POINT('',#75629) ;
#19918=VERTEX_POINT('',#75636) ;
#19919=VERTEX_POINT('',#75645) ;
#19920=VERTEX_POINT('',#75646) ;
#19921=VERTEX_POINT('',#75670) ;
#19922=VERTEX_POINT('',#75672) ;
#19923=VERTEX_POINT('',#75695) ;
#19924=VERTEX_POINT('',#75696) ;
#19925=VERTEX_POINT('',#75736) ;
#19926=VERTEX_POINT('',#75743) ;
#19927=VERTEX_POINT('',#75752) ;
#19928=VERTEX_POINT('',#75753) ;
#19929=VERTEX_POINT('',#75787) ;
#19930=VERTEX_POINT('',#75789) ;
#19931=VERTEX_POINT('',#75793) ;
#19932=VERTEX_POINT('',#75810) ;
#19933=VERTEX_POINT('',#75827) ;
#19934=VERTEX_POINT('',#75834) ;
#19935=VERTEX_POINT('',#75835) ;
#19936=VERTEX_POINT('',#75837) ;
#19937=VERTEX_POINT('',#75839) ;
#19938=VERTEX_POINT('',#75841) ;
#19939=VERTEX_POINT('',#75843) ;
#19940=VERTEX_POINT('',#75845) ;
#19941=VERTEX_POINT('',#75847) ;
#19942=VERTEX_POINT('',#75849) ;
#19943=VERTEX_POINT('',#75851) ;
#19944=VERTEX_POINT('',#75853) ;
#19945=VERTEX_POINT('',#75859) ;
#19946=VERTEX_POINT('',#75861) ;
#19947=VERTEX_POINT('',#75863) ;
#19948=VERTEX_POINT('',#75871) ;
#19949=VERTEX_POINT('',#75877) ;
#19950=VERTEX_POINT('',#75883) ;
#19951=VERTEX_POINT('',#75885) ;
#19952=VERTEX_POINT('',#75887) ;
#19953=VERTEX_POINT('',#75889) ;
#19954=VERTEX_POINT('',#75892) ;
#19955=VERTEX_POINT('',#75893) ;
#19956=VERTEX_POINT('',#75895) ;
#19957=VERTEX_POINT('',#75897) ;
#19958=VERTEX_POINT('',#75899) ;
#19959=VERTEX_POINT('',#75906) ;
#19960=VERTEX_POINT('',#75908) ;
#19961=VERTEX_POINT('',#75914) ;
#19962=VERTEX_POINT('',#75922) ;
#19963=VERTEX_POINT('',#75923) ;
#19964=VERTEX_POINT('',#75930) ;
#19965=VERTEX_POINT('',#75932) ;
#19966=VERTEX_POINT('',#75934) ;
#19967=VERTEX_POINT('',#75942) ;
#19968=VERTEX_POINT('',#75944) ;
#19969=VERTEX_POINT('',#75950) ;
#19970=VERTEX_POINT('',#75952) ;
#19971=VERTEX_POINT('',#75954) ;
#19972=VERTEX_POINT('',#75956) ;
#19973=VERTEX_POINT('',#75959) ;
#19974=VERTEX_POINT('',#75962) ;
#19975=VERTEX_POINT('',#75964) ;
#19976=VERTEX_POINT('',#75987) ;
#19977=VERTEX_POINT('',#76010) ;
#19978=VERTEX_POINT('',#76046) ;
#19979=VERTEX_POINT('',#76055) ;
#19980=VERTEX_POINT('',#76083) ;
#19981=VERTEX_POINT('',#76110) ;
#19982=VERTEX_POINT('',#76164) ;
#19983=VERTEX_POINT('',#76166) ;
#19984=VERTEX_POINT('',#76182) ;
#19985=VERTEX_POINT('',#76196) ;
#19986=VERTEX_POINT('',#76200) ;
#19987=VERTEX_POINT('',#76204) ;
#19988=VERTEX_POINT('',#76208) ;
#19989=VERTEX_POINT('',#76212) ;
#19990=VERTEX_POINT('',#76214) ;
#19991=VERTEX_POINT('',#76218) ;
#19992=VERTEX_POINT('',#76237) ;
#19993=VERTEX_POINT('',#76273) ;
#19994=VERTEX_POINT('',#76296) ;
#19995=VERTEX_POINT('',#76319) ;
#19996=VERTEX_POINT('',#76347) ;
#19997=VERTEX_POINT('',#76383) ;
#19998=VERTEX_POINT('',#76430) ;
#19999=VERTEX_POINT('',#76440) ;
#20000=VERTEX_POINT('',#76463) ;
#20001=VERTEX_POINT('',#76491) ;
#20002=VERTEX_POINT('',#76523) ;
#20003=VERTEX_POINT('',#76546) ;
#20004=VERTEX_POINT('',#76569) ;
#20005=VERTEX_POINT('',#76592) ;
#20006=VERTEX_POINT('',#76615) ;
#20007=VERTEX_POINT('',#76619) ;
#20008=VERTEX_POINT('',#76623) ;
#20009=VERTEX_POINT('',#76672) ;
#20010=VERTEX_POINT('',#76674) ;
#20011=VERTEX_POINT('',#76682) ;
#20012=VERTEX_POINT('',#76705) ;
#20013=VERTEX_POINT('',#76720) ;
#20014=VERTEX_POINT('',#76722) ;
#20015=VERTEX_POINT('',#76725) ;
#20016=VERTEX_POINT('',#76758) ;
#20017=VERTEX_POINT('',#76769) ;
#20018=VERTEX_POINT('',#76778) ;
#20019=VERTEX_POINT('',#76782) ;
#20020=VERTEX_POINT('',#76786) ;
#20021=VERTEX_POINT('',#76790) ;
#20022=VERTEX_POINT('',#76794) ;
#20023=VERTEX_POINT('',#76809) ;
#20024=VERTEX_POINT('',#76850) ;
#20025=VERTEX_POINT('',#76852) ;
#20026=VERTEX_POINT('',#76860) ;
#20027=VERTEX_POINT('',#76861) ;
#20028=VERTEX_POINT('',#76863) ;
#20029=VERTEX_POINT('',#76913) ;
#20030=VERTEX_POINT('',#76915) ;
#20031=VERTEX_POINT('',#76924) ;
#20032=VERTEX_POINT('',#76925) ;
#20033=VERTEX_POINT('',#76927) ;
#20034=VERTEX_POINT('',#76929) ;
#20035=VERTEX_POINT('',#76966) ;
#20036=VERTEX_POINT('',#76967) ;
#20037=VERTEX_POINT('',#76969) ;
#20038=VERTEX_POINT('',#76971) ;
#20039=VERTEX_POINT('',#77036) ;
#20040=VERTEX_POINT('',#77037) ;
#20041=VERTEX_POINT('',#77074) ;
#20042=VERTEX_POINT('',#77118) ;
#20043=VERTEX_POINT('',#77120) ;
#20044=VERTEX_POINT('',#77143) ;
#20045=VERTEX_POINT('',#77144) ;
#20046=VERTEX_POINT('',#77149) ;
#20047=VERTEX_POINT('',#77150) ;
#20048=VERTEX_POINT('',#77185) ;
#20049=VERTEX_POINT('',#77208) ;
#20050=VERTEX_POINT('',#77233) ;
#20051=VERTEX_POINT('',#77248) ;
#20052=VERTEX_POINT('',#77250) ;
#20053=VERTEX_POINT('',#77272) ;
#20054=VERTEX_POINT('',#77274) ;
#20055=VERTEX_POINT('',#77303) ;
#20056=VERTEX_POINT('',#77305) ;
#20057=VERTEX_POINT('',#77332) ;
#20058=VERTEX_POINT('',#77355) ;
#20059=VERTEX_POINT('',#77359) ;
#20060=VERTEX_POINT('',#77392) ;
#20061=VERTEX_POINT('',#77393) ;
#20062=VERTEX_POINT('',#77427) ;
#20063=VERTEX_POINT('',#77429) ;
#20064=VERTEX_POINT('',#77460) ;
#20065=VERTEX_POINT('',#77461) ;
#20066=VERTEX_POINT('',#77507) ;
#20067=VERTEX_POINT('',#77508) ;
#20068=VERTEX_POINT('',#77510) ;
#20069=VERTEX_POINT('',#77517) ;
#20070=VERTEX_POINT('',#77549) ;
#20071=VERTEX_POINT('',#77575) ;
#20072=VERTEX_POINT('',#77579) ;
#20073=VERTEX_POINT('',#77617) ;
#20074=VERTEX_POINT('',#77646) ;
#20075=VERTEX_POINT('',#77672) ;
#20076=VERTEX_POINT('',#77673) ;
#20077=VERTEX_POINT('',#77710) ;
#20078=VERTEX_POINT('',#77711) ;
#20079=VERTEX_POINT('',#77713) ;
#20080=VERTEX_POINT('',#77741) ;
#20081=VERTEX_POINT('',#77742) ;
#20082=VERTEX_POINT('',#77744) ;
#20083=VERTEX_POINT('',#77746) ;
#20084=VERTEX_POINT('',#77764) ;
#20085=VERTEX_POINT('',#77765) ;
#20086=VERTEX_POINT('',#77767) ;
#20087=VERTEX_POINT('',#77769) ;
#20088=VERTEX_POINT('',#77771) ;
#20089=VERTEX_POINT('',#77797) ;
#20090=VERTEX_POINT('',#77802) ;
#20091=VERTEX_POINT('',#77831) ;
#20092=VERTEX_POINT('',#77833) ;
#20093=VERTEX_POINT('',#77837) ;
#20094=VERTEX_POINT('',#77838) ;
#20095=VERTEX_POINT('',#77877) ;
#20096=VERTEX_POINT('',#77885) ;
#20097=VERTEX_POINT('',#77957) ;
#20098=VERTEX_POINT('',#77958) ;
#20099=VERTEX_POINT('',#77960) ;
#20100=VERTEX_POINT('',#77967) ;
#20101=VERTEX_POINT('',#77969) ;
#20102=VERTEX_POINT('',#77977) ;
#20103=VERTEX_POINT('',#78020) ;
#20104=VERTEX_POINT('',#78025) ;
#20105=VERTEX_POINT('',#78051) ;
#20106=VERTEX_POINT('',#78053) ;
#20107=VERTEX_POINT('',#78057) ;
#20108=VERTEX_POINT('',#78058) ;
#20109=VERTEX_POINT('',#78092) ;
#20110=VERTEX_POINT('',#78099) ;
#20111=VERTEX_POINT('',#78180) ;
#20112=VERTEX_POINT('',#78181) ;
#20113=VERTEX_POINT('',#78183) ;
#20114=VERTEX_POINT('',#78185) ;
#20115=VERTEX_POINT('',#78191) ;
#20116=VERTEX_POINT('',#78197) ;
#20117=VERTEX_POINT('',#78203) ;
#20118=VERTEX_POINT('',#78211) ;
#20119=VERTEX_POINT('',#78213) ;
#20120=VERTEX_POINT('',#78215) ;
#20121=VERTEX_POINT('',#78221) ;
#20122=VERTEX_POINT('',#78224) ;
#20123=VERTEX_POINT('',#78225) ;
#20124=VERTEX_POINT('',#78233) ;
#20125=VERTEX_POINT('',#78238) ;
#20126=VERTEX_POINT('',#78244) ;
#20127=VERTEX_POINT('',#78246) ;
#20128=VERTEX_POINT('',#78254) ;
#20129=VERTEX_POINT('',#78259) ;
#20130=VERTEX_POINT('',#78303) ;
#20131=VERTEX_POINT('',#78305) ;
#20132=VERTEX_POINT('',#78315) ;
#20133=VERTEX_POINT('',#78316) ;
#20134=VERTEX_POINT('',#78318) ;
#20135=VERTEX_POINT('',#78362) ;
#20136=VERTEX_POINT('',#78364) ;
#20137=VERTEX_POINT('',#78392) ;
#20138=VERTEX_POINT('',#78394) ;
#20139=VERTEX_POINT('',#78402) ;
#20140=VERTEX_POINT('',#78403) ;
#20141=VERTEX_POINT('',#78405) ;
#20142=VERTEX_POINT('',#78419) ;
#20143=VERTEX_POINT('',#78420) ;
#20144=VERTEX_POINT('',#78422) ;
#20145=VERTEX_POINT('',#78488) ;
#20146=VERTEX_POINT('',#78490) ;
#20147=VERTEX_POINT('',#78500) ;
#20148=VERTEX_POINT('',#78501) ;
#20149=VERTEX_POINT('',#78503) ;
#20150=VERTEX_POINT('',#78505) ;
#20151=VERTEX_POINT('',#78676) ;
#20152=VERTEX_POINT('',#78677) ;
#20153=VERTEX_POINT('',#78690) ;
#20154=VERTEX_POINT('',#78692) ;
#20155=VERTEX_POINT('',#78767) ;
#20156=VERTEX_POINT('',#78772) ;
#20157=VERTEX_POINT('',#78897) ;
#20158=VERTEX_POINT('',#78901) ;
#20159=VERTEX_POINT('',#78939) ;
#20160=VERTEX_POINT('',#78973) ;
#20161=VERTEX_POINT('',#79101) ;
#24365=EDGE_CURVE('',#19895,#19896,#17349,.T.) ;
#24366=EDGE_CURVE('',#19896,#19897,#895,.T.) ;
#24367=EDGE_CURVE('',#19897,#19898,#896,.T.) ;
#24368=EDGE_CURVE('',#19898,#19895,#897,.T.) ;
#24369=EDGE_CURVE('',#19899,#19900,#17350,.T.) ;
#24370=EDGE_CURVE('',#19900,#19901,#17351,.T.) ;
#24371=EDGE_CURVE('',#19901,#19902,#17352,.T.) ;
#24372=EDGE_CURVE('',#19902,#19899,#17353,.T.) ;
#24373=EDGE_CURVE('',#19903,#19904,#17354,.T.) ;
#24374=EDGE_CURVE('',#19904,#19900,#3186,.T.) ;
#24375=EDGE_CURVE('',#19899,#19903,#3187,.T.) ;
#24376=EDGE_CURVE('',#19905,#19906,#898,.T.) ;
#24377=EDGE_CURVE('',#19906,#19904,#899,.T.) ;
#24378=EDGE_CURVE('',#19903,#19905,#900,.T.) ;
#24379=EDGE_CURVE('',#19901,#19896,#901,.T.) ;
#24380=EDGE_CURVE('',#19895,#19902,#902,.T.) ;
#24381=EDGE_CURVE('',#19907,#19899,#3188,.T.) ;
#24382=EDGE_CURVE('',#19908,#19907,#3189,.T.) ;
#24383=EDGE_CURVE('',#19903,#19908,#3190,.T.) ;
#24384=EDGE_CURVE('',#19898,#19909,#3191,.T.) ;
#24385=EDGE_CURVE('',#19907,#19909,#903,.T.) ;
#24386=EDGE_CURVE('',#19910,#19896,#17355,.T.) ;
#24387=EDGE_CURVE('',#19910,#19898,#103,.T.) ;
#24388=EDGE_CURVE('',#19901,#19911,#104,.T.) ;
#24389=EDGE_CURVE('',#19912,#19911,#17356,.T.) ;
#24390=EDGE_CURVE('',#19912,#19910,#105,.T.) ;
#24391=EDGE_CURVE('',#19913,#19914,#17357,.T.) ;
#24392=EDGE_CURVE('',#19914,#19915,#904,.T.) ;
#24393=EDGE_CURVE('',#19915,#19916,#17358,.T.) ;
#24394=EDGE_CURVE('',#19916,#19913,#905,.T.) ;
#24395=EDGE_CURVE('',#19913,#19917,#906,.T.) ;
#24396=EDGE_CURVE('',#19917,#19918,#17359,.T.) ;
#24397=EDGE_CURVE('',#19918,#19914,#907,.T.) ;
#24398=EDGE_CURVE('',#19919,#19920,#17360,.T.) ;
#24399=EDGE_CURVE('',#19920,#19918,#3192,.T.) ;
#24400=EDGE_CURVE('',#19917,#19919,#3193,.T.) ;
#24401=EDGE_CURVE('',#19919,#19921,#106,.T.) ;
#24402=EDGE_CURVE('',#19921,#19922,#17361,.T.) ;
#24403=EDGE_CURVE('',#19922,#19920,#107,.T.) ;
#24404=EDGE_CURVE('',#19923,#19924,#17362,.T.) ;
#24405=EDGE_CURVE('',#19924,#19922,#908,.T.) ;
#24406=EDGE_CURVE('',#19921,#19923,#909,.T.) ;
#24407=EDGE_CURVE('',#19923,#19925,#910,.T.) ;
#24408=EDGE_CURVE('',#19925,#19926,#17363,.T.) ;
#24409=EDGE_CURVE('',#19926,#19924,#911,.T.) ;
#24410=EDGE_CURVE('',#19927,#19928,#17364,.T.) ;
#24411=EDGE_CURVE('',#19928,#19926,#3194,.T.) ;
#24412=EDGE_CURVE('',#19925,#19927,#3195,.T.) ;
#24413=EDGE_CURVE('',#19927,#19916,#108,.T.) ;
#24414=EDGE_CURVE('',#19915,#19928,#109,.T.) ;
#24415=EDGE_CURVE('',#19919,#19929,#3196,.T.) ;
#24416=EDGE_CURVE('',#19930,#19929,#110,.T.) ;
#24417=EDGE_CURVE('',#19930,#19921,#3197,.T.) ;
#24418=EDGE_CURVE('',#19931,#19917,#3198,.T.) ;
#24419=EDGE_CURVE('',#19929,#19931,#3199,.T.) ;
#24420=EDGE_CURVE('',#19913,#19932,#3200,.T.) ;
#24421=EDGE_CURVE('',#19931,#19932,#912,.T.) ;
#24422=EDGE_CURVE('',#19933,#19916,#3201,.T.) ;
#24423=EDGE_CURVE('',#19932,#19933,#913,.T.) ;
#24424=EDGE_CURVE('',#19934,#19935,#3202,.T.) ;
#24425=EDGE_CURVE('',#19936,#19934,#17365,.T.) ;
#24426=EDGE_CURVE('',#19937,#19936,#3203,.T.) ;
#24427=EDGE_CURVE('',#19938,#19937,#3204,.T.) ;
#24428=EDGE_CURVE('',#19939,#19938,#17366,.T.) ;
#24429=EDGE_CURVE('',#19940,#19939,#111,.T.) ;
#24430=EDGE_CURVE('',#19941,#19940,#112,.T.) ;
#24431=EDGE_CURVE('',#19942,#19941,#113,.T.) ;
#24432=EDGE_CURVE('',#19943,#19942,#17367,.T.) ;
#24433=EDGE_CURVE('',#19944,#19943,#914,.T.) ;
#24434=EDGE_CURVE('',#19945,#19944,#114,.T.) ;
#24435=EDGE_CURVE('',#19946,#19945,#3205,.T.) ;
#24436=EDGE_CURVE('',#19947,#19946,#915,.T.) ;
#24437=EDGE_CURVE('',#19948,#19947,#916,.T.) ;
#24438=EDGE_CURVE('',#19949,#19948,#917,.T.) ;
#24439=EDGE_CURVE('',#19950,#19949,#115,.T.) ;
#24440=EDGE_CURVE('',#19951,#19950,#116,.T.) ;
#24441=EDGE_CURVE('',#19952,#19951,#17368,.T.) ;
#24442=EDGE_CURVE('',#19953,#19952,#3206,.T.) ;
#24443=EDGE_CURVE('',#19935,#19953,#17369,.T.) ;
#24444=EDGE_CURVE('',#19954,#19955,#3207,.T.) ;
#24445=EDGE_CURVE('',#19956,#19954,#117,.T.) ;
#24446=EDGE_CURVE('',#19957,#19956,#118,.T.) ;
#24447=EDGE_CURVE('',#19958,#19957,#918,.T.) ;
#24448=EDGE_CURVE('',#19959,#19958,#3208,.T.) ;
#24449=EDGE_CURVE('',#19960,#19959,#919,.T.) ;
#24450=EDGE_CURVE('',#19961,#19960,#119,.T.) ;
#24451=EDGE_CURVE('',#19955,#19961,#920,.T.) ;
#24452=EDGE_CURVE('',#19962,#19963,#921,.T.) ;
#24453=EDGE_CURVE('',#19964,#19962,#120,.T.) ;
#24454=EDGE_CURVE('',#19965,#19964,#121,.T.) ;
#24455=EDGE_CURVE('',#19966,#19965,#922,.T.) ;
#24456=EDGE_CURVE('',#19967,#19966,#3209,.T.) ;
#24457=EDGE_CURVE('',#19968,#19967,#923,.T.) ;
#24458=EDGE_CURVE('',#19969,#19968,#122,.T.) ;
#24459=EDGE_CURVE('',#19970,#19969,#17370,.T.) ;
#24460=EDGE_CURVE('',#19971,#19970,#3210,.T.) ;
#24461=EDGE_CURVE('',#19972,#19971,#17371,.T.) ;
#24462=EDGE_CURVE('',#19963,#19972,#3211,.T.) ;
#24463=EDGE_CURVE('',#19973,#19973,#17372,.T.) ;
#24464=EDGE_CURVE('',#19955,#19974,#17373,.T.) ;
#24465=EDGE_CURVE('',#19974,#19975,#3212,.T.) ;
#24466=EDGE_CURVE('',#19975,#19954,#17374,.T.) ;
#24467=EDGE_CURVE('',#19975,#19976,#123,.T.) ;
#24468=EDGE_CURVE('',#19976,#19956,#17375,.T.) ;
#24469=EDGE_CURVE('',#19977,#19957,#17376,.T.) ;
#24470=EDGE_CURVE('',#19976,#19977,#924,.T.) ;
#24471=EDGE_CURVE('',#19977,#19978,#925,.T.) ;
#24472=EDGE_CURVE('',#19978,#19958,#17377,.T.) ;
#24473=EDGE_CURVE('',#19979,#19959,#17378,.T.) ;
#24474=EDGE_CURVE('',#19978,#19979,#3213,.T.) ;
#24475=EDGE_CURVE('',#19979,#19980,#926,.T.) ;
#24476=EDGE_CURVE('',#19980,#19960,#17379,.T.) ;
#24477=EDGE_CURVE('',#19981,#19961,#17380,.T.) ;
#24478=EDGE_CURVE('',#19980,#19981,#927,.T.) ;
#24479=EDGE_CURVE('',#19981,#19974,#928,.T.) ;
#24480=EDGE_CURVE('',#19977,#19982,#3214,.T.) ;
#24481=EDGE_CURVE('',#19983,#19982,#929,.T.) ;
#24482=EDGE_CURVE('',#19983,#19978,#3215,.T.) ;
#24483=EDGE_CURVE('',#19984,#19976,#3216,.T.) ;
#24484=EDGE_CURVE('',#19982,#19984,#930,.T.) ;
#24485=EDGE_CURVE('',#19975,#19985,#3217,.T.) ;
#24486=EDGE_CURVE('',#19984,#19985,#124,.T.) ;
#24487=EDGE_CURVE('',#19986,#19974,#3218,.T.) ;
#24488=EDGE_CURVE('',#19985,#19986,#3219,.T.) ;
#24489=EDGE_CURVE('',#19973,#19987,#17381,.T.) ;
#24490=EDGE_CURVE('',#19987,#19987,#17382,.T.) ;
#24491=EDGE_CURVE('',#19988,#19988,#17383,.T.) ;
#24492=EDGE_CURVE('',#19988,#19987,#3220,.T.) ;
#24493=EDGE_CURVE('',#19935,#19989,#125,.T.) ;
#24494=EDGE_CURVE('',#19989,#19990,#3221,.T.) ;
#24495=EDGE_CURVE('',#19934,#19990,#126,.T.) ;
#24496=EDGE_CURVE('',#19953,#19991,#931,.T.) ;
#24497=EDGE_CURVE('',#19991,#19989,#17384,.T.) ;
#24498=EDGE_CURVE('',#19952,#19992,#932,.T.) ;
#24499=EDGE_CURVE('',#19992,#19991,#3222,.T.) ;
#24500=EDGE_CURVE('',#19951,#19993,#17385,.T.) ;
#24501=EDGE_CURVE('',#19993,#19992,#17386,.T.) ;
#24502=EDGE_CURVE('',#19950,#19994,#17387,.T.) ;
#24503=EDGE_CURVE('',#19994,#19993,#127,.T.) ;
#24504=EDGE_CURVE('',#19949,#19995,#17388,.T.) ;
#24505=EDGE_CURVE('',#19995,#19994,#128,.T.) ;
#24506=EDGE_CURVE('',#19948,#19996,#17389,.T.) ;
#24507=EDGE_CURVE('',#19996,#19995,#933,.T.) ;
#24508=EDGE_CURVE('',#19947,#19997,#17390,.T.) ;
#24509=EDGE_CURVE('',#19997,#19996,#934,.T.) ;
#24510=EDGE_CURVE('',#19946,#19998,#17391,.T.) ;
#24511=EDGE_CURVE('',#19998,#19997,#935,.T.) ;
#24512=EDGE_CURVE('',#19945,#19999,#17392,.T.) ;
#24513=EDGE_CURVE('',#19999,#19998,#3223,.T.) ;
#24514=EDGE_CURVE('',#19944,#20000,#17393,.T.) ;
#24515=EDGE_CURVE('',#20000,#19999,#129,.T.) ;
#24516=EDGE_CURVE('',#19943,#20001,#17394,.T.) ;
#24517=EDGE_CURVE('',#20001,#20000,#936,.T.) ;
#24518=EDGE_CURVE('',#19942,#20002,#17395,.T.) ;
#24519=EDGE_CURVE('',#20002,#20001,#17396,.T.) ;
#24520=EDGE_CURVE('',#19941,#20003,#17397,.T.) ;
#24521=EDGE_CURVE('',#20003,#20002,#130,.T.) ;
#24522=EDGE_CURVE('',#19940,#20004,#17398,.T.) ;
#24523=EDGE_CURVE('',#20004,#20003,#131,.T.) ;
#24524=EDGE_CURVE('',#19939,#20005,#17399,.T.) ;
#24525=EDGE_CURVE('',#20005,#20004,#132,.T.) ;
#24526=EDGE_CURVE('',#19938,#20006,#17400,.T.) ;
#24527=EDGE_CURVE('',#20006,#20005,#17401,.T.) ;
#24528=EDGE_CURVE('',#20007,#20006,#3224,.T.) ;
#24529=EDGE_CURVE('',#19937,#20007,#133,.T.) ;
#24530=EDGE_CURVE('',#20008,#20007,#3225,.T.) ;
#24531=EDGE_CURVE('',#19936,#20008,#937,.T.) ;
#24532=EDGE_CURVE('',#19990,#20008,#17402,.T.) ;
#24533=EDGE_CURVE('',#20001,#20009,#3226,.T.) ;
#24534=EDGE_CURVE('',#20010,#20009,#938,.T.) ;
#24535=EDGE_CURVE('',#20000,#20010,#3227,.T.) ;
#24536=EDGE_CURVE('',#20011,#20002,#3228,.T.) ;
#24537=EDGE_CURVE('',#20009,#20011,#17403,.T.) ;
#24538=EDGE_CURVE('',#20012,#20003,#3229,.T.) ;
#24539=EDGE_CURVE('',#20011,#20012,#134,.T.) ;
#24540=EDGE_CURVE('',#20013,#20004,#3230,.T.) ;
#24541=EDGE_CURVE('',#20014,#20013,#135,.T.) ;
#24542=EDGE_CURVE('',#19905,#20014,#3231,.T.) ;
#24543=EDGE_CURVE('',#20015,#19905,#3232,.T.) ;
#24544=EDGE_CURVE('',#20012,#20015,#136,.T.) ;
#24545=EDGE_CURVE('',#20016,#20005,#3233,.T.) ;
#24546=EDGE_CURVE('',#20016,#19906,#137,.T.) ;
#24547=EDGE_CURVE('',#20006,#20017,#3234,.T.) ;
#24548=EDGE_CURVE('',#20017,#20016,#939,.T.) ;
#24549=EDGE_CURVE('',#20018,#20007,#3235,.T.) ;
#24550=EDGE_CURVE('',#20018,#20017,#3236,.T.) ;
#24551=EDGE_CURVE('',#20019,#20008,#3237,.T.) ;
#24552=EDGE_CURVE('',#20019,#20018,#3238,.T.) ;
#24553=EDGE_CURVE('',#20020,#19990,#3239,.T.) ;
#24554=EDGE_CURVE('',#20020,#20019,#17404,.T.) ;
#24555=EDGE_CURVE('',#20021,#19989,#3240,.T.) ;
#24556=EDGE_CURVE('',#20021,#20020,#3241,.T.) ;
#24557=EDGE_CURVE('',#19971,#20022,#940,.T.) ;
#24558=EDGE_CURVE('',#20022,#20023,#17405,.T.) ;
#24559=EDGE_CURVE('',#19972,#20023,#941,.T.) ;
#24560=EDGE_CURVE('',#20024,#19967,#17406,.T.) ;
#24561=EDGE_CURVE('',#20025,#20024,#942,.F.) ;
#24562=EDGE_CURVE('',#19968,#20025,#17407,.T.) ;
#24563=EDGE_CURVE('',#20026,#20027,#17408,.F.) ;
#24564=EDGE_CURVE('',#20028,#20026,#17409,.F.) ;
#24565=EDGE_CURVE('',#20027,#20028,#17410,.F.) ;
#24566=EDGE_CURVE('',#20024,#20028,#3242,.T.) ;
#24567=EDGE_CURVE('',#20026,#20025,#3243,.T.) ;
#24568=EDGE_CURVE('',#20029,#19965,#17411,.T.) ;
#24569=EDGE_CURVE('',#20030,#20029,#943,.F.) ;
#24570=EDGE_CURVE('',#19966,#20030,#17412,.T.) ;
#24571=EDGE_CURVE('',#20031,#20032,#17413,.F.) ;
#24572=EDGE_CURVE('',#20033,#20031,#17414,.F.) ;
#24573=EDGE_CURVE('',#20034,#20033,#17415,.F.) ;
#24574=EDGE_CURVE('',#20032,#20034,#17416,.F.) ;
#24575=EDGE_CURVE('',#20029,#20034,#3244,.T.) ;
#24576=EDGE_CURVE('',#20031,#20030,#3245,.T.) ;
#24577=EDGE_CURVE('',#20035,#20036,#17417,.T.) ;
#24578=EDGE_CURVE('',#20036,#20037,#138,.T.) ;
#24579=EDGE_CURVE('',#20037,#20038,#17418,.T.) ;
#24580=EDGE_CURVE('',#20038,#20035,#139,.T.) ;
#24581=EDGE_CURVE('',#20034,#20038,#140,.T.) ;
#24582=EDGE_CURVE('',#20037,#20032,#141,.T.) ;
#24583=EDGE_CURVE('',#20028,#20031,#3246,.T.) ;
#24584=EDGE_CURVE('',#20032,#20027,#3247,.T.) ;
#24585=EDGE_CURVE('',#20030,#20024,#3248,.T.) ;
#24586=EDGE_CURVE('',#20039,#20040,#142,.T.) ;
#24587=EDGE_CURVE('',#20040,#19962,#17419,.T.) ;
#24588=EDGE_CURVE('',#19963,#20039,#944,.T.) ;
#24589=EDGE_CURVE('',#20041,#19964,#17420,.T.) ;
#24590=EDGE_CURVE('',#20040,#20041,#143,.T.) ;
#24591=EDGE_CURVE('',#20041,#20029,#144,.T.) ;
#24592=EDGE_CURVE('',#20027,#20042,#145,.T.) ;
#24593=EDGE_CURVE('',#20042,#20043,#17421,.T.) ;
#24594=EDGE_CURVE('',#20043,#20026,#146,.T.) ;
#24595=EDGE_CURVE('',#20044,#20045,#17422,.T.) ;
#24596=EDGE_CURVE('',#20045,#20043,#17423,.T.) ;
#24597=EDGE_CURVE('',#20042,#20044,#17424,.T.) ;
#24598=EDGE_CURVE('',#20046,#20047,#945,.T.) ;
#24599=EDGE_CURVE('',#20046,#20045,#3249,.T.) ;
#24600=EDGE_CURVE('',#20044,#20047,#3250,.T.) ;
#24601=EDGE_CURVE('',#20023,#20039,#3251,.T.) ;
#24602=EDGE_CURVE('',#20025,#20048,#147,.T.) ;
#24603=EDGE_CURVE('',#20048,#19969,#17425,.T.) ;
#24604=EDGE_CURVE('',#20048,#20049,#17426,.T.) ;
#24605=EDGE_CURVE('',#20049,#19970,#17427,.T.) ;
#24606=EDGE_CURVE('',#20049,#20022,#3252,.T.) ;
#24607=EDGE_CURVE('',#20035,#20050,#946,.T.) ;
#24608=EDGE_CURVE('',#20050,#20036,#148,.T.) ;
#24609=EDGE_CURVE('',#20050,#20051,#3253,.T.) ;
#24610=EDGE_CURVE('',#20052,#20051,#3254,.T.) ;
#24611=EDGE_CURVE('',#20047,#20052,#17428,.T.) ;
#24612=EDGE_CURVE('',#20038,#20041,#3255,.T.) ;
#24613=EDGE_CURVE('',#20035,#20040,#3256,.T.) ;
#24614=EDGE_CURVE('',#20053,#20039,#3257,.T.) ;
#24615=EDGE_CURVE('',#20053,#20054,#149,.T.) ;
#24616=EDGE_CURVE('',#20054,#20035,#3258,.T.) ;
#24617=EDGE_CURVE('',#19982,#20055,#17429,.T.) ;
#24618=EDGE_CURVE('',#20055,#20056,#947,.T.) ;
#24619=EDGE_CURVE('',#20056,#19983,#17430,.T.) ;
#24620=EDGE_CURVE('',#19984,#20057,#17431,.T.) ;
#24621=EDGE_CURVE('',#20057,#20055,#150,.T.) ;
#24622=EDGE_CURVE('',#19985,#20058,#17432,.T.) ;
#24623=EDGE_CURVE('',#20058,#20057,#151,.T.) ;
#24624=EDGE_CURVE('',#19986,#20059,#17433,.T.) ;
#24625=EDGE_CURVE('',#20059,#20058,#3259,.T.) ;
#24626=EDGE_CURVE('',#20060,#20061,#17434,.T.) ;
#24627=EDGE_CURVE('',#20061,#20059,#948,.T.) ;
#24628=EDGE_CURVE('',#19986,#20060,#949,.T.) ;
#24629=EDGE_CURVE('',#20060,#20062,#152,.T.) ;
#24630=EDGE_CURVE('',#20062,#20063,#17435,.T.) ;
#24631=EDGE_CURVE('',#20063,#20061,#950,.T.) ;
#24632=EDGE_CURVE('',#20064,#20065,#17436,.T.) ;
#24633=EDGE_CURVE('',#20065,#20063,#951,.T.) ;
#24634=EDGE_CURVE('',#20062,#20064,#952,.T.) ;
#24635=EDGE_CURVE('',#20064,#19983,#3260,.T.) ;
#24636=EDGE_CURVE('',#20056,#20065,#3261,.T.) ;
#24637=EDGE_CURVE('',#20066,#20067,#17437,.T.) ;
#24638=EDGE_CURVE('',#20067,#20068,#953,.T.) ;
#24639=EDGE_CURVE('',#20068,#20069,#17438,.T.) ;
#24640=EDGE_CURVE('',#20069,#20066,#954,.T.) ;
#24641=EDGE_CURVE('',#20066,#19930,#955,.T.) ;
#24642=EDGE_CURVE('',#19930,#20070,#17439,.T.) ;
#24643=EDGE_CURVE('',#20070,#20067,#956,.T.) ;
#24644=EDGE_CURVE('',#19929,#20071,#17440,.T.) ;
#24645=EDGE_CURVE('',#20071,#20070,#153,.T.) ;
#24646=EDGE_CURVE('',#19931,#20072,#17441,.T.) ;
#24647=EDGE_CURVE('',#20072,#20071,#3262,.T.) ;
#24648=EDGE_CURVE('',#19932,#20073,#17442,.T.) ;
#24649=EDGE_CURVE('',#20073,#20072,#957,.T.) ;
#24650=EDGE_CURVE('',#19933,#20074,#17443,.T.) ;
#24651=EDGE_CURVE('',#20074,#20073,#958,.T.) ;
#24652=EDGE_CURVE('',#20075,#20076,#17444,.T.) ;
#24653=EDGE_CURVE('',#20076,#20074,#154,.T.) ;
#24654=EDGE_CURVE('',#19933,#20075,#155,.T.) ;
#24655=EDGE_CURVE('',#20075,#20069,#3263,.T.) ;
#24656=EDGE_CURVE('',#20068,#20076,#3264,.T.) ;
#24657=EDGE_CURVE('',#19923,#20066,#3265,.T.) ;
#24658=EDGE_CURVE('',#20069,#19925,#3266,.T.) ;
#24659=EDGE_CURVE('',#20077,#20078,#17445,.F.) ;
#24660=EDGE_CURVE('',#20079,#20077,#17446,.F.) ;
#24661=EDGE_CURVE('',#20078,#20079,#17447,.F.) ;
#24662=EDGE_CURVE('',#20080,#20081,#17448,.T.) ;
#24663=EDGE_CURVE('',#20082,#20080,#156,.F.) ;
#24664=EDGE_CURVE('',#20083,#20082,#17449,.T.) ;
#24665=EDGE_CURVE('',#20083,#20081,#959,.T.) ;
#24666=EDGE_CURVE('',#20080,#20079,#3267,.T.) ;
#24667=EDGE_CURVE('',#20077,#20082,#3268,.T.) ;
#24668=EDGE_CURVE('',#20084,#20085,#17450,.F.) ;
#24669=EDGE_CURVE('',#20086,#20084,#17451,.F.) ;
#24670=EDGE_CURVE('',#20087,#20086,#17452,.F.) ;
#24671=EDGE_CURVE('',#20088,#20087,#17453,.F.) ;
#24672=EDGE_CURVE('',#20085,#20088,#17454,.F.) ;
#24673=EDGE_CURVE('',#20084,#20077,#3269,.T.) ;
#24674=EDGE_CURVE('',#20078,#20086,#3270,.T.) ;
#24675=EDGE_CURVE('',#20086,#20089,#960,.T.) ;
#24676=EDGE_CURVE('',#20089,#20090,#17455,.T.) ;
#24677=EDGE_CURVE('',#20090,#20087,#961,.T.) ;
#24678=EDGE_CURVE('',#20089,#20091,#157,.T.) ;
#24679=EDGE_CURVE('',#20091,#20092,#17456,.T.) ;
#24680=EDGE_CURVE('',#20092,#20090,#158,.T.) ;
#24681=EDGE_CURVE('',#20093,#20094,#17457,.T.) ;
#24682=EDGE_CURVE('',#20094,#20092,#3271,.T.) ;
#24683=EDGE_CURVE('',#20091,#20093,#3272,.T.) ;
#24684=EDGE_CURVE('',#20093,#20095,#962,.T.) ;
#24685=EDGE_CURVE('',#20095,#20096,#17458,.T.) ;
#24686=EDGE_CURVE('',#20096,#20094,#963,.T.) ;
#24687=EDGE_CURVE('',#20079,#20096,#964,.T.) ;
#24688=EDGE_CURVE('',#20095,#20078,#965,.T.) ;
#24689=EDGE_CURVE('',#20097,#20098,#159,.T.) ;
#24690=EDGE_CURVE('',#20098,#20099,#966,.T.) ;
#24691=EDGE_CURVE('',#20100,#20099,#17459,.T.) ;
#24692=EDGE_CURVE('',#20101,#20100,#967,.F.) ;
#24693=EDGE_CURVE('',#20102,#20101,#17460,.T.) ;
#24694=EDGE_CURVE('',#20102,#20097,#968,.T.) ;
#24695=EDGE_CURVE('',#20087,#20101,#3273,.T.) ;
#24696=EDGE_CURVE('',#20100,#20084,#3274,.T.) ;
#24697=EDGE_CURVE('',#20101,#20103,#969,.T.) ;
#24698=EDGE_CURVE('',#20103,#20104,#17461,.T.) ;
#24699=EDGE_CURVE('',#20104,#20102,#970,.T.) ;
#24700=EDGE_CURVE('',#20103,#20105,#160,.T.) ;
#24701=EDGE_CURVE('',#20105,#20106,#17462,.T.) ;
#24702=EDGE_CURVE('',#20106,#20104,#161,.T.) ;
#24703=EDGE_CURVE('',#20107,#20108,#17463,.T.) ;
#24704=EDGE_CURVE('',#20108,#20106,#3275,.T.) ;
#24705=EDGE_CURVE('',#20105,#20107,#3276,.T.) ;
#24706=EDGE_CURVE('',#20107,#20109,#971,.T.) ;
#24707=EDGE_CURVE('',#20109,#20110,#17464,.T.) ;
#24708=EDGE_CURVE('',#20110,#20108,#972,.T.) ;
#24709=EDGE_CURVE('',#20081,#20110,#973,.T.) ;
#24710=EDGE_CURVE('',#20109,#20080,#974,.T.) ;
#24711=EDGE_CURVE('',#20099,#20083,#3277,.T.) ;
#24712=EDGE_CURVE('',#20082,#20100,#3278,.T.) ;
#24713=EDGE_CURVE('',#20107,#20094,#3279,.T.) ;
#24714=EDGE_CURVE('',#20096,#20109,#3280,.T.) ;
#24715=EDGE_CURVE('',#20103,#20090,#3281,.T.) ;
#24716=EDGE_CURVE('',#20092,#20105,#3282,.T.) ;
#24717=EDGE_CURVE('',#20111,#20112,#162,.T.) ;
#24718=EDGE_CURVE('',#20113,#20111,#3283,.T.) ;
#24719=EDGE_CURVE('',#20114,#20113,#975,.T.) ;
#24720=EDGE_CURVE('',#20115,#20114,#976,.T.) ;
#24721=EDGE_CURVE('',#20116,#20115,#977,.T.) ;
#24722=EDGE_CURVE('',#20117,#20116,#978,.T.) ;
#24723=EDGE_CURVE('',#20118,#20117,#3284,.T.) ;
#24724=EDGE_CURVE('',#20119,#20118,#163,.T.) ;
#24725=EDGE_CURVE('',#20120,#20119,#979,.T.) ;
#24726=EDGE_CURVE('',#20121,#20120,#17465,.T.) ;
#24727=EDGE_CURVE('',#20112,#20121,#164,.T.) ;
#24728=EDGE_CURVE('',#20122,#20123,#980,.T.) ;
#24729=EDGE_CURVE('',#20124,#20122,#981,.T.) ;
#24730=EDGE_CURVE('',#20125,#20124,#982,.T.) ;
#24731=EDGE_CURVE('',#20126,#20125,#3285,.T.) ;
#24732=EDGE_CURVE('',#20127,#20126,#983,.T.) ;
#24733=EDGE_CURVE('',#20128,#20127,#984,.T.) ;
#24734=EDGE_CURVE('',#20129,#20128,#985,.T.) ;
#24735=EDGE_CURVE('',#20123,#20129,#3286,.T.) ;
#24736=EDGE_CURVE('',#20130,#20126,#17466,.T.) ;
#24737=EDGE_CURVE('',#20131,#20130,#986,.F.) ;
#24738=EDGE_CURVE('',#20127,#20131,#17467,.T.) ;
#24739=EDGE_CURVE('',#20132,#20133,#17468,.F.) ;
#24740=EDGE_CURVE('',#20134,#20132,#17469,.F.) ;
#24741=EDGE_CURVE('',#20133,#20134,#17470,.F.) ;
#24742=EDGE_CURVE('',#20130,#20134,#3287,.T.) ;
#24743=EDGE_CURVE('',#20132,#20131,#3288,.T.) ;
#24744=EDGE_CURVE('',#20135,#20124,#17471,.T.) ;
#24745=EDGE_CURVE('',#20136,#20135,#165,.F.) ;
#24746=EDGE_CURVE('',#20125,#20136,#17472,.T.) ;
#24747=EDGE_CURVE('',#20137,#20128,#17473,.T.) ;
#24748=EDGE_CURVE('',#20138,#20137,#987,.F.) ;
#24749=EDGE_CURVE('',#20129,#20138,#17474,.T.) ;
#24750=EDGE_CURVE('',#20139,#20140,#17475,.F.) ;
#24751=EDGE_CURVE('',#20141,#20139,#17476,.F.) ;
#24752=EDGE_CURVE('',#20140,#20141,#17477,.F.) ;
#24753=EDGE_CURVE('',#20135,#20141,#3289,.T.) ;
#24754=EDGE_CURVE('',#20139,#20136,#3290,.T.) ;
#24755=EDGE_CURVE('',#20142,#20143,#17478,.F.) ;
#24756=EDGE_CURVE('',#20144,#20142,#17479,.F.) ;
#24757=EDGE_CURVE('',#20143,#20144,#17480,.F.) ;
#24758=EDGE_CURVE('',#20142,#20132,#988,.T.) ;
#24759=EDGE_CURVE('',#20133,#20144,#989,.T.) ;
#24760=EDGE_CURVE('',#20145,#20123,#17481,.T.) ;
#24761=EDGE_CURVE('',#20146,#20145,#990,.F.) ;
#24762=EDGE_CURVE('',#20122,#20146,#17482,.T.) ;
#24763=EDGE_CURVE('',#20147,#20148,#17483,.F.) ;
#24764=EDGE_CURVE('',#20149,#20147,#17484,.F.) ;
#24765=EDGE_CURVE('',#20150,#20149,#17485,.F.) ;
#24766=EDGE_CURVE('',#20148,#20150,#17486,.F.) ;
#24767=EDGE_CURVE('',#20145,#20150,#3291,.T.) ;
#24768=EDGE_CURVE('',#20147,#20146,#3292,.T.) ;
#24769=EDGE_CURVE('',#20150,#20143,#3293,.T.) ;
#24770=EDGE_CURVE('',#20144,#20148,#3294,.T.) ;
#24771=EDGE_CURVE('',#20141,#20147,#991,.T.) ;
#24772=EDGE_CURVE('',#20148,#20140,#166,.T.) ;
#24773=EDGE_CURVE('',#20146,#20135,#167,.T.) ;
#24774=EDGE_CURVE('',#20138,#20145,#3295,.T.) ;
#24775=EDGE_CURVE('',#20143,#20138,#3296,.T.) ;
#24776=EDGE_CURVE('',#20137,#20142,#3297,.T.) ;
#24777=EDGE_CURVE('',#20134,#20139,#3298,.T.) ;
#24778=EDGE_CURVE('',#20140,#20133,#3299,.T.) ;
#24779=EDGE_CURVE('',#20131,#20137,#992,.T.) ;
#24780=EDGE_CURVE('',#20136,#20130,#3300,.T.) ;
#24781=EDGE_CURVE('',#20151,#20152,#993,.T.) ;
#24782=EDGE_CURVE('',#20152,#20153,#17487,.T.) ;
#24783=EDGE_CURVE('',#20153,#20154,#17488,.T.) ;
#24784=EDGE_CURVE('',#20154,#20151,#994,.T.) ;
#24785=EDGE_CURVE('',#19911,#20154,#168,.T.) ;
#24786=EDGE_CURVE('',#20153,#19912,#169,.T.) ;
#24787=EDGE_CURVE('',#19910,#19995,#3301,.T.) ;
#24788=EDGE_CURVE('',#19912,#19994,#3302,.T.) ;
#24789=EDGE_CURVE('',#20153,#19993,#3303,.T.) ;
#24790=EDGE_CURVE('',#20152,#19992,#3304,.T.) ;
#24791=EDGE_CURVE('',#20155,#20151,#3305,.T.) ;
#24792=EDGE_CURVE('',#20155,#19991,#3306,.T.) ;
#24793=EDGE_CURVE('',#20015,#20111,#17489,.F.) ;
#24794=EDGE_CURVE('',#20156,#20015,#17490,.F.) ;
#24795=EDGE_CURVE('',#19908,#20156,#17491,.F.) ;
#24796=EDGE_CURVE('',#20111,#19908,#17492,.F.) ;
#24797=EDGE_CURVE('',#20112,#20012,#17493,.T.) ;
#24798=EDGE_CURVE('',#20121,#20011,#17494,.T.) ;
#24799=EDGE_CURVE('',#20120,#20009,#17495,.T.) ;
#24800=EDGE_CURVE('',#20119,#20010,#17496,.T.) ;
#24801=EDGE_CURVE('',#20118,#20157,#17497,.T.) ;
#24802=EDGE_CURVE('',#20157,#20010,#170,.T.) ;
#24803=EDGE_CURVE('',#20117,#20158,#17498,.T.) ;
#24804=EDGE_CURVE('',#20158,#20157,#3307,.T.) ;
#24805=EDGE_CURVE('',#20116,#20159,#17499,.T.) ;
#24806=EDGE_CURVE('',#20159,#20158,#995,.T.) ;
#24807=EDGE_CURVE('',#20115,#20160,#17500,.T.) ;
#24808=EDGE_CURVE('',#20160,#20159,#996,.T.) ;
#24809=EDGE_CURVE('',#20114,#19909,#17501,.T.) ;
#24810=EDGE_CURVE('',#19909,#20160,#997,.T.) ;
#24811=EDGE_CURVE('',#20113,#19907,#17502,.T.) ;
#24812=EDGE_CURVE('',#20157,#19999,#3308,.T.) ;
#24813=EDGE_CURVE('',#19998,#20158,#3309,.T.) ;
#24814=EDGE_CURVE('',#20159,#19997,#3310,.T.) ;
#24815=EDGE_CURVE('',#20160,#19996,#3311,.T.) ;
#24816=EDGE_CURVE('',#20054,#20161,#3312,.T.) ;
#24817=EDGE_CURVE('',#20051,#20161,#3313,.T.) ;
#24818=EDGE_CURVE('',#20048,#20043,#3314,.T.) ;
#24819=EDGE_CURVE('',#20045,#20049,#3315,.T.) ;
#24820=EDGE_CURVE('',#19979,#20064,#3316,.T.) ;
#24821=EDGE_CURVE('',#20062,#19980,#3317,.T.) ;
#24822=EDGE_CURVE('',#19981,#20060,#3318,.T.) ;
#24823=EDGE_CURVE('',#19927,#20075,#3319,.T.) ;
#24824=EDGE_CURVE('',#20046,#20022,#3320,.T.) ;
#24825=EDGE_CURVE('',#20155,#20021,#17503,.T.) ;
#24826=EDGE_CURVE('',#20053,#20161,#3321,.T.) ;
#24827=EDGE_CURVE('',#20052,#20023,#3322,.T.) ;
#32174=ORIENTED_EDGE('',*,*,#24365,.T.) ;
#32175=ORIENTED_EDGE('',*,*,#24366,.T.) ;
#32176=ORIENTED_EDGE('',*,*,#24367,.T.) ;
#32177=ORIENTED_EDGE('',*,*,#24368,.T.) ;
#32178=ORIENTED_EDGE('',*,*,#24369,.T.) ;
#32179=ORIENTED_EDGE('',*,*,#24370,.T.) ;
#32180=ORIENTED_EDGE('',*,*,#24371,.T.) ;
#32181=ORIENTED_EDGE('',*,*,#24372,.T.) ;
#32182=ORIENTED_EDGE('',*,*,#24373,.T.) ;
#32183=ORIENTED_EDGE('',*,*,#24374,.T.) ;
#32184=ORIENTED_EDGE('',*,*,#24369,.F.) ;
#32185=ORIENTED_EDGE('',*,*,#24375,.T.) ;
#32186=ORIENTED_EDGE('',*,*,#24376,.T.) ;
#32187=ORIENTED_EDGE('',*,*,#24377,.T.) ;
#32188=ORIENTED_EDGE('',*,*,#24373,.F.) ;
#32189=ORIENTED_EDGE('',*,*,#24378,.T.) ;
#32190=ORIENTED_EDGE('',*,*,#24371,.F.) ;
#32191=ORIENTED_EDGE('',*,*,#24379,.T.) ;
#32192=ORIENTED_EDGE('',*,*,#24365,.F.) ;
#32193=ORIENTED_EDGE('',*,*,#24380,.T.) ;
#32194=ORIENTED_EDGE('',*,*,#24375,.F.) ;
#32195=ORIENTED_EDGE('',*,*,#24381,.F.) ;
#32196=ORIENTED_EDGE('',*,*,#24382,.F.) ;
#32197=ORIENTED_EDGE('',*,*,#24383,.F.) ;
#32198=ORIENTED_EDGE('',*,*,#24372,.F.) ;
#32199=ORIENTED_EDGE('',*,*,#24380,.F.) ;
#32200=ORIENTED_EDGE('',*,*,#24368,.F.) ;
#32201=ORIENTED_EDGE('',*,*,#24384,.T.) ;
#32202=ORIENTED_EDGE('',*,*,#24385,.F.) ;
#32203=ORIENTED_EDGE('',*,*,#24381,.T.) ;
#32204=ORIENTED_EDGE('',*,*,#24366,.F.) ;
#32205=ORIENTED_EDGE('',*,*,#24386,.F.) ;
#32206=ORIENTED_EDGE('',*,*,#24387,.T.) ;
#32207=ORIENTED_EDGE('',*,*,#24367,.F.) ;
#32208=ORIENTED_EDGE('',*,*,#24379,.F.) ;
#32209=ORIENTED_EDGE('',*,*,#24388,.T.) ;
#32210=ORIENTED_EDGE('',*,*,#24389,.F.) ;
#32211=ORIENTED_EDGE('',*,*,#24390,.T.) ;
#32212=ORIENTED_EDGE('',*,*,#24386,.T.) ;
#32213=ORIENTED_EDGE('',*,*,#24391,.T.) ;
#32214=ORIENTED_EDGE('',*,*,#24392,.T.) ;
#32215=ORIENTED_EDGE('',*,*,#24393,.T.) ;
#32216=ORIENTED_EDGE('',*,*,#24394,.T.) ;
#32217=ORIENTED_EDGE('',*,*,#24391,.F.) ;
#32218=ORIENTED_EDGE('',*,*,#24395,.T.) ;
#32219=ORIENTED_EDGE('',*,*,#24396,.T.) ;
#32220=ORIENTED_EDGE('',*,*,#24397,.T.) ;
#32221=ORIENTED_EDGE('',*,*,#24398,.T.) ;
#32222=ORIENTED_EDGE('',*,*,#24399,.T.) ;
#32223=ORIENTED_EDGE('',*,*,#24396,.F.) ;
#32224=ORIENTED_EDGE('',*,*,#24400,.T.) ;
#32225=ORIENTED_EDGE('',*,*,#24398,.F.) ;
#32226=ORIENTED_EDGE('',*,*,#24401,.T.) ;
#32227=ORIENTED_EDGE('',*,*,#24402,.T.) ;
#32228=ORIENTED_EDGE('',*,*,#24403,.T.) ;
#32229=ORIENTED_EDGE('',*,*,#24404,.T.) ;
#32230=ORIENTED_EDGE('',*,*,#24405,.T.) ;
#32231=ORIENTED_EDGE('',*,*,#24402,.F.) ;
#32232=ORIENTED_EDGE('',*,*,#24406,.T.) ;
#32233=ORIENTED_EDGE('',*,*,#24404,.F.) ;
#32234=ORIENTED_EDGE('',*,*,#24407,.T.) ;
#32235=ORIENTED_EDGE('',*,*,#24408,.T.) ;
#32236=ORIENTED_EDGE('',*,*,#24409,.T.) ;
#32237=ORIENTED_EDGE('',*,*,#24410,.T.) ;
#32238=ORIENTED_EDGE('',*,*,#24411,.T.) ;
#32239=ORIENTED_EDGE('',*,*,#24408,.F.) ;
#32240=ORIENTED_EDGE('',*,*,#24412,.T.) ;
#32241=ORIENTED_EDGE('',*,*,#24410,.F.) ;
#32242=ORIENTED_EDGE('',*,*,#24413,.T.) ;
#32243=ORIENTED_EDGE('',*,*,#24393,.F.) ;
#32244=ORIENTED_EDGE('',*,*,#24414,.T.) ;
#32245=ORIENTED_EDGE('',*,*,#24401,.F.) ;
#32246=ORIENTED_EDGE('',*,*,#24415,.T.) ;
#32247=ORIENTED_EDGE('',*,*,#24416,.F.) ;
#32248=ORIENTED_EDGE('',*,*,#24417,.T.) ;
#32249=ORIENTED_EDGE('',*,*,#24400,.F.) ;
#32250=ORIENTED_EDGE('',*,*,#24418,.F.) ;
#32251=ORIENTED_EDGE('',*,*,#24419,.F.) ;
#32252=ORIENTED_EDGE('',*,*,#24415,.F.) ;
#32253=ORIENTED_EDGE('',*,*,#24395,.F.) ;
#32254=ORIENTED_EDGE('',*,*,#24420,.T.) ;
#32255=ORIENTED_EDGE('',*,*,#24421,.F.) ;
#32256=ORIENTED_EDGE('',*,*,#24418,.T.) ;
#32257=ORIENTED_EDGE('',*,*,#24394,.F.) ;
#32258=ORIENTED_EDGE('',*,*,#24422,.F.) ;
#32259=ORIENTED_EDGE('',*,*,#24423,.F.) ;
#32260=ORIENTED_EDGE('',*,*,#24420,.F.) ;
#32261=ORIENTED_EDGE('',*,*,#24424,.F.) ;
#32262=ORIENTED_EDGE('',*,*,#24425,.F.) ;
#32263=ORIENTED_EDGE('',*,*,#24426,.F.) ;
#32264=ORIENTED_EDGE('',*,*,#24427,.F.) ;
#32265=ORIENTED_EDGE('',*,*,#24428,.F.) ;
#32266=ORIENTED_EDGE('',*,*,#24429,.F.) ;
#32267=ORIENTED_EDGE('',*,*,#24430,.F.) ;
#32268=ORIENTED_EDGE('',*,*,#24431,.F.) ;
#32269=ORIENTED_EDGE('',*,*,#24432,.F.) ;
#32270=ORIENTED_EDGE('',*,*,#24433,.F.) ;
#32271=ORIENTED_EDGE('',*,*,#24434,.F.) ;
#32272=ORIENTED_EDGE('',*,*,#24435,.F.) ;
#32273=ORIENTED_EDGE('',*,*,#24436,.F.) ;
#32274=ORIENTED_EDGE('',*,*,#24437,.F.) ;
#32275=ORIENTED_EDGE('',*,*,#24438,.F.) ;
#32276=ORIENTED_EDGE('',*,*,#24439,.F.) ;
#32277=ORIENTED_EDGE('',*,*,#24440,.F.) ;
#32278=ORIENTED_EDGE('',*,*,#24441,.F.) ;
#32279=ORIENTED_EDGE('',*,*,#24442,.F.) ;
#32280=ORIENTED_EDGE('',*,*,#24443,.F.) ;
#32281=ORIENTED_EDGE('',*,*,#24444,.F.) ;
#32282=ORIENTED_EDGE('',*,*,#24445,.F.) ;
#32283=ORIENTED_EDGE('',*,*,#24446,.F.) ;
#32284=ORIENTED_EDGE('',*,*,#24447,.F.) ;
#32285=ORIENTED_EDGE('',*,*,#24448,.F.) ;
#32286=ORIENTED_EDGE('',*,*,#24449,.F.) ;
#32287=ORIENTED_EDGE('',*,*,#24450,.F.) ;
#32288=ORIENTED_EDGE('',*,*,#24451,.F.) ;
#32289=ORIENTED_EDGE('',*,*,#24452,.F.) ;
#32290=ORIENTED_EDGE('',*,*,#24453,.F.) ;
#32291=ORIENTED_EDGE('',*,*,#24454,.F.) ;
#32292=ORIENTED_EDGE('',*,*,#24455,.F.) ;
#32293=ORIENTED_EDGE('',*,*,#24456,.F.) ;
#32294=ORIENTED_EDGE('',*,*,#24457,.F.) ;
#32295=ORIENTED_EDGE('',*,*,#24458,.F.) ;
#32296=ORIENTED_EDGE('',*,*,#24459,.F.) ;
#32297=ORIENTED_EDGE('',*,*,#24460,.F.) ;
#32298=ORIENTED_EDGE('',*,*,#24461,.F.) ;
#32299=ORIENTED_EDGE('',*,*,#24462,.F.) ;
#32300=ORIENTED_EDGE('',*,*,#24463,.F.) ;
#32301=ORIENTED_EDGE('',*,*,#24392,.F.) ;
#32302=ORIENTED_EDGE('',*,*,#24397,.F.) ;
#32303=ORIENTED_EDGE('',*,*,#24399,.F.) ;
#32304=ORIENTED_EDGE('',*,*,#24403,.F.) ;
#32305=ORIENTED_EDGE('',*,*,#24405,.F.) ;
#32306=ORIENTED_EDGE('',*,*,#24409,.F.) ;
#32307=ORIENTED_EDGE('',*,*,#24411,.F.) ;
#32308=ORIENTED_EDGE('',*,*,#24414,.F.) ;
#32309=ORIENTED_EDGE('',*,*,#24464,.T.) ;
#32310=ORIENTED_EDGE('',*,*,#24465,.T.) ;
#32311=ORIENTED_EDGE('',*,*,#24466,.T.) ;
#32312=ORIENTED_EDGE('',*,*,#24444,.T.) ;
#32313=ORIENTED_EDGE('',*,*,#24466,.F.) ;
#32314=ORIENTED_EDGE('',*,*,#24467,.T.) ;
#32315=ORIENTED_EDGE('',*,*,#24468,.T.) ;
#32316=ORIENTED_EDGE('',*,*,#24445,.T.) ;
#32317=ORIENTED_EDGE('',*,*,#24469,.T.) ;
#32318=ORIENTED_EDGE('',*,*,#24446,.T.) ;
#32319=ORIENTED_EDGE('',*,*,#24468,.F.) ;
#32320=ORIENTED_EDGE('',*,*,#24470,.T.) ;
#32321=ORIENTED_EDGE('',*,*,#24469,.F.) ;
#32322=ORIENTED_EDGE('',*,*,#24471,.T.) ;
#32323=ORIENTED_EDGE('',*,*,#24472,.T.) ;
#32324=ORIENTED_EDGE('',*,*,#24447,.T.) ;
#32325=ORIENTED_EDGE('',*,*,#24473,.T.) ;
#32326=ORIENTED_EDGE('',*,*,#24448,.T.) ;
#32327=ORIENTED_EDGE('',*,*,#24472,.F.) ;
#32328=ORIENTED_EDGE('',*,*,#24474,.T.) ;
#32329=ORIENTED_EDGE('',*,*,#24473,.F.) ;
#32330=ORIENTED_EDGE('',*,*,#24475,.T.) ;
#32331=ORIENTED_EDGE('',*,*,#24476,.T.) ;
#32332=ORIENTED_EDGE('',*,*,#24449,.T.) ;
#32333=ORIENTED_EDGE('',*,*,#24477,.T.) ;
#32334=ORIENTED_EDGE('',*,*,#24450,.T.) ;
#32335=ORIENTED_EDGE('',*,*,#24476,.F.) ;
#32336=ORIENTED_EDGE('',*,*,#24478,.T.) ;
#32337=ORIENTED_EDGE('',*,*,#24477,.F.) ;
#32338=ORIENTED_EDGE('',*,*,#24479,.T.) ;
#32339=ORIENTED_EDGE('',*,*,#24464,.F.) ;
#32340=ORIENTED_EDGE('',*,*,#24451,.T.) ;
#32341=ORIENTED_EDGE('',*,*,#24471,.F.) ;
#32342=ORIENTED_EDGE('',*,*,#24480,.T.) ;
#32343=ORIENTED_EDGE('',*,*,#24481,.F.) ;
#32344=ORIENTED_EDGE('',*,*,#24482,.T.) ;
#32345=ORIENTED_EDGE('',*,*,#24470,.F.) ;
#32346=ORIENTED_EDGE('',*,*,#24483,.F.) ;
#32347=ORIENTED_EDGE('',*,*,#24484,.F.) ;
#32348=ORIENTED_EDGE('',*,*,#24480,.F.) ;
#32349=ORIENTED_EDGE('',*,*,#24467,.F.) ;
#32350=ORIENTED_EDGE('',*,*,#24485,.T.) ;
#32351=ORIENTED_EDGE('',*,*,#24486,.F.) ;
#32352=ORIENTED_EDGE('',*,*,#24483,.T.) ;
#32353=ORIENTED_EDGE('',*,*,#24465,.F.) ;
#32354=ORIENTED_EDGE('',*,*,#24487,.F.) ;
#32355=ORIENTED_EDGE('',*,*,#24488,.F.) ;
#32356=ORIENTED_EDGE('',*,*,#24485,.F.) ;
#32357=ORIENTED_EDGE('',*,*,#24463,.T.) ;
#32358=ORIENTED_EDGE('',*,*,#24489,.T.) ;
#32359=ORIENTED_EDGE('',*,*,#24490,.T.) ;
#32360=ORIENTED_EDGE('',*,*,#24489,.F.) ;
#32361=ORIENTED_EDGE('',*,*,#24491,.F.) ;
#32362=ORIENTED_EDGE('',*,*,#24492,.T.) ;
#32363=ORIENTED_EDGE('',*,*,#24490,.F.) ;
#32364=ORIENTED_EDGE('',*,*,#24492,.F.) ;
#32365=ORIENTED_EDGE('',*,*,#24424,.T.) ;
#32366=ORIENTED_EDGE('',*,*,#24493,.T.) ;
#32367=ORIENTED_EDGE('',*,*,#24494,.T.) ;
#32368=ORIENTED_EDGE('',*,*,#24495,.F.) ;
#32369=ORIENTED_EDGE('',*,*,#24443,.T.) ;
#32370=ORIENTED_EDGE('',*,*,#24496,.T.) ;
#32371=ORIENTED_EDGE('',*,*,#24497,.T.) ;
#32372=ORIENTED_EDGE('',*,*,#24493,.F.) ;
#32373=ORIENTED_EDGE('',*,*,#24442,.T.) ;
#32374=ORIENTED_EDGE('',*,*,#24498,.T.) ;
#32375=ORIENTED_EDGE('',*,*,#24499,.T.) ;
#32376=ORIENTED_EDGE('',*,*,#24496,.F.) ;
#32377=ORIENTED_EDGE('',*,*,#24441,.T.) ;
#32378=ORIENTED_EDGE('',*,*,#24500,.T.) ;
#32379=ORIENTED_EDGE('',*,*,#24501,.T.) ;
#32380=ORIENTED_EDGE('',*,*,#24498,.F.) ;
#32381=ORIENTED_EDGE('',*,*,#24500,.F.) ;
#32382=ORIENTED_EDGE('',*,*,#24440,.T.) ;
#32383=ORIENTED_EDGE('',*,*,#24502,.T.) ;
#32384=ORIENTED_EDGE('',*,*,#24503,.T.) ;
#32385=ORIENTED_EDGE('',*,*,#24502,.F.) ;
#32386=ORIENTED_EDGE('',*,*,#24439,.T.) ;
#32387=ORIENTED_EDGE('',*,*,#24504,.T.) ;
#32388=ORIENTED_EDGE('',*,*,#24505,.T.) ;
#32389=ORIENTED_EDGE('',*,*,#24504,.F.) ;
#32390=ORIENTED_EDGE('',*,*,#24438,.T.) ;
#32391=ORIENTED_EDGE('',*,*,#24506,.T.) ;
#32392=ORIENTED_EDGE('',*,*,#24507,.T.) ;
#32393=ORIENTED_EDGE('',*,*,#24506,.F.) ;
#32394=ORIENTED_EDGE('',*,*,#24437,.T.) ;
#32395=ORIENTED_EDGE('',*,*,#24508,.T.) ;
#32396=ORIENTED_EDGE('',*,*,#24509,.T.) ;
#32397=ORIENTED_EDGE('',*,*,#24510,.T.) ;
#32398=ORIENTED_EDGE('',*,*,#24511,.T.) ;
#32399=ORIENTED_EDGE('',*,*,#24508,.F.) ;
#32400=ORIENTED_EDGE('',*,*,#24436,.T.) ;
#32401=ORIENTED_EDGE('',*,*,#24512,.T.) ;
#32402=ORIENTED_EDGE('',*,*,#24513,.T.) ;
#32403=ORIENTED_EDGE('',*,*,#24510,.F.) ;
#32404=ORIENTED_EDGE('',*,*,#24435,.T.) ;
#32405=ORIENTED_EDGE('',*,*,#24514,.T.) ;
#32406=ORIENTED_EDGE('',*,*,#24515,.T.) ;
#32407=ORIENTED_EDGE('',*,*,#24512,.F.) ;
#32408=ORIENTED_EDGE('',*,*,#24434,.T.) ;
#32409=ORIENTED_EDGE('',*,*,#24514,.F.) ;
#32410=ORIENTED_EDGE('',*,*,#24433,.T.) ;
#32411=ORIENTED_EDGE('',*,*,#24516,.T.) ;
#32412=ORIENTED_EDGE('',*,*,#24517,.T.) ;
#32413=ORIENTED_EDGE('',*,*,#24516,.F.) ;
#32414=ORIENTED_EDGE('',*,*,#24432,.T.) ;
#32415=ORIENTED_EDGE('',*,*,#24518,.T.) ;
#32416=ORIENTED_EDGE('',*,*,#24519,.T.) ;
#32417=ORIENTED_EDGE('',*,*,#24518,.F.) ;
#32418=ORIENTED_EDGE('',*,*,#24431,.T.) ;
#32419=ORIENTED_EDGE('',*,*,#24520,.T.) ;
#32420=ORIENTED_EDGE('',*,*,#24521,.T.) ;
#32421=ORIENTED_EDGE('',*,*,#24520,.F.) ;
#32422=ORIENTED_EDGE('',*,*,#24430,.T.) ;
#32423=ORIENTED_EDGE('',*,*,#24522,.T.) ;
#32424=ORIENTED_EDGE('',*,*,#24523,.T.) ;
#32425=ORIENTED_EDGE('',*,*,#24522,.F.) ;
#32426=ORIENTED_EDGE('',*,*,#24429,.T.) ;
#32427=ORIENTED_EDGE('',*,*,#24524,.T.) ;
#32428=ORIENTED_EDGE('',*,*,#24525,.T.) ;
#32429=ORIENTED_EDGE('',*,*,#24526,.T.) ;
#32430=ORIENTED_EDGE('',*,*,#24527,.T.) ;
#32431=ORIENTED_EDGE('',*,*,#24524,.F.) ;
#32432=ORIENTED_EDGE('',*,*,#24428,.T.) ;
#32433=ORIENTED_EDGE('',*,*,#24528,.T.) ;
#32434=ORIENTED_EDGE('',*,*,#24526,.F.) ;
#32435=ORIENTED_EDGE('',*,*,#24427,.T.) ;
#32436=ORIENTED_EDGE('',*,*,#24529,.T.) ;
#32437=ORIENTED_EDGE('',*,*,#24530,.T.) ;
#32438=ORIENTED_EDGE('',*,*,#24529,.F.) ;
#32439=ORIENTED_EDGE('',*,*,#24426,.T.) ;
#32440=ORIENTED_EDGE('',*,*,#24531,.T.) ;
#32441=ORIENTED_EDGE('',*,*,#24532,.T.) ;
#32442=ORIENTED_EDGE('',*,*,#24531,.F.) ;
#32443=ORIENTED_EDGE('',*,*,#24425,.T.) ;
#32444=ORIENTED_EDGE('',*,*,#24495,.T.) ;
#32445=ORIENTED_EDGE('',*,*,#24517,.F.) ;
#32446=ORIENTED_EDGE('',*,*,#24533,.T.) ;
#32447=ORIENTED_EDGE('',*,*,#24534,.F.) ;
#32448=ORIENTED_EDGE('',*,*,#24535,.F.) ;
#32449=ORIENTED_EDGE('',*,*,#24519,.F.) ;
#32450=ORIENTED_EDGE('',*,*,#24536,.F.) ;
#32451=ORIENTED_EDGE('',*,*,#24537,.F.) ;
#32452=ORIENTED_EDGE('',*,*,#24533,.F.) ;
#32453=ORIENTED_EDGE('',*,*,#24521,.F.) ;
#32454=ORIENTED_EDGE('',*,*,#24538,.F.) ;
#32455=ORIENTED_EDGE('',*,*,#24539,.F.) ;
#32456=ORIENTED_EDGE('',*,*,#24536,.T.) ;
#32457=ORIENTED_EDGE('',*,*,#24523,.F.) ;
#32458=ORIENTED_EDGE('',*,*,#24540,.F.) ;
#32459=ORIENTED_EDGE('',*,*,#24541,.F.) ;
#32460=ORIENTED_EDGE('',*,*,#24542,.F.) ;
#32461=ORIENTED_EDGE('',*,*,#24543,.F.) ;
#32462=ORIENTED_EDGE('',*,*,#24544,.F.) ;
#32463=ORIENTED_EDGE('',*,*,#24538,.T.) ;
#32464=ORIENTED_EDGE('',*,*,#24525,.F.) ;
#32465=ORIENTED_EDGE('',*,*,#24545,.F.) ;
#32466=ORIENTED_EDGE('',*,*,#24546,.T.) ;
#32467=ORIENTED_EDGE('',*,*,#24376,.F.) ;
#32468=ORIENTED_EDGE('',*,*,#24542,.T.) ;
#32469=ORIENTED_EDGE('',*,*,#24541,.T.) ;
#32470=ORIENTED_EDGE('',*,*,#24540,.T.) ;
#32471=ORIENTED_EDGE('',*,*,#24527,.F.) ;
#32472=ORIENTED_EDGE('',*,*,#24547,.T.) ;
#32473=ORIENTED_EDGE('',*,*,#24548,.T.) ;
#32474=ORIENTED_EDGE('',*,*,#24545,.T.) ;
#32475=ORIENTED_EDGE('',*,*,#24528,.F.) ;
#32476=ORIENTED_EDGE('',*,*,#24549,.F.) ;
#32477=ORIENTED_EDGE('',*,*,#24550,.T.) ;
#32478=ORIENTED_EDGE('',*,*,#24547,.F.) ;
#32479=ORIENTED_EDGE('',*,*,#24530,.F.) ;
#32480=ORIENTED_EDGE('',*,*,#24551,.F.) ;
#32481=ORIENTED_EDGE('',*,*,#24552,.T.) ;
#32482=ORIENTED_EDGE('',*,*,#24549,.T.) ;
#32483=ORIENTED_EDGE('',*,*,#24532,.F.) ;
#32484=ORIENTED_EDGE('',*,*,#24553,.F.) ;
#32485=ORIENTED_EDGE('',*,*,#24554,.T.) ;
#32486=ORIENTED_EDGE('',*,*,#24551,.T.) ;
#32487=ORIENTED_EDGE('',*,*,#24494,.F.) ;
#32488=ORIENTED_EDGE('',*,*,#24555,.F.) ;
#32489=ORIENTED_EDGE('',*,*,#24556,.T.) ;
#32490=ORIENTED_EDGE('',*,*,#24553,.T.) ;
#32491=ORIENTED_EDGE('',*,*,#24461,.T.) ;
#32492=ORIENTED_EDGE('',*,*,#24557,.T.) ;
#32493=ORIENTED_EDGE('',*,*,#24558,.T.) ;
#32494=ORIENTED_EDGE('',*,*,#24559,.F.) ;
#32495=ORIENTED_EDGE('',*,*,#24560,.F.) ;
#32496=ORIENTED_EDGE('',*,*,#24561,.F.) ;
#32497=ORIENTED_EDGE('',*,*,#24562,.F.) ;
#32498=ORIENTED_EDGE('',*,*,#24457,.T.) ;
#32499=ORIENTED_EDGE('',*,*,#24563,.F.) ;
#32500=ORIENTED_EDGE('',*,*,#24564,.F.) ;
#32501=ORIENTED_EDGE('',*,*,#24565,.F.) ;
#32502=ORIENTED_EDGE('',*,*,#24561,.T.) ;
#32503=ORIENTED_EDGE('',*,*,#24566,.T.) ;
#32504=ORIENTED_EDGE('',*,*,#24564,.T.) ;
#32505=ORIENTED_EDGE('',*,*,#24567,.T.) ;
#32506=ORIENTED_EDGE('',*,*,#24568,.F.) ;
#32507=ORIENTED_EDGE('',*,*,#24569,.F.) ;
#32508=ORIENTED_EDGE('',*,*,#24570,.F.) ;
#32509=ORIENTED_EDGE('',*,*,#24455,.T.) ;
#32510=ORIENTED_EDGE('',*,*,#24571,.F.) ;
#32511=ORIENTED_EDGE('',*,*,#24572,.F.) ;
#32512=ORIENTED_EDGE('',*,*,#24573,.F.) ;
#32513=ORIENTED_EDGE('',*,*,#24574,.F.) ;
#32514=ORIENTED_EDGE('',*,*,#24569,.T.) ;
#32515=ORIENTED_EDGE('',*,*,#24575,.T.) ;
#32516=ORIENTED_EDGE('',*,*,#24573,.T.) ;
#32517=ORIENTED_EDGE('',*,*,#24572,.T.) ;
#32518=ORIENTED_EDGE('',*,*,#24576,.T.) ;
#32519=ORIENTED_EDGE('',*,*,#24577,.T.) ;
#32520=ORIENTED_EDGE('',*,*,#24578,.T.) ;
#32521=ORIENTED_EDGE('',*,*,#24579,.T.) ;
#32522=ORIENTED_EDGE('',*,*,#24580,.T.) ;
#32523=ORIENTED_EDGE('',*,*,#24574,.T.) ;
#32524=ORIENTED_EDGE('',*,*,#24581,.T.) ;
#32525=ORIENTED_EDGE('',*,*,#24579,.F.) ;
#32526=ORIENTED_EDGE('',*,*,#24582,.T.) ;
#32527=ORIENTED_EDGE('',*,*,#24565,.T.) ;
#32528=ORIENTED_EDGE('',*,*,#24583,.T.) ;
#32529=ORIENTED_EDGE('',*,*,#24571,.T.) ;
#32530=ORIENTED_EDGE('',*,*,#24584,.T.) ;
#32531=ORIENTED_EDGE('',*,*,#24560,.T.) ;
#32532=ORIENTED_EDGE('',*,*,#24456,.T.) ;
#32533=ORIENTED_EDGE('',*,*,#24570,.T.) ;
#32534=ORIENTED_EDGE('',*,*,#24585,.T.) ;
#32535=ORIENTED_EDGE('',*,*,#24586,.T.) ;
#32536=ORIENTED_EDGE('',*,*,#24587,.T.) ;
#32537=ORIENTED_EDGE('',*,*,#24452,.T.) ;
#32538=ORIENTED_EDGE('',*,*,#24588,.T.) ;
#32539=ORIENTED_EDGE('',*,*,#24589,.T.) ;
#32540=ORIENTED_EDGE('',*,*,#24453,.T.) ;
#32541=ORIENTED_EDGE('',*,*,#24587,.F.) ;
#32542=ORIENTED_EDGE('',*,*,#24590,.T.) ;
#32543=ORIENTED_EDGE('',*,*,#24568,.T.) ;
#32544=ORIENTED_EDGE('',*,*,#24454,.T.) ;
#32545=ORIENTED_EDGE('',*,*,#24589,.F.) ;
#32546=ORIENTED_EDGE('',*,*,#24591,.T.) ;
#32547=ORIENTED_EDGE('',*,*,#24563,.T.) ;
#32548=ORIENTED_EDGE('',*,*,#24592,.T.) ;
#32549=ORIENTED_EDGE('',*,*,#24593,.T.) ;
#32550=ORIENTED_EDGE('',*,*,#24594,.T.) ;
#32551=ORIENTED_EDGE('',*,*,#24595,.T.) ;
#32552=ORIENTED_EDGE('',*,*,#24596,.T.) ;
#32553=ORIENTED_EDGE('',*,*,#24593,.F.) ;
#32554=ORIENTED_EDGE('',*,*,#24597,.T.) ;
#32555=ORIENTED_EDGE('',*,*,#24598,.F.) ;
#32556=ORIENTED_EDGE('',*,*,#24599,.T.) ;
#32557=ORIENTED_EDGE('',*,*,#24595,.F.) ;
#32558=ORIENTED_EDGE('',*,*,#24600,.T.) ;
#32559=ORIENTED_EDGE('',*,*,#24601,.T.) ;
#32560=ORIENTED_EDGE('',*,*,#24588,.F.) ;
#32561=ORIENTED_EDGE('',*,*,#24462,.T.) ;
#32562=ORIENTED_EDGE('',*,*,#24559,.T.) ;
#32563=ORIENTED_EDGE('',*,*,#24562,.T.) ;
#32564=ORIENTED_EDGE('',*,*,#24602,.T.) ;
#32565=ORIENTED_EDGE('',*,*,#24603,.T.) ;
#32566=ORIENTED_EDGE('',*,*,#24458,.T.) ;
#32567=ORIENTED_EDGE('',*,*,#24603,.F.) ;
#32568=ORIENTED_EDGE('',*,*,#24604,.T.) ;
#32569=ORIENTED_EDGE('',*,*,#24605,.T.) ;
#32570=ORIENTED_EDGE('',*,*,#24459,.T.) ;
#32571=ORIENTED_EDGE('',*,*,#24460,.T.) ;
#32572=ORIENTED_EDGE('',*,*,#24605,.F.) ;
#32573=ORIENTED_EDGE('',*,*,#24606,.T.) ;
#32574=ORIENTED_EDGE('',*,*,#24557,.F.) ;
#32575=ORIENTED_EDGE('',*,*,#24607,.T.) ;
#32576=ORIENTED_EDGE('',*,*,#24608,.T.) ;
#32577=ORIENTED_EDGE('',*,*,#24577,.F.) ;
#32578=ORIENTED_EDGE('',*,*,#24600,.F.) ;
#32579=ORIENTED_EDGE('',*,*,#24597,.F.) ;
#32580=ORIENTED_EDGE('',*,*,#24592,.F.) ;
#32581=ORIENTED_EDGE('',*,*,#24584,.F.) ;
#32582=ORIENTED_EDGE('',*,*,#24582,.F.) ;
#32583=ORIENTED_EDGE('',*,*,#24578,.F.) ;
#32584=ORIENTED_EDGE('',*,*,#24608,.F.) ;
#32585=ORIENTED_EDGE('',*,*,#24609,.T.) ;
#32586=ORIENTED_EDGE('',*,*,#24610,.F.) ;
#32587=ORIENTED_EDGE('',*,*,#24611,.F.) ;
#32588=ORIENTED_EDGE('',*,*,#24581,.F.) ;
#32589=ORIENTED_EDGE('',*,*,#24575,.F.) ;
#32590=ORIENTED_EDGE('',*,*,#24591,.F.) ;
#32591=ORIENTED_EDGE('',*,*,#24612,.F.) ;
#32592=ORIENTED_EDGE('',*,*,#24580,.F.) ;
#32593=ORIENTED_EDGE('',*,*,#24612,.T.) ;
#32594=ORIENTED_EDGE('',*,*,#24590,.F.) ;
#32595=ORIENTED_EDGE('',*,*,#24613,.F.) ;
#32596=ORIENTED_EDGE('',*,*,#24586,.F.) ;
#32597=ORIENTED_EDGE('',*,*,#24614,.F.) ;
#32598=ORIENTED_EDGE('',*,*,#24615,.T.) ;
#32599=ORIENTED_EDGE('',*,*,#24616,.T.) ;
#32600=ORIENTED_EDGE('',*,*,#24613,.T.) ;
#32601=ORIENTED_EDGE('',*,*,#24576,.F.) ;
#32602=ORIENTED_EDGE('',*,*,#24583,.F.) ;
#32603=ORIENTED_EDGE('',*,*,#24566,.F.) ;
#32604=ORIENTED_EDGE('',*,*,#24585,.F.) ;
#32605=ORIENTED_EDGE('',*,*,#24617,.T.) ;
#32606=ORIENTED_EDGE('',*,*,#24618,.T.) ;
#32607=ORIENTED_EDGE('',*,*,#24619,.T.) ;
#32608=ORIENTED_EDGE('',*,*,#24481,.T.) ;
#32609=ORIENTED_EDGE('',*,*,#24617,.F.) ;
#32610=ORIENTED_EDGE('',*,*,#24484,.T.) ;
#32611=ORIENTED_EDGE('',*,*,#24620,.T.) ;
#32612=ORIENTED_EDGE('',*,*,#24621,.T.) ;
#32613=ORIENTED_EDGE('',*,*,#24622,.T.) ;
#32614=ORIENTED_EDGE('',*,*,#24623,.T.) ;
#32615=ORIENTED_EDGE('',*,*,#24620,.F.) ;
#32616=ORIENTED_EDGE('',*,*,#24486,.T.) ;
#32617=ORIENTED_EDGE('',*,*,#24624,.T.) ;
#32618=ORIENTED_EDGE('',*,*,#24625,.T.) ;
#32619=ORIENTED_EDGE('',*,*,#24622,.F.) ;
#32620=ORIENTED_EDGE('',*,*,#24488,.T.) ;
#32621=ORIENTED_EDGE('',*,*,#24626,.T.) ;
#32622=ORIENTED_EDGE('',*,*,#24627,.T.) ;
#32623=ORIENTED_EDGE('',*,*,#24624,.F.) ;
#32624=ORIENTED_EDGE('',*,*,#24628,.T.) ;
#32625=ORIENTED_EDGE('',*,*,#24626,.F.) ;
#32626=ORIENTED_EDGE('',*,*,#24629,.T.) ;
#32627=ORIENTED_EDGE('',*,*,#24630,.T.) ;
#32628=ORIENTED_EDGE('',*,*,#24631,.T.) ;
#32629=ORIENTED_EDGE('',*,*,#24632,.T.) ;
#32630=ORIENTED_EDGE('',*,*,#24633,.T.) ;
#32631=ORIENTED_EDGE('',*,*,#24630,.F.) ;
#32632=ORIENTED_EDGE('',*,*,#24634,.T.) ;
#32633=ORIENTED_EDGE('',*,*,#24632,.F.) ;
#32634=ORIENTED_EDGE('',*,*,#24635,.T.) ;
#32635=ORIENTED_EDGE('',*,*,#24619,.F.) ;
#32636=ORIENTED_EDGE('',*,*,#24636,.T.) ;
#32637=ORIENTED_EDGE('',*,*,#24618,.F.) ;
#32638=ORIENTED_EDGE('',*,*,#24621,.F.) ;
#32639=ORIENTED_EDGE('',*,*,#24623,.F.) ;
#32640=ORIENTED_EDGE('',*,*,#24625,.F.) ;
#32641=ORIENTED_EDGE('',*,*,#24627,.F.) ;
#32642=ORIENTED_EDGE('',*,*,#24631,.F.) ;
#32643=ORIENTED_EDGE('',*,*,#24633,.F.) ;
#32644=ORIENTED_EDGE('',*,*,#24636,.F.) ;
#32645=ORIENTED_EDGE('',*,*,#24637,.T.) ;
#32646=ORIENTED_EDGE('',*,*,#24638,.T.) ;
#32647=ORIENTED_EDGE('',*,*,#24639,.T.) ;
#32648=ORIENTED_EDGE('',*,*,#24640,.T.) ;
#32649=ORIENTED_EDGE('',*,*,#24637,.F.) ;
#32650=ORIENTED_EDGE('',*,*,#24641,.T.) ;
#32651=ORIENTED_EDGE('',*,*,#24642,.T.) ;
#32652=ORIENTED_EDGE('',*,*,#24643,.T.) ;
#32653=ORIENTED_EDGE('',*,*,#24644,.T.) ;
#32654=ORIENTED_EDGE('',*,*,#24645,.T.) ;
#32655=ORIENTED_EDGE('',*,*,#24642,.F.) ;
#32656=ORIENTED_EDGE('',*,*,#24416,.T.) ;
#32657=ORIENTED_EDGE('',*,*,#24646,.T.) ;
#32658=ORIENTED_EDGE('',*,*,#24647,.T.) ;
#32659=ORIENTED_EDGE('',*,*,#24644,.F.) ;
#32660=ORIENTED_EDGE('',*,*,#24419,.T.) ;
#32661=ORIENTED_EDGE('',*,*,#24648,.T.) ;
#32662=ORIENTED_EDGE('',*,*,#24649,.T.) ;
#32663=ORIENTED_EDGE('',*,*,#24646,.F.) ;
#32664=ORIENTED_EDGE('',*,*,#24421,.T.) ;
#32665=ORIENTED_EDGE('',*,*,#24648,.F.) ;
#32666=ORIENTED_EDGE('',*,*,#24423,.T.) ;
#32667=ORIENTED_EDGE('',*,*,#24650,.T.) ;
#32668=ORIENTED_EDGE('',*,*,#24651,.T.) ;
#32669=ORIENTED_EDGE('',*,*,#24652,.T.) ;
#32670=ORIENTED_EDGE('',*,*,#24653,.T.) ;
#32671=ORIENTED_EDGE('',*,*,#24650,.F.) ;
#32672=ORIENTED_EDGE('',*,*,#24654,.T.) ;
#32673=ORIENTED_EDGE('',*,*,#24652,.F.) ;
#32674=ORIENTED_EDGE('',*,*,#24655,.T.) ;
#32675=ORIENTED_EDGE('',*,*,#24639,.F.) ;
#32676=ORIENTED_EDGE('',*,*,#24656,.T.) ;
#32677=ORIENTED_EDGE('',*,*,#24406,.F.) ;
#32678=ORIENTED_EDGE('',*,*,#24417,.F.) ;
#32679=ORIENTED_EDGE('',*,*,#24641,.F.) ;
#32680=ORIENTED_EDGE('',*,*,#24657,.F.) ;
#32681=ORIENTED_EDGE('',*,*,#24407,.F.) ;
#32682=ORIENTED_EDGE('',*,*,#24657,.T.) ;
#32683=ORIENTED_EDGE('',*,*,#24640,.F.) ;
#32684=ORIENTED_EDGE('',*,*,#24658,.T.) ;
#32685=ORIENTED_EDGE('',*,*,#24638,.F.) ;
#32686=ORIENTED_EDGE('',*,*,#24643,.F.) ;
#32687=ORIENTED_EDGE('',*,*,#24645,.F.) ;
#32688=ORIENTED_EDGE('',*,*,#24647,.F.) ;
#32689=ORIENTED_EDGE('',*,*,#24649,.F.) ;
#32690=ORIENTED_EDGE('',*,*,#24651,.F.) ;
#32691=ORIENTED_EDGE('',*,*,#24653,.F.) ;
#32692=ORIENTED_EDGE('',*,*,#24656,.F.) ;
#32693=ORIENTED_EDGE('',*,*,#24659,.F.) ;
#32694=ORIENTED_EDGE('',*,*,#24660,.F.) ;
#32695=ORIENTED_EDGE('',*,*,#24661,.F.) ;
#32696=ORIENTED_EDGE('',*,*,#24662,.F.) ;
#32697=ORIENTED_EDGE('',*,*,#24663,.F.) ;
#32698=ORIENTED_EDGE('',*,*,#24664,.F.) ;
#32699=ORIENTED_EDGE('',*,*,#24665,.T.) ;
#32700=ORIENTED_EDGE('',*,*,#24663,.T.) ;
#32701=ORIENTED_EDGE('',*,*,#24666,.T.) ;
#32702=ORIENTED_EDGE('',*,*,#24660,.T.) ;
#32703=ORIENTED_EDGE('',*,*,#24667,.T.) ;
#32704=ORIENTED_EDGE('',*,*,#24668,.F.) ;
#32705=ORIENTED_EDGE('',*,*,#24669,.F.) ;
#32706=ORIENTED_EDGE('',*,*,#24670,.F.) ;
#32707=ORIENTED_EDGE('',*,*,#24671,.F.) ;
#32708=ORIENTED_EDGE('',*,*,#24672,.F.) ;
#32709=ORIENTED_EDGE('',*,*,#24669,.T.) ;
#32710=ORIENTED_EDGE('',*,*,#24673,.T.) ;
#32711=ORIENTED_EDGE('',*,*,#24659,.T.) ;
#32712=ORIENTED_EDGE('',*,*,#24674,.T.) ;
#32713=ORIENTED_EDGE('',*,*,#24670,.T.) ;
#32714=ORIENTED_EDGE('',*,*,#24675,.T.) ;
#32715=ORIENTED_EDGE('',*,*,#24676,.T.) ;
#32716=ORIENTED_EDGE('',*,*,#24677,.T.) ;
#32717=ORIENTED_EDGE('',*,*,#24676,.F.) ;
#32718=ORIENTED_EDGE('',*,*,#24678,.T.) ;
#32719=ORIENTED_EDGE('',*,*,#24679,.T.) ;
#32720=ORIENTED_EDGE('',*,*,#24680,.T.) ;
#32721=ORIENTED_EDGE('',*,*,#24681,.T.) ;
#32722=ORIENTED_EDGE('',*,*,#24682,.T.) ;
#32723=ORIENTED_EDGE('',*,*,#24679,.F.) ;
#32724=ORIENTED_EDGE('',*,*,#24683,.T.) ;
#32725=ORIENTED_EDGE('',*,*,#24681,.F.) ;
#32726=ORIENTED_EDGE('',*,*,#24684,.T.) ;
#32727=ORIENTED_EDGE('',*,*,#24685,.T.) ;
#32728=ORIENTED_EDGE('',*,*,#24686,.T.) ;
#32729=ORIENTED_EDGE('',*,*,#24661,.T.) ;
#32730=ORIENTED_EDGE('',*,*,#24687,.T.) ;
#32731=ORIENTED_EDGE('',*,*,#24685,.F.) ;
#32732=ORIENTED_EDGE('',*,*,#24688,.T.) ;
#32733=ORIENTED_EDGE('',*,*,#24689,.T.) ;
#32734=ORIENTED_EDGE('',*,*,#24690,.T.) ;
#32735=ORIENTED_EDGE('',*,*,#24691,.F.) ;
#32736=ORIENTED_EDGE('',*,*,#24692,.F.) ;
#32737=ORIENTED_EDGE('',*,*,#24693,.F.) ;
#32738=ORIENTED_EDGE('',*,*,#24694,.T.) ;
#32739=ORIENTED_EDGE('',*,*,#24668,.T.) ;
#32740=ORIENTED_EDGE('',*,*,#24672,.T.) ;
#32741=ORIENTED_EDGE('',*,*,#24671,.T.) ;
#32742=ORIENTED_EDGE('',*,*,#24695,.T.) ;
#32743=ORIENTED_EDGE('',*,*,#24692,.T.) ;
#32744=ORIENTED_EDGE('',*,*,#24696,.T.) ;
#32745=ORIENTED_EDGE('',*,*,#24693,.T.) ;
#32746=ORIENTED_EDGE('',*,*,#24697,.T.) ;
#32747=ORIENTED_EDGE('',*,*,#24698,.T.) ;
#32748=ORIENTED_EDGE('',*,*,#24699,.T.) ;
#32749=ORIENTED_EDGE('',*,*,#24698,.F.) ;
#32750=ORIENTED_EDGE('',*,*,#24700,.T.) ;
#32751=ORIENTED_EDGE('',*,*,#24701,.T.) ;
#32752=ORIENTED_EDGE('',*,*,#24702,.T.) ;
#32753=ORIENTED_EDGE('',*,*,#24703,.T.) ;
#32754=ORIENTED_EDGE('',*,*,#24704,.T.) ;
#32755=ORIENTED_EDGE('',*,*,#24701,.F.) ;
#32756=ORIENTED_EDGE('',*,*,#24705,.T.) ;
#32757=ORIENTED_EDGE('',*,*,#24703,.F.) ;
#32758=ORIENTED_EDGE('',*,*,#24706,.T.) ;
#32759=ORIENTED_EDGE('',*,*,#24707,.T.) ;
#32760=ORIENTED_EDGE('',*,*,#24708,.T.) ;
#32761=ORIENTED_EDGE('',*,*,#24662,.T.) ;
#32762=ORIENTED_EDGE('',*,*,#24709,.T.) ;
#32763=ORIENTED_EDGE('',*,*,#24707,.F.) ;
#32764=ORIENTED_EDGE('',*,*,#24710,.T.) ;
#32765=ORIENTED_EDGE('',*,*,#24691,.T.) ;
#32766=ORIENTED_EDGE('',*,*,#24711,.T.) ;
#32767=ORIENTED_EDGE('',*,*,#24664,.T.) ;
#32768=ORIENTED_EDGE('',*,*,#24712,.T.) ;
#32769=ORIENTED_EDGE('',*,*,#24706,.F.) ;
#32770=ORIENTED_EDGE('',*,*,#24713,.T.) ;
#32771=ORIENTED_EDGE('',*,*,#24686,.F.) ;
#32772=ORIENTED_EDGE('',*,*,#24714,.T.) ;
#32773=ORIENTED_EDGE('',*,*,#24697,.F.) ;
#32774=ORIENTED_EDGE('',*,*,#24695,.F.) ;
#32775=ORIENTED_EDGE('',*,*,#24677,.F.) ;
#32776=ORIENTED_EDGE('',*,*,#24715,.F.) ;
#32777=ORIENTED_EDGE('',*,*,#24705,.F.) ;
#32778=ORIENTED_EDGE('',*,*,#24716,.F.) ;
#32779=ORIENTED_EDGE('',*,*,#24682,.F.) ;
#32780=ORIENTED_EDGE('',*,*,#24713,.F.) ;
#32781=ORIENTED_EDGE('',*,*,#24700,.F.) ;
#32782=ORIENTED_EDGE('',*,*,#24715,.T.) ;
#32783=ORIENTED_EDGE('',*,*,#24680,.F.) ;
#32784=ORIENTED_EDGE('',*,*,#24716,.T.) ;
#32785=ORIENTED_EDGE('',*,*,#24717,.F.) ;
#32786=ORIENTED_EDGE('',*,*,#24718,.F.) ;
#32787=ORIENTED_EDGE('',*,*,#24719,.F.) ;
#32788=ORIENTED_EDGE('',*,*,#24720,.F.) ;
#32789=ORIENTED_EDGE('',*,*,#24721,.F.) ;
#32790=ORIENTED_EDGE('',*,*,#24722,.F.) ;
#32791=ORIENTED_EDGE('',*,*,#24723,.F.) ;
#32792=ORIENTED_EDGE('',*,*,#24724,.F.) ;
#32793=ORIENTED_EDGE('',*,*,#24725,.F.) ;
#32794=ORIENTED_EDGE('',*,*,#24726,.F.) ;
#32795=ORIENTED_EDGE('',*,*,#24727,.F.) ;
#32796=ORIENTED_EDGE('',*,*,#24728,.F.) ;
#32797=ORIENTED_EDGE('',*,*,#24729,.F.) ;
#32798=ORIENTED_EDGE('',*,*,#24730,.F.) ;
#32799=ORIENTED_EDGE('',*,*,#24731,.F.) ;
#32800=ORIENTED_EDGE('',*,*,#24732,.F.) ;
#32801=ORIENTED_EDGE('',*,*,#24733,.F.) ;
#32802=ORIENTED_EDGE('',*,*,#24734,.F.) ;
#32803=ORIENTED_EDGE('',*,*,#24735,.F.) ;
#32804=ORIENTED_EDGE('',*,*,#24694,.F.) ;
#32805=ORIENTED_EDGE('',*,*,#24699,.F.) ;
#32806=ORIENTED_EDGE('',*,*,#24702,.F.) ;
#32807=ORIENTED_EDGE('',*,*,#24704,.F.) ;
#32808=ORIENTED_EDGE('',*,*,#24708,.F.) ;
#32809=ORIENTED_EDGE('',*,*,#24709,.F.) ;
#32810=ORIENTED_EDGE('',*,*,#24665,.F.) ;
#32811=ORIENTED_EDGE('',*,*,#24711,.F.) ;
#32812=ORIENTED_EDGE('',*,*,#24690,.F.) ;
#32813=ORIENTED_EDGE('',*,*,#24689,.F.) ;
#32814=ORIENTED_EDGE('',*,*,#24667,.F.) ;
#32815=ORIENTED_EDGE('',*,*,#24673,.F.) ;
#32816=ORIENTED_EDGE('',*,*,#24696,.F.) ;
#32817=ORIENTED_EDGE('',*,*,#24712,.F.) ;
#32818=ORIENTED_EDGE('',*,*,#24674,.F.) ;
#32819=ORIENTED_EDGE('',*,*,#24688,.F.) ;
#32820=ORIENTED_EDGE('',*,*,#24684,.F.) ;
#32821=ORIENTED_EDGE('',*,*,#24683,.F.) ;
#32822=ORIENTED_EDGE('',*,*,#24678,.F.) ;
#32823=ORIENTED_EDGE('',*,*,#24675,.F.) ;
#32824=ORIENTED_EDGE('',*,*,#24736,.F.) ;
#32825=ORIENTED_EDGE('',*,*,#24737,.F.) ;
#32826=ORIENTED_EDGE('',*,*,#24738,.F.) ;
#32827=ORIENTED_EDGE('',*,*,#24732,.T.) ;
#32828=ORIENTED_EDGE('',*,*,#24739,.F.) ;
#32829=ORIENTED_EDGE('',*,*,#24740,.F.) ;
#32830=ORIENTED_EDGE('',*,*,#24741,.F.) ;
#32831=ORIENTED_EDGE('',*,*,#24737,.T.) ;
#32832=ORIENTED_EDGE('',*,*,#24742,.T.) ;
#32833=ORIENTED_EDGE('',*,*,#24740,.T.) ;
#32834=ORIENTED_EDGE('',*,*,#24743,.T.) ;
#32835=ORIENTED_EDGE('',*,*,#24744,.F.) ;
#32836=ORIENTED_EDGE('',*,*,#24745,.F.) ;
#32837=ORIENTED_EDGE('',*,*,#24746,.F.) ;
#32838=ORIENTED_EDGE('',*,*,#24730,.T.) ;
#32839=ORIENTED_EDGE('',*,*,#24747,.F.) ;
#32840=ORIENTED_EDGE('',*,*,#24748,.F.) ;
#32841=ORIENTED_EDGE('',*,*,#24749,.F.) ;
#32842=ORIENTED_EDGE('',*,*,#24734,.T.) ;
#32843=ORIENTED_EDGE('',*,*,#24750,.F.) ;
#32844=ORIENTED_EDGE('',*,*,#24751,.F.) ;
#32845=ORIENTED_EDGE('',*,*,#24752,.F.) ;
#32846=ORIENTED_EDGE('',*,*,#24745,.T.) ;
#32847=ORIENTED_EDGE('',*,*,#24753,.T.) ;
#32848=ORIENTED_EDGE('',*,*,#24751,.T.) ;
#32849=ORIENTED_EDGE('',*,*,#24754,.T.) ;
#32850=ORIENTED_EDGE('',*,*,#24755,.F.) ;
#32851=ORIENTED_EDGE('',*,*,#24756,.F.) ;
#32852=ORIENTED_EDGE('',*,*,#24757,.F.) ;
#32853=ORIENTED_EDGE('',*,*,#24756,.T.) ;
#32854=ORIENTED_EDGE('',*,*,#24758,.T.) ;
#32855=ORIENTED_EDGE('',*,*,#24739,.T.) ;
#32856=ORIENTED_EDGE('',*,*,#24759,.T.) ;
#32857=ORIENTED_EDGE('',*,*,#24760,.F.) ;
#32858=ORIENTED_EDGE('',*,*,#24761,.F.) ;
#32859=ORIENTED_EDGE('',*,*,#24762,.F.) ;
#32860=ORIENTED_EDGE('',*,*,#24728,.T.) ;
#32861=ORIENTED_EDGE('',*,*,#24763,.F.) ;
#32862=ORIENTED_EDGE('',*,*,#24764,.F.) ;
#32863=ORIENTED_EDGE('',*,*,#24765,.F.) ;
#32864=ORIENTED_EDGE('',*,*,#24766,.F.) ;
#32865=ORIENTED_EDGE('',*,*,#24761,.T.) ;
#32866=ORIENTED_EDGE('',*,*,#24767,.T.) ;
#32867=ORIENTED_EDGE('',*,*,#24765,.T.) ;
#32868=ORIENTED_EDGE('',*,*,#24764,.T.) ;
#32869=ORIENTED_EDGE('',*,*,#24768,.T.) ;
#32870=ORIENTED_EDGE('',*,*,#24766,.T.) ;
#32871=ORIENTED_EDGE('',*,*,#24769,.T.) ;
#32872=ORIENTED_EDGE('',*,*,#24757,.T.) ;
#32873=ORIENTED_EDGE('',*,*,#24770,.T.) ;
#32874=ORIENTED_EDGE('',*,*,#24752,.T.) ;
#32875=ORIENTED_EDGE('',*,*,#24771,.T.) ;
#32876=ORIENTED_EDGE('',*,*,#24763,.T.) ;
#32877=ORIENTED_EDGE('',*,*,#24772,.T.) ;
#32878=ORIENTED_EDGE('',*,*,#24744,.T.) ;
#32879=ORIENTED_EDGE('',*,*,#24729,.T.) ;
#32880=ORIENTED_EDGE('',*,*,#24762,.T.) ;
#32881=ORIENTED_EDGE('',*,*,#24773,.T.) ;
#32882=ORIENTED_EDGE('',*,*,#24760,.T.) ;
#32883=ORIENTED_EDGE('',*,*,#24735,.T.) ;
#32884=ORIENTED_EDGE('',*,*,#24749,.T.) ;
#32885=ORIENTED_EDGE('',*,*,#24774,.T.) ;
#32886=ORIENTED_EDGE('',*,*,#24755,.T.) ;
#32887=ORIENTED_EDGE('',*,*,#24775,.T.) ;
#32888=ORIENTED_EDGE('',*,*,#24748,.T.) ;
#32889=ORIENTED_EDGE('',*,*,#24776,.T.) ;
#32890=ORIENTED_EDGE('',*,*,#24741,.T.) ;
#32891=ORIENTED_EDGE('',*,*,#24777,.T.) ;
#32892=ORIENTED_EDGE('',*,*,#24750,.T.) ;
#32893=ORIENTED_EDGE('',*,*,#24778,.T.) ;
#32894=ORIENTED_EDGE('',*,*,#24747,.T.) ;
#32895=ORIENTED_EDGE('',*,*,#24733,.T.) ;
#32896=ORIENTED_EDGE('',*,*,#24738,.T.) ;
#32897=ORIENTED_EDGE('',*,*,#24779,.T.) ;
#32898=ORIENTED_EDGE('',*,*,#24736,.T.) ;
#32899=ORIENTED_EDGE('',*,*,#24731,.T.) ;
#32900=ORIENTED_EDGE('',*,*,#24746,.T.) ;
#32901=ORIENTED_EDGE('',*,*,#24780,.T.) ;
#32902=ORIENTED_EDGE('',*,*,#24743,.F.) ;
#32903=ORIENTED_EDGE('',*,*,#24758,.F.) ;
#32904=ORIENTED_EDGE('',*,*,#24776,.F.) ;
#32905=ORIENTED_EDGE('',*,*,#24779,.F.) ;
#32906=ORIENTED_EDGE('',*,*,#24754,.F.) ;
#32907=ORIENTED_EDGE('',*,*,#24777,.F.) ;
#32908=ORIENTED_EDGE('',*,*,#24742,.F.) ;
#32909=ORIENTED_EDGE('',*,*,#24780,.F.) ;
#32910=ORIENTED_EDGE('',*,*,#24759,.F.) ;
#32911=ORIENTED_EDGE('',*,*,#24778,.F.) ;
#32912=ORIENTED_EDGE('',*,*,#24772,.F.) ;
#32913=ORIENTED_EDGE('',*,*,#24770,.F.) ;
#32914=ORIENTED_EDGE('',*,*,#24768,.F.) ;
#32915=ORIENTED_EDGE('',*,*,#24771,.F.) ;
#32916=ORIENTED_EDGE('',*,*,#24753,.F.) ;
#32917=ORIENTED_EDGE('',*,*,#24773,.F.) ;
#32918=ORIENTED_EDGE('',*,*,#24767,.F.) ;
#32919=ORIENTED_EDGE('',*,*,#24774,.F.) ;
#32920=ORIENTED_EDGE('',*,*,#24775,.F.) ;
#32921=ORIENTED_EDGE('',*,*,#24769,.F.) ;
#32922=ORIENTED_EDGE('',*,*,#24781,.T.) ;
#32923=ORIENTED_EDGE('',*,*,#24782,.T.) ;
#32924=ORIENTED_EDGE('',*,*,#24783,.T.) ;
#32925=ORIENTED_EDGE('',*,*,#24784,.T.) ;
#32926=ORIENTED_EDGE('',*,*,#24389,.T.) ;
#32927=ORIENTED_EDGE('',*,*,#24785,.T.) ;
#32928=ORIENTED_EDGE('',*,*,#24783,.F.) ;
#32929=ORIENTED_EDGE('',*,*,#24786,.T.) ;
#32930=ORIENTED_EDGE('',*,*,#24505,.F.) ;
#32931=ORIENTED_EDGE('',*,*,#24787,.F.) ;
#32932=ORIENTED_EDGE('',*,*,#24390,.F.) ;
#32933=ORIENTED_EDGE('',*,*,#24788,.T.) ;
#32934=ORIENTED_EDGE('',*,*,#24503,.F.) ;
#32935=ORIENTED_EDGE('',*,*,#24788,.F.) ;
#32936=ORIENTED_EDGE('',*,*,#24786,.F.) ;
#32937=ORIENTED_EDGE('',*,*,#24789,.T.) ;
#32938=ORIENTED_EDGE('',*,*,#24501,.F.) ;
#32939=ORIENTED_EDGE('',*,*,#24789,.F.) ;
#32940=ORIENTED_EDGE('',*,*,#24782,.F.) ;
#32941=ORIENTED_EDGE('',*,*,#24790,.T.) ;
#32942=ORIENTED_EDGE('',*,*,#24499,.F.) ;
#32943=ORIENTED_EDGE('',*,*,#24790,.F.) ;
#32944=ORIENTED_EDGE('',*,*,#24781,.F.) ;
#32945=ORIENTED_EDGE('',*,*,#24791,.F.) ;
#32946=ORIENTED_EDGE('',*,*,#24792,.T.) ;
#32947=ORIENTED_EDGE('',*,*,#24793,.F.) ;
#32948=ORIENTED_EDGE('',*,*,#24794,.F.) ;
#32949=ORIENTED_EDGE('',*,*,#24795,.F.) ;
#32950=ORIENTED_EDGE('',*,*,#24796,.F.) ;
#32951=ORIENTED_EDGE('',*,*,#24378,.F.) ;
#32952=ORIENTED_EDGE('',*,*,#24383,.T.) ;
#32953=ORIENTED_EDGE('',*,*,#24795,.T.) ;
#32954=ORIENTED_EDGE('',*,*,#24794,.T.) ;
#32955=ORIENTED_EDGE('',*,*,#24543,.T.) ;
#32956=ORIENTED_EDGE('',*,*,#24793,.T.) ;
#32957=ORIENTED_EDGE('',*,*,#24717,.T.) ;
#32958=ORIENTED_EDGE('',*,*,#24797,.T.) ;
#32959=ORIENTED_EDGE('',*,*,#24544,.T.) ;
#32960=ORIENTED_EDGE('',*,*,#24797,.F.) ;
#32961=ORIENTED_EDGE('',*,*,#24727,.T.) ;
#32962=ORIENTED_EDGE('',*,*,#24798,.T.) ;
#32963=ORIENTED_EDGE('',*,*,#24539,.T.) ;
#32964=ORIENTED_EDGE('',*,*,#24798,.F.) ;
#32965=ORIENTED_EDGE('',*,*,#24726,.T.) ;
#32966=ORIENTED_EDGE('',*,*,#24799,.T.) ;
#32967=ORIENTED_EDGE('',*,*,#24537,.T.) ;
#32968=ORIENTED_EDGE('',*,*,#24799,.F.) ;
#32969=ORIENTED_EDGE('',*,*,#24725,.T.) ;
#32970=ORIENTED_EDGE('',*,*,#24800,.T.) ;
#32971=ORIENTED_EDGE('',*,*,#24534,.T.) ;
#32972=ORIENTED_EDGE('',*,*,#24801,.T.) ;
#32973=ORIENTED_EDGE('',*,*,#24802,.T.) ;
#32974=ORIENTED_EDGE('',*,*,#24800,.F.) ;
#32975=ORIENTED_EDGE('',*,*,#24724,.T.) ;
#32976=ORIENTED_EDGE('',*,*,#24803,.T.) ;
#32977=ORIENTED_EDGE('',*,*,#24804,.T.) ;
#32978=ORIENTED_EDGE('',*,*,#24801,.F.) ;
#32979=ORIENTED_EDGE('',*,*,#24723,.T.) ;
#32980=ORIENTED_EDGE('',*,*,#24805,.T.) ;
#32981=ORIENTED_EDGE('',*,*,#24806,.T.) ;
#32982=ORIENTED_EDGE('',*,*,#24803,.F.) ;
#32983=ORIENTED_EDGE('',*,*,#24722,.T.) ;
#32984=ORIENTED_EDGE('',*,*,#24805,.F.) ;
#32985=ORIENTED_EDGE('',*,*,#24721,.T.) ;
#32986=ORIENTED_EDGE('',*,*,#24807,.T.) ;
#32987=ORIENTED_EDGE('',*,*,#24808,.T.) ;
#32988=ORIENTED_EDGE('',*,*,#24807,.F.) ;
#32989=ORIENTED_EDGE('',*,*,#24720,.T.) ;
#32990=ORIENTED_EDGE('',*,*,#24809,.T.) ;
#32991=ORIENTED_EDGE('',*,*,#24810,.T.) ;
#32992=ORIENTED_EDGE('',*,*,#24811,.T.) ;
#32993=ORIENTED_EDGE('',*,*,#24385,.T.) ;
#32994=ORIENTED_EDGE('',*,*,#24809,.F.) ;
#32995=ORIENTED_EDGE('',*,*,#24719,.T.) ;
#32996=ORIENTED_EDGE('',*,*,#24811,.F.) ;
#32997=ORIENTED_EDGE('',*,*,#24718,.T.) ;
#32998=ORIENTED_EDGE('',*,*,#24796,.T.) ;
#32999=ORIENTED_EDGE('',*,*,#24382,.T.) ;
#33000=ORIENTED_EDGE('',*,*,#24513,.F.) ;
#33001=ORIENTED_EDGE('',*,*,#24812,.F.) ;
#33002=ORIENTED_EDGE('',*,*,#24804,.F.) ;
#33003=ORIENTED_EDGE('',*,*,#24813,.F.) ;
#33004=ORIENTED_EDGE('',*,*,#24511,.F.) ;
#33005=ORIENTED_EDGE('',*,*,#24813,.T.) ;
#33006=ORIENTED_EDGE('',*,*,#24806,.F.) ;
#33007=ORIENTED_EDGE('',*,*,#24814,.T.) ;
#33008=ORIENTED_EDGE('',*,*,#24509,.F.) ;
#33009=ORIENTED_EDGE('',*,*,#24814,.F.) ;
#33010=ORIENTED_EDGE('',*,*,#24808,.F.) ;
#33011=ORIENTED_EDGE('',*,*,#24815,.T.) ;
#33012=ORIENTED_EDGE('',*,*,#24507,.F.) ;
#33013=ORIENTED_EDGE('',*,*,#24815,.F.) ;
#33014=ORIENTED_EDGE('',*,*,#24810,.F.) ;
#33015=ORIENTED_EDGE('',*,*,#24384,.F.) ;
#33016=ORIENTED_EDGE('',*,*,#24387,.F.) ;
#33017=ORIENTED_EDGE('',*,*,#24787,.T.) ;
#33018=ORIENTED_EDGE('',*,*,#24816,.T.) ;
#33019=ORIENTED_EDGE('',*,*,#24817,.F.) ;
#33020=ORIENTED_EDGE('',*,*,#24609,.F.) ;
#33021=ORIENTED_EDGE('',*,*,#24607,.F.) ;
#33022=ORIENTED_EDGE('',*,*,#24616,.F.) ;
#33023=ORIENTED_EDGE('',*,*,#24594,.F.) ;
#33024=ORIENTED_EDGE('',*,*,#24818,.F.) ;
#33025=ORIENTED_EDGE('',*,*,#24602,.F.) ;
#33026=ORIENTED_EDGE('',*,*,#24567,.F.) ;
#33027=ORIENTED_EDGE('',*,*,#24596,.F.) ;
#33028=ORIENTED_EDGE('',*,*,#24819,.T.) ;
#33029=ORIENTED_EDGE('',*,*,#24604,.F.) ;
#33030=ORIENTED_EDGE('',*,*,#24818,.T.) ;
#33031=ORIENTED_EDGE('',*,*,#24475,.F.) ;
#33032=ORIENTED_EDGE('',*,*,#24820,.T.) ;
#33033=ORIENTED_EDGE('',*,*,#24634,.F.) ;
#33034=ORIENTED_EDGE('',*,*,#24821,.T.) ;
#33035=ORIENTED_EDGE('',*,*,#24474,.F.) ;
#33036=ORIENTED_EDGE('',*,*,#24482,.F.) ;
#33037=ORIENTED_EDGE('',*,*,#24635,.F.) ;
#33038=ORIENTED_EDGE('',*,*,#24820,.F.) ;
#33039=ORIENTED_EDGE('',*,*,#24479,.F.) ;
#33040=ORIENTED_EDGE('',*,*,#24822,.T.) ;
#33041=ORIENTED_EDGE('',*,*,#24628,.F.) ;
#33042=ORIENTED_EDGE('',*,*,#24487,.T.) ;
#33043=ORIENTED_EDGE('',*,*,#24413,.F.) ;
#33044=ORIENTED_EDGE('',*,*,#24823,.T.) ;
#33045=ORIENTED_EDGE('',*,*,#24654,.F.) ;
#33046=ORIENTED_EDGE('',*,*,#24422,.T.) ;
#33047=ORIENTED_EDGE('',*,*,#24515,.F.) ;
#33048=ORIENTED_EDGE('',*,*,#24535,.T.) ;
#33049=ORIENTED_EDGE('',*,*,#24802,.F.) ;
#33050=ORIENTED_EDGE('',*,*,#24812,.T.) ;
#33051=ORIENTED_EDGE('',*,*,#24710,.F.) ;
#33052=ORIENTED_EDGE('',*,*,#24714,.F.) ;
#33053=ORIENTED_EDGE('',*,*,#24687,.F.) ;
#33054=ORIENTED_EDGE('',*,*,#24666,.F.) ;
#33055=ORIENTED_EDGE('',*,*,#24412,.F.) ;
#33056=ORIENTED_EDGE('',*,*,#24658,.F.) ;
#33057=ORIENTED_EDGE('',*,*,#24655,.F.) ;
#33058=ORIENTED_EDGE('',*,*,#24823,.F.) ;
#33059=ORIENTED_EDGE('',*,*,#24478,.F.) ;
#33060=ORIENTED_EDGE('',*,*,#24821,.F.) ;
#33061=ORIENTED_EDGE('',*,*,#24629,.F.) ;
#33062=ORIENTED_EDGE('',*,*,#24822,.F.) ;
#33063=ORIENTED_EDGE('',*,*,#24599,.F.) ;
#33064=ORIENTED_EDGE('',*,*,#24824,.T.) ;
#33065=ORIENTED_EDGE('',*,*,#24606,.F.) ;
#33066=ORIENTED_EDGE('',*,*,#24819,.F.) ;
#33067=ORIENTED_EDGE('',*,*,#24377,.F.) ;
#33068=ORIENTED_EDGE('',*,*,#24546,.F.) ;
#33069=ORIENTED_EDGE('',*,*,#24548,.F.) ;
#33070=ORIENTED_EDGE('',*,*,#24550,.F.) ;
#33071=ORIENTED_EDGE('',*,*,#24552,.F.) ;
#33072=ORIENTED_EDGE('',*,*,#24554,.F.) ;
#33073=ORIENTED_EDGE('',*,*,#24556,.F.) ;
#33074=ORIENTED_EDGE('',*,*,#24825,.F.) ;
#33075=ORIENTED_EDGE('',*,*,#24791,.T.) ;
#33076=ORIENTED_EDGE('',*,*,#24784,.F.) ;
#33077=ORIENTED_EDGE('',*,*,#24785,.F.) ;
#33078=ORIENTED_EDGE('',*,*,#24388,.F.) ;
#33079=ORIENTED_EDGE('',*,*,#24370,.F.) ;
#33080=ORIENTED_EDGE('',*,*,#24374,.F.) ;
#33081=ORIENTED_EDGE('',*,*,#24615,.F.) ;
#33082=ORIENTED_EDGE('',*,*,#24826,.T.) ;
#33083=ORIENTED_EDGE('',*,*,#24816,.F.) ;
#33084=ORIENTED_EDGE('',*,*,#24491,.T.) ;
#33085=ORIENTED_EDGE('',*,*,#24601,.F.) ;
#33086=ORIENTED_EDGE('',*,*,#24827,.F.) ;
#33087=ORIENTED_EDGE('',*,*,#24610,.T.) ;
#33088=ORIENTED_EDGE('',*,*,#24817,.T.) ;
#33089=ORIENTED_EDGE('',*,*,#24826,.F.) ;
#33090=ORIENTED_EDGE('',*,*,#24614,.T.) ;
#33091=ORIENTED_EDGE('',*,*,#24598,.T.) ;
#33092=ORIENTED_EDGE('',*,*,#24611,.T.) ;
#33093=ORIENTED_EDGE('',*,*,#24827,.T.) ;
#33094=ORIENTED_EDGE('',*,*,#24558,.F.) ;
#33095=ORIENTED_EDGE('',*,*,#24824,.F.) ;
#33096=ORIENTED_EDGE('',*,*,#24497,.F.) ;
#33097=ORIENTED_EDGE('',*,*,#24792,.F.) ;
#33098=ORIENTED_EDGE('',*,*,#24825,.T.) ;
#33099=ORIENTED_EDGE('',*,*,#24555,.T.) ;
#45490=TOROIDAL_SURFACE('',#49930,2.12,0.12) ;
#45491=TOROIDAL_SURFACE('',#49938,3.48,0.12) ;
#45492=TOROIDAL_SURFACE('',#49968,3.48,0.12) ;
#45493=TOROIDAL_SURFACE('',#49981,3.48,0.12) ;
#46224=ADVANCED_FACE('',(#11006),#1789,.T.) ;
#46225=ADVANCED_FACE('',(#11007),#1790,.T.) ;
#46226=ADVANCED_FACE('',(#11008),#9557,.F.) ;
#46227=ADVANCED_FACE('',(#11009),#1791,.T.) ;
#46228=ADVANCED_FACE('',(#11010),#1792,.T.) ;
#46229=ADVANCED_FACE('',(#11011),#2251,.T.) ;
#46230=ADVANCED_FACE('',(#11012),#1793,.F.) ;
#46231=ADVANCED_FACE('',(#11013),#1794,.F.) ;
#46232=ADVANCED_FACE('',(#11014),#1795,.F.) ;
#46233=ADVANCED_FACE('',(#11015),#1796,.F.) ;
#46234=ADVANCED_FACE('',(#11016),#1797,.F.) ;
#46235=ADVANCED_FACE('',(#11017),#9558,.T.) ;
#46236=ADVANCED_FACE('',(#11018),#1798,.F.) ;
#46237=ADVANCED_FACE('',(#11019),#1799,.F.) ;
#46238=ADVANCED_FACE('',(#11020),#1800,.F.) ;
#46239=ADVANCED_FACE('',(#11021),#9559,.T.) ;
#46240=ADVANCED_FACE('',(#11022),#1801,.F.) ;
#46241=ADVANCED_FACE('',(#11023),#1802,.T.) ;
#46242=ADVANCED_FACE('',(#11024),#2252,.T.) ;
#46243=ADVANCED_FACE('',(#11025),#1803,.T.) ;
#46244=ADVANCED_FACE('',(#11026),#1804,.T.) ;
#46245=ADVANCED_FACE('',(#11027,#671,#672,#673,#674),#2253,.T.) ;
#46246=ADVANCED_FACE('',(#11028),#9560,.T.) ;
#46247=ADVANCED_FACE('',(#11029),#1805,.F.) ;
#46248=ADVANCED_FACE('',(#11030),#1806,.F.) ;
#46249=ADVANCED_FACE('',(#11031),#1807,.F.) ;
#46250=ADVANCED_FACE('',(#11032),#9561,.T.) ;
#46251=ADVANCED_FACE('',(#11033),#1808,.F.) ;
#46252=ADVANCED_FACE('',(#11034),#1809,.F.) ;
#46253=ADVANCED_FACE('',(#11035),#1810,.F.) ;
#46254=ADVANCED_FACE('',(#11036),#1811,.T.) ;
#46255=ADVANCED_FACE('',(#11037),#1812,.T.) ;
#46256=ADVANCED_FACE('',(#11038),#1813,.T.) ;
#46257=ADVANCED_FACE('',(#11039),#2254,.T.) ;
#46258=ADVANCED_FACE('',(#11040),#45490,.T.) ;
#46259=ADVANCED_FACE('',(#11041),#9562,.F.) ;
#46260=ADVANCED_FACE('',(#11042),#9563,.T.) ;
#46261=ADVANCED_FACE('',(#11043),#45491,.T.) ;
#46262=ADVANCED_FACE('',(#11044),#9564,.T.) ;
#46263=ADVANCED_FACE('',(#11045),#1814,.F.) ;
#46264=ADVANCED_FACE('',(#11046),#1815,.F.) ;
#46265=ADVANCED_FACE('',(#11047),#1816,.F.) ;
#46266=ADVANCED_FACE('',(#11048),#1817,.F.) ;
#46267=ADVANCED_FACE('',(#11049),#1818,.F.) ;
#46268=ADVANCED_FACE('',(#11050),#1819,.F.) ;
#46269=ADVANCED_FACE('',(#11051),#9565,.T.) ;
#46270=ADVANCED_FACE('',(#11052),#1820,.F.) ;
#46271=ADVANCED_FACE('',(#11053),#1821,.F.) ;
#46272=ADVANCED_FACE('',(#11054),#1822,.F.) ;
#46273=ADVANCED_FACE('',(#11055),#1823,.F.) ;
#46274=ADVANCED_FACE('',(#11056),#1824,.F.) ;
#46275=ADVANCED_FACE('',(#11057),#1825,.F.) ;
#46276=ADVANCED_FACE('',(#11058),#1826,.F.) ;
#46277=ADVANCED_FACE('',(#11059),#9566,.T.) ;
#46278=ADVANCED_FACE('',(#11060),#9567,.T.) ;
#46279=ADVANCED_FACE('',(#11061),#45492,.T.) ;
#46280=ADVANCED_FACE('',(#11062),#1827,.T.) ;
#46281=ADVANCED_FACE('',(#11063),#9568,.T.) ;
#46282=ADVANCED_FACE('',(#11064),#1828,.T.) ;
#46283=ADVANCED_FACE('',(#11065),#1829,.T.) ;
#46284=ADVANCED_FACE('',(#11066),#1830,.T.) ;
#46285=ADVANCED_FACE('',(#11067),#1831,.F.) ;
#46286=ADVANCED_FACE('',(#11068),#2255,.T.) ;
#46287=ADVANCED_FACE('',(#11069),#2256,.T.) ;
#46288=ADVANCED_FACE('',(#11070),#9569,.T.) ;
#46289=ADVANCED_FACE('',(#11071),#2257,.T.) ;
#46290=ADVANCED_FACE('',(#11072),#45493,.T.) ;
#46291=ADVANCED_FACE('',(#11073),#1832,.F.) ;
#46292=ADVANCED_FACE('',(#11074),#2167,.F.) ;
#46293=ADVANCED_FACE('',(#11075),#1833,.T.) ;
#46294=ADVANCED_FACE('',(#11076),#1834,.F.) ;
#46295=ADVANCED_FACE('',(#11077),#2168,.F.) ;
#46296=ADVANCED_FACE('',(#11078),#1835,.T.) ;
#46297=ADVANCED_FACE('',(#11079),#1836,.T.) ;
#46298=ADVANCED_FACE('',(#11080),#1837,.T.) ;
#46299=ADVANCED_FACE('',(#11081),#9570,.F.) ;
#46300=ADVANCED_FACE('',(#11082),#9571,.T.) ;
#46301=ADVANCED_FACE('',(#11083),#1838,.F.) ;
#46302=ADVANCED_FACE('',(#11084),#1839,.F.) ;
#46303=ADVANCED_FACE('',(#11085),#1840,.F.) ;
#46304=ADVANCED_FACE('',(#11086),#1841,.T.) ;
#46305=ADVANCED_FACE('',(#11087),#1842,.T.) ;
#46306=ADVANCED_FACE('',(#11088),#9572,.F.) ;
#46307=ADVANCED_FACE('',(#11089),#9573,.T.) ;
#46308=ADVANCED_FACE('',(#11090),#1843,.F.) ;
#46309=ADVANCED_FACE('',(#11091),#1844,.F.) ;
#46310=ADVANCED_FACE('',(#11092),#9574,.T.) ;
#46311=ADVANCED_FACE('',(#11093),#1845,.T.) ;
#46312=ADVANCED_FACE('',(#11094),#2258,.T.) ;
#46313=ADVANCED_FACE('',(#11095),#1846,.T.) ;
#46314=ADVANCED_FACE('',(#11096),#1847,.T.) ;
#46315=ADVANCED_FACE('',(#11097),#9575,.T.) ;
#46316=ADVANCED_FACE('',(#11098),#2259,.T.) ;
#46317=ADVANCED_FACE('',(#11099),#1848,.T.) ;
#46318=ADVANCED_FACE('',(#11100),#1849,.T.) ;
#46319=ADVANCED_FACE('',(#11101),#1850,.T.) ;
#46320=ADVANCED_FACE('',(#11102),#9576,.F.) ;
#46321=ADVANCED_FACE('',(#11103),#1851,.T.) ;
#46322=ADVANCED_FACE('',(#11104),#1852,.T.) ;
#46323=ADVANCED_FACE('',(#11105),#1853,.T.) ;
#46324=ADVANCED_FACE('',(#11106),#9577,.F.) ;
#46325=ADVANCED_FACE('',(#11107),#2260,.T.) ;
#46326=ADVANCED_FACE('',(#11108),#1854,.T.) ;
#46327=ADVANCED_FACE('',(#11109),#1855,.T.) ;
#46328=ADVANCED_FACE('',(#11110),#1856,.T.) ;
#46329=ADVANCED_FACE('',(#11111),#9578,.F.) ;
#46330=ADVANCED_FACE('',(#11112),#1857,.T.) ;
#46331=ADVANCED_FACE('',(#11113),#1858,.T.) ;
#46332=ADVANCED_FACE('',(#11114),#1859,.T.) ;
#46333=ADVANCED_FACE('',(#11115),#9579,.F.) ;
#46334=ADVANCED_FACE('',(#11116),#1860,.T.) ;
#46335=ADVANCED_FACE('',(#11117),#1861,.T.) ;
#46336=ADVANCED_FACE('',(#11118),#2261,.T.) ;
#46337=ADVANCED_FACE('',(#11119),#2169,.F.) ;
#46338=ADVANCED_FACE('',(#11120),#1862,.F.) ;
#46339=ADVANCED_FACE('',(#11121),#1863,.T.) ;
#46340=ADVANCED_FACE('',(#11122),#2170,.F.) ;
#46341=ADVANCED_FACE('',(#11123),#9580,.F.) ;
#46342=ADVANCED_FACE('',(#11124),#1864,.T.) ;
#46343=ADVANCED_FACE('',(#11125),#1865,.T.) ;
#46344=ADVANCED_FACE('',(#11126),#9581,.F.) ;
#46345=ADVANCED_FACE('',(#11127),#1866,.T.) ;
#46346=ADVANCED_FACE('',(#11128),#1867,.T.) ;
#46347=ADVANCED_FACE('',(#11129),#1868,.F.) ;
#46348=ADVANCED_FACE('',(#11130),#1869,.T.) ;
#46349=ADVANCED_FACE('',(#11131),#1870,.F.) ;
#46350=ADVANCED_FACE('',(#11132),#1871,.F.) ;
#46351=ADVANCED_FACE('',(#11133),#9582,.T.) ;
#46352=ADVANCED_FACE('',(#11134),#1872,.F.) ;
#46353=ADVANCED_FACE('',(#11135),#1873,.F.) ;
#46354=ADVANCED_FACE('',(#11136),#9583,.T.) ;
#46355=ADVANCED_FACE('',(#11137),#1874,.T.) ;
#46356=ADVANCED_FACE('',(#11138),#1875,.T.) ;
#46357=ADVANCED_FACE('',(#11139),#2262,.T.) ;
#46358=ADVANCED_FACE('',(#11140),#1876,.T.) ;
#46359=ADVANCED_FACE('',(#11141,#675,#676),#2263,.F.) ;
#46360=ADVANCED_FACE('',(#11142),#2264,.T.) ;
#46361=ADVANCED_FACE('',(#11143),#2265,.F.) ;
#46362=ADVANCED_FACE('',(#11144),#1877,.F.) ;
#46363=ADVANCED_FACE('',(#11145),#2171,.F.) ;
#46364=ADVANCED_FACE('',(#11146),#1878,.T.) ;
#46365=ADVANCED_FACE('',(#11147),#1879,.F.) ;
#46366=ADVANCED_FACE('',(#11148),#1880,.F.) ;
#46367=ADVANCED_FACE('',(#11149),#2172,.F.) ;
#46368=ADVANCED_FACE('',(#11150),#1881,.T.) ;
#46369=ADVANCED_FACE('',(#11151),#2173,.F.) ;
#46370=ADVANCED_FACE('',(#11152),#1882,.T.) ;
#46371=ADVANCED_FACE('',(#11153),#1883,.F.) ;
#46372=ADVANCED_FACE('',(#11154),#2174,.F.) ;
#46373=ADVANCED_FACE('',(#11155),#1884,.T.) ;
#46374=ADVANCED_FACE('',(#11156),#9584,.F.) ;
#46375=ADVANCED_FACE('',(#11157),#1885,.T.) ;
#46376=ADVANCED_FACE('',(#11158),#1886,.F.) ;
#46377=ADVANCED_FACE('',(#11159),#9585,.T.) ;
#46378=ADVANCED_FACE('',(#11160),#1887,.T.) ;
#46379=ADVANCED_FACE('',(#11161),#9586,.F.) ;
#46380=ADVANCED_FACE('',(#11162),#1888,.F.) ;
#46381=ADVANCED_FACE('',(#11163),#9587,.T.) ;
#46382=ADVANCED_FACE('',(#11164),#1889,.T.) ;
#46383=ADVANCED_FACE('',(#11165),#2266,.T.) ;
#46384=ADVANCED_FACE('',(#11166),#2267,.F.) ;
#46385=ADVANCED_FACE('',(#11167),#1890,.T.) ;
#46386=ADVANCED_FACE('',(#11168),#2268,.T.) ;
#46387=ADVANCED_FACE('',(#11169),#1891,.F.) ;
#46388=ADVANCED_FACE('',(#11170),#1892,.F.) ;
#46389=ADVANCED_FACE('',(#11171),#1893,.T.) ;
#46390=ADVANCED_FACE('',(#11172),#1894,.T.) ;
#46391=ADVANCED_FACE('',(#11173),#1895,.T.) ;
#46392=ADVANCED_FACE('',(#11174),#2269,.T.) ;
#46393=ADVANCED_FACE('',(#11175),#2175,.T.) ;
#46394=ADVANCED_FACE('',(#11176),#1896,.F.) ;
#46395=ADVANCED_FACE('',(#11177),#1897,.F.) ;
#46396=ADVANCED_FACE('',(#11178),#1898,.F.) ;
#46397=ADVANCED_FACE('',(#11179),#1899,.F.) ;
#46398=ADVANCED_FACE('',(#11180),#1900,.F.) ;
#46399=ADVANCED_FACE('',(#11181),#1901,.F.) ;
#46400=ADVANCED_FACE('',(#11182),#9588,.T.) ;
#46401=ADVANCED_FACE('',(#11183),#1902,.F.) ;
#46402=ADVANCED_FACE('',(#11184),#1903,.F.) ;
#46403=ADVANCED_FACE('',(#11185),#1904,.F.) ;
#46404=ADVANCED_FACE('',(#11186),#1905,.F.) ;
#46405=ADVANCED_FACE('',(#11187),#9589,.T.) ;
#46406=ADVANCED_FACE('',(#11188),#2270,.T.) ;
#46407=ADVANCED_FACE('',(#11189),#1906,.F.) ;
#46408=ADVANCED_FACE('',(#11190),#1907,.T.) ;
#46409=ADVANCED_FACE('',(#11191),#1908,.T.) ;
#46410=ADVANCED_FACE('',(#11192),#2271,.T.) ;
#46411=ADVANCED_FACE('',(#11193),#1909,.T.) ;
#46412=ADVANCED_FACE('',(#11194),#1910,.T.) ;
#46413=ADVANCED_FACE('',(#11195),#1911,.T.) ;
#46414=ADVANCED_FACE('',(#11196),#2272,.T.) ;
#46415=ADVANCED_FACE('',(#11197),#1912,.T.) ;
#46416=ADVANCED_FACE('',(#11198),#1913,.T.) ;
#46417=ADVANCED_FACE('',(#11199),#1914,.F.) ;
#46418=ADVANCED_FACE('',(#11200),#1915,.T.) ;
#46419=ADVANCED_FACE('',(#11201),#2273,.T.) ;
#46420=ADVANCED_FACE('',(#11202),#1916,.T.) ;
#46421=ADVANCED_FACE('',(#11203),#2274,.T.) ;
#46422=ADVANCED_FACE('',(#11204,#677,#678),#2275,.F.) ;
#46423=ADVANCED_FACE('',(#11205),#2276,.T.) ;
#46424=ADVANCED_FACE('',(#11206),#9590,.T.) ;
#46425=ADVANCED_FACE('',(#11207),#9591,.T.) ;
#49058=CLOSED_SHELL('',(#46224,#46225,#46226,#46227,#46228,#46229,#46230,
#46231,#46232,#46233,#46234,#46235,#46236,#46237,#46238,#46239,#46240,#46241,
#46242,#46243,#46244,#46245,#46246,#46247,#46248,#46249,#46250,#46251,#46252,
#46253,#46254,#46255,#46256,#46257,#46258,#46259,#46260,#46261,#46262,#46263,
#46264,#46265,#46266,#46267,#46268,#46269,#46270,#46271,#46272,#46273,#46274,
#46275,#46276,#46277,#46278,#46279,#46280,#46281,#46282,#46283,#46284,#46285,
#46286,#46287,#46288,#46289,#46290,#46291,#46292,#46293,#46294,#46295,#46296,
#46297,#46298,#46299,#46300,#46301,#46302,#46303,#46304,#46305,#46306,#46307,
#46308,#46309,#46310,#46311,#46312,#46313,#46314,#46315,#46316,#46317,#46318,
#46319,#46320,#46321,#46322,#46323,#46324,#46325,#46326,#46327,#46328,#46329,
#46330,#46331,#46332,#46333,#46334,#46335,#46336,#46337,#46338,#46339,#46340,
#46341,#46342,#46343,#46344,#46345,#46346,#46347,#46348,#46349,#46350,#46351,
#46352,#46353,#46354,#46355,#46356,#46357,#46358,#46359,#46360,#46361,#46362,
#46363,#46364,#46365,#46366,#46367,#46368,#46369,#46370,#46371,#46372,#46373,
#46374,#46375,#46376,#46377,#46378,#46379,#46380,#46381,#46382,#46383,#46384,
#46385,#46386,#46387,#46388,#46389,#46390,#46391,#46392,#46393,#46394,#46395,
#46396,#46397,#46398,#46399,#46400,#46401,#46402,#46403,#46404,#46405,#46406,
#46407,#46408,#46409,#46410,#46411,#46412,#46413,#46414,#46415,#46416,#46417,
#46418,#46419,#46420,#46421,#46422,#46423,#46424,#46425)) ;
#49866=AXIS2_PLACEMENT_3D('',#75311,#56363,#56364) ;
#49867=AXIS2_PLACEMENT_3D('',#75338,#56365,#56366) ;
#49868=AXIS2_PLACEMENT_3D('',#75379,#56367,#56368) ;
#49869=AXIS2_PLACEMENT_3D('',#75381,#56369,#56370) ;
#49870=AXIS2_PLACEMENT_3D('',#75383,#56371,#56372) ;
#49871=AXIS2_PLACEMENT_3D('',#75384,#56373,#56374) ;
#49872=AXIS2_PLACEMENT_3D('',#75385,#56375,#56376) ;
#49873=AXIS2_PLACEMENT_3D('',#75388,#56377,#56378) ;
#49874=AXIS2_PLACEMENT_3D('',#75498,#56381,#56382) ;
#49875=AXIS2_PLACEMENT_3D('',#75538,#56387,#56388) ;
#49876=AXIS2_PLACEMENT_3D('',#75539,#56389,#56390) ;
#49877=AXIS2_PLACEMENT_3D('',#75561,#56391,#56392) ;
#49878=AXIS2_PLACEMENT_3D('',#75563,#56393,#56394) ;
#49879=AXIS2_PLACEMENT_3D('',#75564,#56395,#56396) ;
#49880=AXIS2_PLACEMENT_3D('',#75587,#56397,#56398) ;
#49881=AXIS2_PLACEMENT_3D('',#75594,#56399,#56400) ;
#49882=AXIS2_PLACEMENT_3D('',#75637,#56401,#56402) ;
#49883=AXIS2_PLACEMENT_3D('',#75644,#56403,#56404) ;
#49884=AXIS2_PLACEMENT_3D('',#75647,#56405,#56406) ;
#49885=AXIS2_PLACEMENT_3D('',#75671,#56409,#56410) ;
#49886=AXIS2_PLACEMENT_3D('',#75673,#56411,#56412) ;
#49887=AXIS2_PLACEMENT_3D('',#75674,#56413,#56414) ;
#49888=AXIS2_PLACEMENT_3D('',#75697,#56415,#56416) ;
#49889=AXIS2_PLACEMENT_3D('',#75744,#56417,#56418) ;
#49890=AXIS2_PLACEMENT_3D('',#75751,#56419,#56420) ;
#49891=AXIS2_PLACEMENT_3D('',#75754,#56421,#56422) ;
#49892=AXIS2_PLACEMENT_3D('',#75777,#56425,#56426) ;
#49893=AXIS2_PLACEMENT_3D('',#75778,#56427,#56428) ;
#49894=AXIS2_PLACEMENT_3D('',#75790,#56430,#56431) ;
#49895=AXIS2_PLACEMENT_3D('',#75792,#56433,#56434) ;
#49896=AXIS2_PLACEMENT_3D('',#75833,#56439,#56440) ;
#49897=AXIS2_PLACEMENT_3D('',#75838,#56442,#56443) ;
#49898=AXIS2_PLACEMENT_3D('',#75844,#56446,#56447) ;
#49899=AXIS2_PLACEMENT_3D('',#75846,#56448,#56449) ;
#49900=AXIS2_PLACEMENT_3D('',#75848,#56450,#56451) ;
#49901=AXIS2_PLACEMENT_3D('',#75850,#56452,#56453) ;
#49902=AXIS2_PLACEMENT_3D('',#75852,#56454,#56455) ;
#49903=AXIS2_PLACEMENT_3D('',#75860,#56456,#56457) ;
#49904=AXIS2_PLACEMENT_3D('',#75884,#56459,#56460) ;
#49905=AXIS2_PLACEMENT_3D('',#75886,#56461,#56462) ;
#49906=AXIS2_PLACEMENT_3D('',#75888,#56463,#56464) ;
#49907=AXIS2_PLACEMENT_3D('',#75891,#56466,#56467) ;
#49908=AXIS2_PLACEMENT_3D('',#75896,#56469,#56470) ;
#49909=AXIS2_PLACEMENT_3D('',#75898,#56471,#56472) ;
#49910=AXIS2_PLACEMENT_3D('',#75915,#56474,#56475) ;
#49911=AXIS2_PLACEMENT_3D('',#75931,#56476,#56477) ;
#49912=AXIS2_PLACEMENT_3D('',#75933,#56478,#56479) ;
#49913=AXIS2_PLACEMENT_3D('',#75951,#56481,#56482) ;
#49914=AXIS2_PLACEMENT_3D('',#75953,#56483,#56484) ;
#49915=AXIS2_PLACEMENT_3D('',#75957,#56486,#56487) ;
#49916=AXIS2_PLACEMENT_3D('',#75960,#56489,#56490) ;
#49917=AXIS2_PLACEMENT_3D('',#75961,#56491,#56492) ;
#49918=AXIS2_PLACEMENT_3D('',#75963,#56493,#56494) ;
#49919=AXIS2_PLACEMENT_3D('',#75966,#56496,#56497) ;
#49920=AXIS2_PLACEMENT_3D('',#75988,#56498,#56499) ;
#49921=AXIS2_PLACEMENT_3D('',#75989,#56500,#56501) ;
#49922=AXIS2_PLACEMENT_3D('',#76011,#56502,#56503) ;
#49923=AXIS2_PLACEMENT_3D('',#76053,#56504,#56505) ;
#49924=AXIS2_PLACEMENT_3D('',#76054,#56506,#56507) ;
#49925=AXIS2_PLACEMENT_3D('',#76056,#56508,#56509) ;
#49926=AXIS2_PLACEMENT_3D('',#76089,#56511,#56512) ;
#49927=AXIS2_PLACEMENT_3D('',#76111,#56513,#56514) ;
#49928=AXIS2_PLACEMENT_3D('',#76198,#56519,#56520) ;
#49929=AXIS2_PLACEMENT_3D('',#76199,#56521,#56522) ;
#49930=AXIS2_PLACEMENT_3D('',#76203,#56525,#56526) ;
#49931=AXIS2_PLACEMENT_3D('',#76205,#56527,#56528) ;
#49932=AXIS2_PLACEMENT_3D('',#76206,#56529,#56530) ;
#49933=AXIS2_PLACEMENT_3D('',#76207,#56531,#56532) ;
#49934=AXIS2_PLACEMENT_3D('',#76209,#56533,#56534) ;
#49935=AXIS2_PLACEMENT_3D('',#76211,#56536,#56537) ;
#49936=AXIS2_PLACEMENT_3D('',#76213,#56538,#56539) ;
#49937=AXIS2_PLACEMENT_3D('',#76216,#56541,#56542) ;
#49938=AXIS2_PLACEMENT_3D('',#76217,#56543,#56544) ;
#49939=AXIS2_PLACEMENT_3D('',#76235,#56545,#56546) ;
#49940=AXIS2_PLACEMENT_3D('',#76236,#56547,#56548) ;
#49941=AXIS2_PLACEMENT_3D('',#76274,#56550,#56551) ;
#49942=AXIS2_PLACEMENT_3D('',#76275,#56552,#56553) ;
#49943=AXIS2_PLACEMENT_3D('',#76297,#56554,#56555) ;
#49944=AXIS2_PLACEMENT_3D('',#76298,#56556,#56557) ;
#49945=AXIS2_PLACEMENT_3D('',#76320,#56558,#56559) ;
#49946=AXIS2_PLACEMENT_3D('',#76321,#56560,#56561) ;
#49947=AXIS2_PLACEMENT_3D('',#76348,#56562,#56563) ;
#49948=AXIS2_PLACEMENT_3D('',#76384,#56564,#56565) ;
#49949=AXIS2_PLACEMENT_3D('',#76431,#56566,#56567) ;
#49950=AXIS2_PLACEMENT_3D('',#76439,#56568,#56569) ;
#49951=AXIS2_PLACEMENT_3D('',#76441,#56570,#56571) ;
#49952=AXIS2_PLACEMENT_3D('',#76464,#56573,#56574) ;
#49953=AXIS2_PLACEMENT_3D('',#76465,#56575,#56576) ;
#49954=AXIS2_PLACEMENT_3D('',#76492,#56577,#56578) ;
#49955=AXIS2_PLACEMENT_3D('',#76524,#56579,#56580) ;
#49956=AXIS2_PLACEMENT_3D('',#76525,#56581,#56582) ;
#49957=AXIS2_PLACEMENT_3D('',#76547,#56583,#56584) ;
#49958=AXIS2_PLACEMENT_3D('',#76548,#56585,#56586) ;
#49959=AXIS2_PLACEMENT_3D('',#76570,#56587,#56588) ;
#49960=AXIS2_PLACEMENT_3D('',#76571,#56589,#56590) ;
#49961=AXIS2_PLACEMENT_3D('',#76593,#56591,#56592) ;
#49962=AXIS2_PLACEMENT_3D('',#76594,#56593,#56594) ;
#49963=AXIS2_PLACEMENT_3D('',#76616,#56595,#56596) ;
#49964=AXIS2_PLACEMENT_3D('',#76617,#56597,#56598) ;
#49965=AXIS2_PLACEMENT_3D('',#76618,#56599,#56600) ;
#49966=AXIS2_PLACEMENT_3D('',#76621,#56602,#56603) ;
#49967=AXIS2_PLACEMENT_3D('',#76622,#56604,#56605) ;
#49968=AXIS2_PLACEMENT_3D('',#76650,#56607,#56608) ;
#49969=AXIS2_PLACEMENT_3D('',#76651,#56609,#56610) ;
#49970=AXIS2_PLACEMENT_3D('',#76681,#56613,#56614) ;
#49971=AXIS2_PLACEMENT_3D('',#76684,#56616,#56617) ;
#49972=AXIS2_PLACEMENT_3D('',#76707,#56619,#56620) ;
#49973=AXIS2_PLACEMENT_3D('',#76723,#56622,#56623) ;
#49974=AXIS2_PLACEMENT_3D('',#76727,#56626,#56627) ;
#49975=AXIS2_PLACEMENT_3D('',#76760,#56629,#56630) ;
#49976=AXIS2_PLACEMENT_3D('',#76777,#56632,#56633) ;
#49977=AXIS2_PLACEMENT_3D('',#76781,#56636,#56637) ;
#49978=AXIS2_PLACEMENT_3D('',#76785,#56640,#56641) ;
#49979=AXIS2_PLACEMENT_3D('',#76788,#56643,#56644) ;
#49980=AXIS2_PLACEMENT_3D('',#76789,#56645,#56646) ;
#49981=AXIS2_PLACEMENT_3D('',#76793,#56649,#56650) ;
#49982=AXIS2_PLACEMENT_3D('',#76810,#56651,#56652) ;
#49983=AXIS2_PLACEMENT_3D('',#76851,#56653,#56654) ;
#49984=AXIS2_PLACEMENT_3D('',#76858,#56655,#56656) ;
#49985=AXIS2_PLACEMENT_3D('',#76859,#56657,#56658) ;
#49986=AXIS2_PLACEMENT_3D('',#76862,#56659,#56660) ;
#49987=AXIS2_PLACEMENT_3D('',#76864,#56661,#56662) ;
#49988=AXIS2_PLACEMENT_3D('',#76865,#56663,#56664) ;
#49989=AXIS2_PLACEMENT_3D('',#76914,#56667,#56668) ;
#49990=AXIS2_PLACEMENT_3D('',#76922,#56669,#56670) ;
#49991=AXIS2_PLACEMENT_3D('',#76923,#56671,#56672) ;
#49992=AXIS2_PLACEMENT_3D('',#76926,#56673,#56674) ;
#49993=AXIS2_PLACEMENT_3D('',#76928,#56675,#56676) ;
#49994=AXIS2_PLACEMENT_3D('',#76930,#56677,#56678) ;
#49995=AXIS2_PLACEMENT_3D('',#76931,#56679,#56680) ;
#49996=AXIS2_PLACEMENT_3D('',#76968,#56683,#56684) ;
#49997=AXIS2_PLACEMENT_3D('',#76970,#56685,#56686) ;
#49998=AXIS2_PLACEMENT_3D('',#76972,#56687,#56688) ;
#49999=AXIS2_PLACEMENT_3D('',#76973,#56689,#56690) ;
#50000=AXIS2_PLACEMENT_3D('',#76994,#56691,#56692) ;
#50001=AXIS2_PLACEMENT_3D('',#76995,#56693,#56694) ;
#50002=AXIS2_PLACEMENT_3D('',#76996,#56695,#56696) ;
#50003=AXIS2_PLACEMENT_3D('',#76999,#56699,#56700) ;
#50004=AXIS2_PLACEMENT_3D('',#77038,#56702,#56703) ;
#50005=AXIS2_PLACEMENT_3D('',#77039,#56704,#56705) ;
#50006=AXIS2_PLACEMENT_3D('',#77075,#56706,#56707) ;
#50007=AXIS2_PLACEMENT_3D('',#77076,#56708,#56709) ;
#50008=AXIS2_PLACEMENT_3D('',#77097,#56710,#56711) ;
#50009=AXIS2_PLACEMENT_3D('',#77119,#56712,#56713) ;
#50010=AXIS2_PLACEMENT_3D('',#77121,#56714,#56715) ;
#50011=AXIS2_PLACEMENT_3D('',#77122,#56716,#56717) ;
#50012=AXIS2_PLACEMENT_3D('',#77145,#56718,#56719) ;
#50013=AXIS2_PLACEMENT_3D('',#77146,#56720,#56721) ;
#50014=AXIS2_PLACEMENT_3D('',#77147,#56722,#56723) ;
#50015=AXIS2_PLACEMENT_3D('',#77148,#56724,#56725) ;
#50016=AXIS2_PLACEMENT_3D('',#77163,#56728,#56729) ;
#50017=AXIS2_PLACEMENT_3D('',#77186,#56731,#56732) ;
#50018=AXIS2_PLACEMENT_3D('',#77187,#56733,#56734) ;
#50019=AXIS2_PLACEMENT_3D('',#77209,#56735,#56736) ;
#50020=AXIS2_PLACEMENT_3D('',#77210,#56737,#56738) ;
#50021=AXIS2_PLACEMENT_3D('',#77211,#56739,#56740) ;
#50022=AXIS2_PLACEMENT_3D('',#77246,#56742,#56743) ;
#50023=AXIS2_PLACEMENT_3D('',#77247,#56744,#56745) ;
#50024=AXIS2_PLACEMENT_3D('',#77252,#56748,#56749) ;
#50025=AXIS2_PLACEMENT_3D('',#77271,#56752,#56753) ;
#50026=AXIS2_PLACEMENT_3D('',#77275,#56755,#56756) ;
#50027=AXIS2_PLACEMENT_3D('',#77277,#56758,#56759) ;
#50028=AXIS2_PLACEMENT_3D('',#77304,#56760,#56761) ;
#50029=AXIS2_PLACEMENT_3D('',#77311,#56762,#56763) ;
#50030=AXIS2_PLACEMENT_3D('',#77333,#56764,#56765) ;
#50031=AXIS2_PLACEMENT_3D('',#77334,#56766,#56767) ;
#50032=AXIS2_PLACEMENT_3D('',#77356,#56768,#56769) ;
#50033=AXIS2_PLACEMENT_3D('',#77357,#56770,#56771) ;
#50034=AXIS2_PLACEMENT_3D('',#77358,#56772,#56773) ;
#50035=AXIS2_PLACEMENT_3D('',#77360,#56774,#56775) ;
#50036=AXIS2_PLACEMENT_3D('',#77394,#56777,#56778) ;
#50037=AXIS2_PLACEMENT_3D('',#77428,#56779,#56780) ;
#50038=AXIS2_PLACEMENT_3D('',#77430,#56781,#56782) ;
#50039=AXIS2_PLACEMENT_3D('',#77462,#56783,#56784) ;
#50040=AXIS2_PLACEMENT_3D('',#77473,#56785,#56786) ;
#50041=AXIS2_PLACEMENT_3D('',#77476,#56789,#56790) ;
#50042=AXIS2_PLACEMENT_3D('',#77509,#56791,#56792) ;
#50043=AXIS2_PLACEMENT_3D('',#77518,#56793,#56794) ;
#50044=AXIS2_PLACEMENT_3D('',#77550,#56795,#56796) ;
#50045=AXIS2_PLACEMENT_3D('',#77576,#56797,#56798) ;
#50046=AXIS2_PLACEMENT_3D('',#77577,#56799,#56800) ;
#50047=AXIS2_PLACEMENT_3D('',#77578,#56801,#56802) ;
#50048=AXIS2_PLACEMENT_3D('',#77580,#56803,#56804) ;
#50049=AXIS2_PLACEMENT_3D('',#77618,#56806,#56807) ;
#50050=AXIS2_PLACEMENT_3D('',#77647,#56808,#56809) ;
#50051=AXIS2_PLACEMENT_3D('',#77674,#56810,#56811) ;
#50052=AXIS2_PLACEMENT_3D('',#77675,#56812,#56813) ;
#50053=AXIS2_PLACEMENT_3D('',#77676,#56814,#56815) ;
#50054=AXIS2_PLACEMENT_3D('',#77677,#56816,#56817) ;
#50055=AXIS2_PLACEMENT_3D('',#77708,#56822,#56823) ;
#50056=AXIS2_PLACEMENT_3D('',#77709,#56824,#56825) ;
#50057=AXIS2_PLACEMENT_3D('',#77712,#56826,#56827) ;
#50058=AXIS2_PLACEMENT_3D('',#77714,#56828,#56829) ;
#50059=AXIS2_PLACEMENT_3D('',#77715,#56830,#56831) ;
#50060=AXIS2_PLACEMENT_3D('',#77743,#56832,#56833) ;
#50061=AXIS2_PLACEMENT_3D('',#77745,#56834,#56835) ;
#50062=AXIS2_PLACEMENT_3D('',#77747,#56836,#56837) ;
#50063=AXIS2_PLACEMENT_3D('',#77763,#56840,#56841) ;
#50064=AXIS2_PLACEMENT_3D('',#77766,#56842,#56843) ;
#50065=AXIS2_PLACEMENT_3D('',#77768,#56844,#56845) ;
#50066=AXIS2_PLACEMENT_3D('',#77770,#56846,#56847) ;
#50067=AXIS2_PLACEMENT_3D('',#77772,#56848,#56849) ;
#50068=AXIS2_PLACEMENT_3D('',#77773,#56850,#56851) ;
#50069=AXIS2_PLACEMENT_3D('',#77774,#56852,#56853) ;
#50070=AXIS2_PLACEMENT_3D('',#77803,#56856,#56857) ;
#50071=AXIS2_PLACEMENT_3D('',#77832,#56858,#56859) ;
#50072=AXIS2_PLACEMENT_3D('',#77834,#56860,#56861) ;
#50073=AXIS2_PLACEMENT_3D('',#77835,#56862,#56863) ;
#50074=AXIS2_PLACEMENT_3D('',#77836,#56864,#56865) ;
#50075=AXIS2_PLACEMENT_3D('',#77839,#56866,#56867) ;
#50076=AXIS2_PLACEMENT_3D('',#77886,#56870,#56871) ;
#50077=AXIS2_PLACEMENT_3D('',#77959,#56872,#56873) ;
#50078=AXIS2_PLACEMENT_3D('',#77968,#56874,#56875) ;
#50079=AXIS2_PLACEMENT_3D('',#77978,#56876,#56877) ;
#50080=AXIS2_PLACEMENT_3D('',#78026,#56880,#56881) ;
#50081=AXIS2_PLACEMENT_3D('',#78052,#56882,#56883) ;
#50082=AXIS2_PLACEMENT_3D('',#78054,#56884,#56885) ;
#50083=AXIS2_PLACEMENT_3D('',#78055,#56886,#56887) ;
#50084=AXIS2_PLACEMENT_3D('',#78056,#56888,#56889) ;
#50085=AXIS2_PLACEMENT_3D('',#78059,#56890,#56891) ;
#50086=AXIS2_PLACEMENT_3D('',#78100,#56894,#56895) ;
#50087=AXIS2_PLACEMENT_3D('',#78135,#56896,#56897) ;
#50088=AXIS2_PLACEMENT_3D('',#78169,#56903,#56904) ;
#50089=AXIS2_PLACEMENT_3D('',#78179,#56906,#56907) ;
#50090=AXIS2_PLACEMENT_3D('',#78182,#56908,#56909) ;
#50091=AXIS2_PLACEMENT_3D('',#78214,#56912,#56913) ;
#50092=AXIS2_PLACEMENT_3D('',#78222,#56914,#56915) ;
#50093=AXIS2_PLACEMENT_3D('',#78223,#56916,#56917) ;
#50094=AXIS2_PLACEMENT_3D('',#78266,#56920,#56921) ;
#50095=AXIS2_PLACEMENT_3D('',#78267,#56922,#56923) ;
#50096=AXIS2_PLACEMENT_3D('',#78304,#56924,#56925) ;
#50097=AXIS2_PLACEMENT_3D('',#78313,#56926,#56927) ;
#50098=AXIS2_PLACEMENT_3D('',#78314,#56928,#56929) ;
#50099=AXIS2_PLACEMENT_3D('',#78317,#56930,#56931) ;
#50100=AXIS2_PLACEMENT_3D('',#78319,#56932,#56933) ;
#50101=AXIS2_PLACEMENT_3D('',#78320,#56934,#56935) ;
#50102=AXIS2_PLACEMENT_3D('',#78363,#56938,#56939) ;
#50103=AXIS2_PLACEMENT_3D('',#78365,#56940,#56941) ;
#50104=AXIS2_PLACEMENT_3D('',#78366,#56942,#56943) ;
#50105=AXIS2_PLACEMENT_3D('',#78393,#56944,#56945) ;
#50106=AXIS2_PLACEMENT_3D('',#78400,#56946,#56947) ;
#50107=AXIS2_PLACEMENT_3D('',#78401,#56948,#56949) ;
#50108=AXIS2_PLACEMENT_3D('',#78404,#56950,#56951) ;
#50109=AXIS2_PLACEMENT_3D('',#78406,#56952,#56953) ;
#50110=AXIS2_PLACEMENT_3D('',#78407,#56954,#56955) ;
#50111=AXIS2_PLACEMENT_3D('',#78418,#56958,#56959) ;
#50112=AXIS2_PLACEMENT_3D('',#78421,#56960,#56961) ;
#50113=AXIS2_PLACEMENT_3D('',#78423,#56962,#56963) ;
#50114=AXIS2_PLACEMENT_3D('',#78424,#56964,#56965) ;
#50115=AXIS2_PLACEMENT_3D('',#78489,#56966,#56967) ;
#50116=AXIS2_PLACEMENT_3D('',#78498,#56968,#56969) ;
#50117=AXIS2_PLACEMENT_3D('',#78499,#56970,#56971) ;
#50118=AXIS2_PLACEMENT_3D('',#78502,#56972,#56973) ;
#50119=AXIS2_PLACEMENT_3D('',#78504,#56974,#56975) ;
#50120=AXIS2_PLACEMENT_3D('',#78506,#56976,#56977) ;
#50121=AXIS2_PLACEMENT_3D('',#78507,#56978,#56979) ;
#50122=AXIS2_PLACEMENT_3D('',#78524,#56982,#56983) ;
#50123=AXIS2_PLACEMENT_3D('',#78551,#56986,#56987) ;
#50124=AXIS2_PLACEMENT_3D('',#78572,#56988,#56989) ;
#50125=AXIS2_PLACEMENT_3D('',#78573,#56990,#56991) ;
#50126=AXIS2_PLACEMENT_3D('',#78587,#56995,#56996) ;
#50127=AXIS2_PLACEMENT_3D('',#78614,#56999,#57000) ;
#50128=AXIS2_PLACEMENT_3D('',#78630,#57002,#57003) ;
#50129=AXIS2_PLACEMENT_3D('',#78631,#57004,#57005) ;
#50130=AXIS2_PLACEMENT_3D('',#78640,#57006,#57007) ;
#50131=AXIS2_PLACEMENT_3D('',#78691,#57008,#57009) ;
#50132=AXIS2_PLACEMENT_3D('',#78693,#57010,#57011) ;
#50133=AXIS2_PLACEMENT_3D('',#78720,#57012,#57013) ;
#50134=AXIS2_PLACEMENT_3D('',#78721,#57014,#57015) ;
#50135=AXIS2_PLACEMENT_3D('',#78766,#57020,#57021) ;
#50136=AXIS2_PLACEMENT_3D('',#78770,#57024,#57025) ;
#50137=AXIS2_PLACEMENT_3D('',#78771,#57026,#57027) ;
#50138=AXIS2_PLACEMENT_3D('',#78773,#57028,#57029) ;
#50139=AXIS2_PLACEMENT_3D('',#78774,#57030,#57031) ;
#50140=AXIS2_PLACEMENT_3D('',#78775,#57032,#57033) ;
#50141=AXIS2_PLACEMENT_3D('',#78808,#57034,#57035) ;
#50142=AXIS2_PLACEMENT_3D('',#78829,#57036,#57037) ;
#50143=AXIS2_PLACEMENT_3D('',#78850,#57038,#57039) ;
#50144=AXIS2_PLACEMENT_3D('',#78876,#57040,#57041) ;
#50145=AXIS2_PLACEMENT_3D('',#78898,#57042,#57043) ;
#50146=AXIS2_PLACEMENT_3D('',#78899,#57044,#57045) ;
#50147=AXIS2_PLACEMENT_3D('',#78900,#57046,#57047) ;
#50148=AXIS2_PLACEMENT_3D('',#78902,#57048,#57049) ;
#50149=AXIS2_PLACEMENT_3D('',#78940,#57051,#57052) ;
#50150=AXIS2_PLACEMENT_3D('',#78974,#57053,#57054) ;
#50151=AXIS2_PLACEMENT_3D('',#79010,#57055,#57056) ;
#50152=AXIS2_PLACEMENT_3D('',#79041,#57057,#57058) ;
#50153=AXIS2_PLACEMENT_3D('',#79042,#57059,#57060) ;
#50154=AXIS2_PLACEMENT_3D('',#79043,#57061,#57062) ;
#50155=AXIS2_PLACEMENT_3D('',#79100,#57067,#57068) ;
#50156=AXIS2_PLACEMENT_3D('',#79134,#57075,#57076) ;
#50157=AXIS2_PLACEMENT_3D('',#79173,#57079,#57080) ;
#50158=AXIS2_PLACEMENT_3D('',#79188,#57081,#57082) ;
#50159=AXIS2_PLACEMENT_3D('',#79190,#57084,#57085) ;
#50160=AXIS2_PLACEMENT_3D('',#79191,#57086,#57087) ;
#50161=AXIS2_PLACEMENT_3D('',#79193,#57089,#57090) ;
#50162=AXIS2_PLACEMENT_3D('',#79195,#57092,#57093) ;
#50163=AXIS2_PLACEMENT_3D('',#79196,#57094,#57095) ;
#56363=DIRECTION('axis',(0.,0.,1.)) ;
#56364=DIRECTION('refdir',(1.,0.,0.)) ;
#56365=DIRECTION('center_axis',(-0.587427618878729,0.654887367420063,-0.47544855512672)) ;
#56366=DIRECTION('ref_axis',(-0.744407146074326,-0.667725992360247,-1.89646896053702E-16)) ;
#56367=DIRECTION('center_axis',(-0.995319431851992,0.096639684280469,0.)) ;
#56368=DIRECTION('ref_axis',(-0.096639684280469,-0.995319431851992,0.)) ;
#56369=DIRECTION('center_axis',(0.,0.,-1.)) ;
#56370=DIRECTION('ref_axis',(0.318773588672553,0.947830891649361,0.)) ;
#56371=DIRECTION('center_axis',(0.947791521574129,-0.318890626441414,-5.85612796687415E-15)) ;
#56372=DIRECTION('ref_axis',(1.99840144432528E-12,5.9211894646675E-12,1.)) ;
#56373=DIRECTION('center_axis',(0.,0.,1.)) ;
#56374=DIRECTION('ref_axis',(0.096762587722359,0.995307490988224,0.)) ;
#56375=DIRECTION('center_axis',(-0.995319431851989,0.0966396842804928,-7.19611906216879E-49)) ;
#56376=DIRECTION('ref_axis',(-0.0683345760864578,-0.703797119709225,0.707106781186606)) ;
#56377=DIRECTION('center_axis',(-0.995319431851992,0.096639684280469,0.)) ;
#56378=DIRECTION('ref_axis',(-0.096639684280469,-0.995319431851992,0.)) ;
#56379=DIRECTION('',(0.995319431851989,-0.0966396842804928,7.19611906216879E-49)) ;
#56380=DIRECTION('',(-0.995319431851989,0.0966396842804928,-7.19611906216879E-49)) ;
#56381=DIRECTION('center_axis',(0.0966396842804928,0.995319431851989,0.)) ;
#56382=DIRECTION('ref_axis',(-0.995319431851989,0.0966396842804928,-5.45822738711604E-33)) ;
#56383=DIRECTION('',(0.,0.,1.)) ;
#56384=DIRECTION('',(0.995319431851989,-0.0966396842804928,0.)) ;
#56385=DIRECTION('',(0.,0.,-1.)) ;
#56386=DIRECTION('',(0.,0.,-1.)) ;
#56387=DIRECTION('center_axis',(-0.116360000472909,0.99320710342302,0.)) ;
#56388=DIRECTION('ref_axis',(0.993207103423019,0.116360000472909,0.)) ;
#56389=DIRECTION('center_axis',(0.,0.,1.)) ;
#56390=DIRECTION('ref_axis',(-0.476528951337224,-0.879158778911662,0.)) ;
#56391=DIRECTION('center_axis',(0.,0.,-1.)) ;
#56392=DIRECTION('ref_axis',(0.505066256142945,0.863080573820167,0.)) ;
#56393=DIRECTION('center_axis',(-0.0271755831899855,0.9996306756389,0.)) ;
#56394=DIRECTION('ref_axis',(0.9996306756389,0.0271755831899855,0.)) ;
#56395=DIRECTION('center_axis',(0.,0.,1.)) ;
#56396=DIRECTION('ref_axis',(-0.509318332147653,-0.860578198967609,0.)) ;
#56397=DIRECTION('center_axis',(-0.686781523075192,0.726863907181062,0.)) ;
#56398=DIRECTION('ref_axis',(-0.726863907181062,-0.686781523075192,0.)) ;
#56399=DIRECTION('center_axis',(0.515397663572033,-0.856951135353988,0.)) ;
#56400=DIRECTION('ref_axis',(0.,0.,1.)) ;
#56401=DIRECTION('center_axis',(1.,0.,0.)) ;
#56402=DIRECTION('ref_axis',(0.,1.,0.)) ;
#56403=DIRECTION('center_axis',(-1.,0.,-7.18398817372806E-49)) ;
#56404=DIRECTION('ref_axis',(-5.07984675360707E-49,0.707106781186547,0.707106781186547)) ;
#56405=DIRECTION('center_axis',(1.,0.,0.)) ;
#56406=DIRECTION('ref_axis',(0.,1.,0.)) ;
#56407=DIRECTION('',(1.,0.,7.18398817372806E-49)) ;
#56408=DIRECTION('',(-1.,0.,-7.18398817372806E-49)) ;
#56409=DIRECTION('center_axis',(0.,0.,-1.)) ;
#56410=DIRECTION('ref_axis',(0.95026155010241,-0.311453024382434,0.)) ;
#56411=DIRECTION('center_axis',(0.805994027221583,-0.591923667446348,0.)) ;
#56412=DIRECTION('ref_axis',(0.591923667446348,0.805994027221583,0.)) ;
#56413=DIRECTION('center_axis',(0.,0.,1.)) ;
#56414=DIRECTION('ref_axis',(0.950261550112609,-0.311453024351316,0.)) ;
#56415=DIRECTION('center_axis',(0.583094656822871,-0.81240422277621,0.)) ;
#56416=DIRECTION('ref_axis',(0.81240422277621,0.583094656822871,0.)) ;
#56417=DIRECTION('center_axis',(-1.,0.,0.)) ;
#56418=DIRECTION('ref_axis',(0.,-1.,0.)) ;
#56419=DIRECTION('center_axis',(1.,0.,7.18398817372806E-49)) ;
#56420=DIRECTION('ref_axis',(-5.07984675360707E-49,-0.707106781186547,0.707106781186547)) ;
#56421=DIRECTION('center_axis',(-1.,0.,0.)) ;
#56422=DIRECTION('ref_axis',(0.,-1.,0.)) ;
#56423=DIRECTION('',(-1.,0.,-7.18398817372806E-49)) ;
#56424=DIRECTION('',(1.,0.,7.18398817372806E-49)) ;
#56425=DIRECTION('center_axis',(0.,0.,-1.)) ;
#56426=DIRECTION('ref_axis',(0.87045897764999,-0.49224096561393,0.)) ;
#56427=DIRECTION('center_axis',(0.,0.,1.)) ;
#56428=DIRECTION('ref_axis',(0.870458977657674,-0.492240965600342,0.)) ;
#56429=DIRECTION('',(0.,0.,-1.)) ;
#56430=DIRECTION('center_axis',(0.,0.,1.)) ;
#56431=DIRECTION('ref_axis',(0.950261550099627,-0.311453024390925,0.)) ;
#56432=DIRECTION('',(0.,0.,1.)) ;
#56433=DIRECTION('center_axis',(0.,1.,0.)) ;
#56434=DIRECTION('ref_axis',(-1.,0.,7.51759117411176E-34)) ;
#56435=DIRECTION('',(0.,0.,1.)) ;
#56436=DIRECTION('',(1.,0.,0.)) ;
#56437=DIRECTION('',(0.,0.,-1.)) ;
#56438=DIRECTION('',(0.,0.,1.)) ;
#56439=DIRECTION('center_axis',(-7.18398817372806E-49,4.73470448533E-50,
1.)) ;
#56440=DIRECTION('ref_axis',(-1.,-8.69145204082858E-115,-7.18398817372806E-49)) ;
#56441=DIRECTION('',(0.,1.,-4.73470448533E-50)) ;
#56442=DIRECTION('center_axis',(7.18398817372806E-49,-4.73470448533E-50,
-1.)) ;
#56443=DIRECTION('ref_axis',(-0.988714441989024,-0.149812390016092,-7.03198111894656E-49)) ;
#56444=DIRECTION('',(0.52991926423319,0.848048096156435,3.40540801481717E-49)) ;
#56445=DIRECTION('',(0.,1.,-4.73470448533E-50)) ;
#56446=DIRECTION('center_axis',(0.,0.,-1.)) ;
#56447=DIRECTION('ref_axis',(-0.999999996867551,-7.91511064151848E-5,0.)) ;
#56448=DIRECTION('center_axis',(0.,0.,-1.)) ;
#56449=DIRECTION('ref_axis',(0.695780933920748,0.718254058110618,0.)) ;
#56450=DIRECTION('center_axis',(0.,0.,-1.)) ;
#56451=DIRECTION('ref_axis',(0.719657715388816,0.694329008958541,0.)) ;
#56452=DIRECTION('center_axis',(0.,0.,-1.)) ;
#56453=DIRECTION('ref_axis',(0.588307081130752,0.808637606280721,0.)) ;
#56454=DIRECTION('center_axis',(0.,0.,-1.)) ;
#56455=DIRECTION('ref_axis',(-0.864233277861794,-0.503091285390891,0.)) ;
#56456=DIRECTION('center_axis',(0.,0.,-1.)) ;
#56457=DIRECTION('ref_axis',(0.951152389067781,-0.308721772427299,0.)) ;
#56458=DIRECTION('',(-1.,0.,-7.18398817372806E-49)) ;
#56459=DIRECTION('center_axis',(0.,0.,1.)) ;
#56460=DIRECTION('ref_axis',(-0.508512638759206,-0.86105452569634,0.)) ;
#56461=DIRECTION('center_axis',(0.,0.,1.)) ;
#56462=DIRECTION('ref_axis',(-0.575679505271721,-0.817675429012091,0.)) ;
#56463=DIRECTION('center_axis',(0.,0.,1.)) ;
#56464=DIRECTION('ref_axis',(-0.999001972402703,0.0446660848464377,0.)) ;
#56465=DIRECTION('',(0.801695394071906,-0.597732795757345,6.04237904485494E-49)) ;
#56466=DIRECTION('center_axis',(7.18398817372806E-49,-4.73470448533E-50,
-1.)) ;
#56467=DIRECTION('ref_axis',(-0.564686561222103,0.825305451075634,-4.44745931978026E-49)) ;
#56468=DIRECTION('',(1.,0.,7.18398817372806E-49)) ;
#56469=DIRECTION('center_axis',(0.,0.,1.)) ;
#56470=DIRECTION('ref_axis',(0.87103386621213,-0.491222967614045,0.)) ;
#56471=DIRECTION('center_axis',(0.,0.,1.)) ;
#56472=DIRECTION('ref_axis',(-0.557169735681217,-0.830398630563011,0.)) ;
#56473=DIRECTION('',(-0.995319431851989,0.0966396842804928,-7.19611906216879E-49)) ;
#56474=DIRECTION('center_axis',(0.,0.,-1.)) ;
#56475=DIRECTION('ref_axis',(-0.686121032649195,0.727487407833567,0.)) ;
#56476=DIRECTION('center_axis',(0.,0.,-1.)) ;
#56477=DIRECTION('ref_axis',(0.559966405429213,0.828515313552312,0.)) ;
#56478=DIRECTION('center_axis',(0.,0.,-1.)) ;
#56479=DIRECTION('ref_axis',(0.502348696023835,0.864665130326852,0.)) ;
#56480=DIRECTION('',(0.995319431851989,-0.0966396842804928,7.19611906216879E-49)) ;
#56481=DIRECTION('center_axis',(0.,0.,1.)) ;
#56482=DIRECTION('ref_axis',(0.710148456608062,0.704051965111374,0.)) ;
#56483=DIRECTION('center_axis',(0.,0.,1.)) ;
#56484=DIRECTION('ref_axis',(-0.980153473557896,-0.198240178249495,0.)) ;
#56485=DIRECTION('',(0.,-1.,4.73470448533E-50)) ;
#56486=DIRECTION('center_axis',(7.18398817372806E-49,-4.73470448533E-50,
-1.)) ;
#56487=DIRECTION('ref_axis',(0.382998231470488,-0.923749075610081,3.1888226546038E-49)) ;
#56488=DIRECTION('',(-0.992304006159154,0.123825519827269,-7.18732796940279E-49)) ;
#56489=DIRECTION('center_axis',(-7.18398817372806E-49,4.73470448533E-50,
1.)) ;
#56490=DIRECTION('ref_axis',(0.600000000000003,0.799999999999998,3.93161654541046E-49)) ;
#56491=DIRECTION('center_axis',(-1.,0.,-7.18398817372806E-49)) ;
#56492=DIRECTION('ref_axis',(-5.07984675360707E-49,0.707106781186547,0.707106781186547)) ;
#56493=DIRECTION('center_axis',(-1.,0.,0.)) ;
#56494=DIRECTION('ref_axis',(0.,0.,1.)) ;
#56495=DIRECTION('',(-1.,0.,-7.18398817372806E-49)) ;
#56496=DIRECTION('center_axis',(1.,0.,0.)) ;
#56497=DIRECTION('ref_axis',(0.,1.,0.)) ;
#56498=DIRECTION('center_axis',(0.,0.,-1.)) ;
#56499=DIRECTION('ref_axis',(0.871033866206537,-0.491222967623962,0.)) ;
#56500=DIRECTION('center_axis',(0.517399992172763,-0.855743681308617,0.)) ;
#56501=DIRECTION('ref_axis',(0.855743681308617,0.517399992172763,0.)) ;
#56502=DIRECTION('center_axis',(0.248948925328251,-0.968516614507933,0.)) ;
#56503=DIRECTION('ref_axis',(0.968516614507933,0.248948925328251,0.)) ;
#56504=DIRECTION('center_axis',(-0.995319431851992,0.096639684280469,0.)) ;
#56505=DIRECTION('ref_axis',(-0.096639684280469,-0.995319431851992,0.)) ;
#56506=DIRECTION('center_axis',(0.995319431851989,-0.0966396842804928,7.19611906216879E-49)) ;
#56507=DIRECTION('ref_axis',(-0.0683345760864578,-0.703797119709225,0.707106781186606)) ;
#56508=DIRECTION('center_axis',(-0.995319431851992,0.096639684280469,0.)) ;
#56509=DIRECTION('ref_axis',(-0.096639684280469,-0.995319431851992,0.)) ;
#56510=DIRECTION('',(0.995319431851989,-0.0966396842804928,7.19611906216879E-49)) ;
#56511=DIRECTION('center_axis',(-0.164953742105299,0.986301304351494,0.)) ;
#56512=DIRECTION('ref_axis',(-0.986301304351494,-0.164953742105299,0.)) ;
#56513=DIRECTION('center_axis',(-0.45978265173531,0.888031482078899,0.)) ;
#56514=DIRECTION('ref_axis',(-0.888031482078899,-0.45978265173531,0.)) ;
#56515=DIRECTION('',(0.,0.,-1.)) ;
#56516=DIRECTION('',(0.,0.,1.)) ;
#56517=DIRECTION('',(0.,0.,1.)) ;
#56518=DIRECTION('',(0.,0.,-1.)) ;
#56519=DIRECTION('center_axis',(0.,0.,1.)) ;
#56520=DIRECTION('ref_axis',(0.871033866207808,-0.491222967621709,0.)) ;
#56521=DIRECTION('center_axis',(0.,1.,0.)) ;
#56522=DIRECTION('ref_axis',(-1.,0.,0.)) ;
#56523=DIRECTION('',(0.,0.,1.)) ;
#56524=DIRECTION('',(1.,0.,0.)) ;
#56525=DIRECTION('center_axis',(7.18398817372806E-49,-4.73470448533E-50,
-1.)) ;
#56526=DIRECTION('ref_axis',(-1.,0.,0.)) ;
#56527=DIRECTION('center_axis',(0.,-1.,4.73470448533E-50)) ;
#56528=DIRECTION('ref_axis',(1.,0.,0.)) ;
#56529=DIRECTION('center_axis',(7.18398817372806E-49,-4.73470448533E-50,
-1.)) ;
#56530=DIRECTION('ref_axis',(0.600000000000003,0.799999999999998,3.93161654541046E-49)) ;
#56531=DIRECTION('center_axis',(0.,0.,1.)) ;
#56532=DIRECTION('ref_axis',(-1.,0.,0.)) ;
#56533=DIRECTION('center_axis',(-1.09763027743844E-32,-3.07546720254364E-67,
1.)) ;
#56534=DIRECTION('ref_axis',(-1.,1.74482680966927E-115,-1.09763027743844E-32)) ;
#56535=DIRECTION('',(0.,0.,1.)) ;
#56536=DIRECTION('center_axis',(0.,-1.,4.73470448533E-50)) ;
#56537=DIRECTION('ref_axis',(-0.707106781186495,3.34794164849145E-50,0.7071067811866)) ;
#56538=DIRECTION('center_axis',(-0.0703834704923706,-0.997519963951429,
0.000297657167785072)) ;
#56539=DIRECTION('ref_axis',(0.997396008926277,-0.0703794229952271,-0.0157460533719646)) ;
#56540=DIRECTION('',(0.,-1.,4.73470448533E-50)) ;
#56541=DIRECTION('center_axis',(0.0703834704969201,-0.997519963951109,-0.000297657163792654)) ;
#56542=DIRECTION('ref_axis',(0.997396008921092,0.0703794229994621,-0.0157460536814624)) ;
#56543=DIRECTION('center_axis',(-7.18398817372806E-49,4.73470448533E-50,
1.)) ;
#56544=DIRECTION('ref_axis',(1.,0.,0.)) ;
#56545=DIRECTION('center_axis',(-7.18398817372806E-49,4.73470448533E-50,
1.)) ;
#56546=DIRECTION('ref_axis',(-0.564686561222103,0.825305451075634,-4.44745931978026E-49)) ;
#56547=DIRECTION('center_axis',(-0.801695394071906,0.597732795757345,-6.04237904485494E-49)) ;
#56548=DIRECTION('ref_axis',(0.422660913217549,0.566884249594181,0.707106781186654)) ;
#56549=DIRECTION('',(-0.801695394071906,0.597732795757345,-6.04237904485494E-49)) ;
#56550=DIRECTION('center_axis',(0.0446052839668792,0.999004688999123,0.)) ;
#56551=DIRECTION('ref_axis',(0.,0.,1.)) ;
#56552=DIRECTION('center_axis',(0.,0.,-1.)) ;
#56553=DIRECTION('ref_axis',(-0.996530462288612,0.083228827522952,0.)) ;
#56554=DIRECTION('center_axis',(-0.0271755831899875,0.9996306756389,0.)) ;
#56555=DIRECTION('ref_axis',(0.,0.,1.)) ;
#56556=DIRECTION('center_axis',(0.,0.,-1.)) ;
#56557=DIRECTION('ref_axis',(0.566808378068744,0.823849660163236,0.)) ;
#56558=DIRECTION('center_axis',(-0.116360000473519,0.993207103422948,0.)) ;
#56559=DIRECTION('ref_axis',(0.,0.,1.)) ;
#56560=DIRECTION('center_axis',(0.,0.,-1.)) ;
#56561=DIRECTION('ref_axis',(0.509318333459063,0.860578198191473,0.)) ;
#56562=DIRECTION('center_axis',(-0.488003536614868,0.872841651304165,0.)) ;
#56563=DIRECTION('ref_axis',(0.,0.,1.)) ;
#56564=DIRECTION('center_axis',(-0.707983649981725,0.70622882365318,0.)) ;
#56565=DIRECTION('ref_axis',(0.,0.,1.)) ;
#56566=DIRECTION('center_axis',(1.,0.,0.)) ;
#56567=DIRECTION('ref_axis',(0.,0.,1.)) ;
#56568=DIRECTION('center_axis',(1.,0.,7.18398817372806E-49)) ;
#56569=DIRECTION('ref_axis',(-5.07984675360707E-49,-0.707106781186547,0.707106781186547)) ;
#56570=DIRECTION('center_axis',(1.,0.,0.)) ;
#56571=DIRECTION('ref_axis',(0.,0.,1.)) ;
#56572=DIRECTION('',(1.,0.,7.18398817372806E-49)) ;
#56573=DIRECTION('center_axis',(0.809381734448945,-0.587282902816366,0.)) ;
#56574=DIRECTION('ref_axis',(0.,0.,1.)) ;
#56575=DIRECTION('center_axis',(0.,0.,1.)) ;
#56576=DIRECTION('ref_axis',(0.95115238906757,-0.308721772427949,0.)) ;
#56577=DIRECTION('center_axis',(0.548205483813554,-0.83634367787217,0.)) ;
#56578=DIRECTION('ref_axis',(0.,0.,1.)) ;
#56579=DIRECTION('center_axis',(0.503089999549594,-0.864234026380118,0.)) ;
#56580=DIRECTION('ref_axis',(0.,0.,1.)) ;
#56581=DIRECTION('center_axis',(0.,0.,1.)) ;
#56582=DIRECTION('ref_axis',(-0.836344700122326,-0.548203924262949,0.)) ;
#56583=DIRECTION('center_axis',(0.231127698080859,-0.972923423081099,0.)) ;
#56584=DIRECTION('ref_axis',(0.,0.,1.)) ;
#56585=DIRECTION('center_axis',(0.,0.,1.)) ;
#56586=DIRECTION('ref_axis',(-0.588703310582201,-0.808349189465516,0.)) ;
#56587=DIRECTION('center_axis',(0.199440361015477,-0.9799099664755,0.)) ;
#56588=DIRECTION('ref_axis',(0.,0.,1.)) ;
#56589=DIRECTION('center_axis',(0.,0.,1.)) ;
#56590=DIRECTION('ref_axis',(0.731503731905511,0.681837436789965,0.)) ;
#56591=DIRECTION('center_axis',(0.195410291837853,-0.980721580186673,0.)) ;
#56592=DIRECTION('ref_axis',(0.,0.,1.)) ;
#56593=DIRECTION('center_axis',(0.,0.,1.)) ;
#56594=DIRECTION('ref_axis',(0.710838965198327,0.703354793511619,0.)) ;
#56595=DIRECTION('center_axis',(0.,-1.,0.)) ;
#56596=DIRECTION('ref_axis',(0.,0.,1.)) ;
#56597=DIRECTION('center_axis',(0.,0.,1.)) ;
#56598=DIRECTION('ref_axis',(-0.980737044055406,-0.195332666027636,0.)) ;
#56599=DIRECTION('center_axis',(0.,-1.,4.73470448533E-50)) ;
#56600=DIRECTION('ref_axis',(-0.707106781186495,3.34794164849145E-50,0.7071067811866)) ;
#56601=DIRECTION('',(0.,-1.,4.73470448533E-50)) ;
#56602=DIRECTION('center_axis',(-0.27563735581696,-0.96126169593833,0.)) ;
#56603=DIRECTION('ref_axis',(-0.96126169593833,0.27563735581696,-1.7177296129898E-49)) ;
#56604=DIRECTION('center_axis',(-0.52991926423319,-0.848048096156435,-3.40540801481717E-49)) ;
#56605=DIRECTION('ref_axis',(-0.599660559564581,0.37470950522069,0.707106781186519)) ;
#56606=DIRECTION('',(-0.52991926423319,-0.848048096156435,-3.40540801481717E-49)) ;
#56607=DIRECTION('center_axis',(-7.18398817372806E-49,4.73470448533E-50,
1.)) ;
#56608=DIRECTION('ref_axis',(1.,0.,0.)) ;
#56609=DIRECTION('center_axis',(-7.18398817372806E-49,4.73470448533E-50,
1.)) ;
#56610=DIRECTION('ref_axis',(-0.988714441989024,-0.149812390016092,-7.03198111894657E-49)) ;
#56611=DIRECTION('',(0.,0.,-1.)) ;
#56612=DIRECTION('',(0.,0.,-1.)) ;
#56613=DIRECTION('center_axis',(0.,0.,-1.)) ;
#56614=DIRECTION('ref_axis',(-0.850596491898227,-0.525818987837477,0.)) ;
#56615=DIRECTION('',(0.,0.,1.)) ;
#56616=DIRECTION('center_axis',(0.,0.,-1.)) ;
#56617=DIRECTION('ref_axis',(-0.864233152292046,-0.5030915011003,0.)) ;
#56618=DIRECTION('',(0.,0.,1.)) ;
#56619=DIRECTION('center_axis',(0.,0.,-1.)) ;
#56620=DIRECTION('ref_axis',(0.58870331058208,0.808349189465604,0.)) ;
#56621=DIRECTION('',(0.,0.,1.)) ;
#56622=DIRECTION('center_axis',(0.,0.,-1.)) ;
#56623=DIRECTION('ref_axis',(-0.0605458183509709,0.99816541909656,0.)) ;
#56624=DIRECTION('',(0.,0.,1.)) ;
#56625=DIRECTION('',(-1.69617406539954E-14,0.,1.)) ;
#56626=DIRECTION('center_axis',(0.,0.,-1.)) ;
#56627=DIRECTION('ref_axis',(0.73297616972146,0.680254316135118,0.)) ;
#56628=DIRECTION('',(0.,0.,1.)) ;
#56629=DIRECTION('center_axis',(0.,0.,1.)) ;
#56630=DIRECTION('ref_axis',(0.0630245162323191,-0.998011979063218,0.)) ;
#56631=DIRECTION('',(0.,0.,-1.)) ;
#56632=DIRECTION('center_axis',(-1.,0.,0.)) ;
#56633=DIRECTION('ref_axis',(0.,-1.,0.)) ;
#56634=DIRECTION('',(0.,0.,1.)) ;
#56635=DIRECTION('',(0.,-1.,0.)) ;
#56636=DIRECTION('center_axis',(-0.848048096156435,0.52991926423319,0.)) ;
#56637=DIRECTION('ref_axis',(-0.52991926423319,-0.848048096156435,0.)) ;
#56638=DIRECTION('',(0.,0.,1.)) ;
#56639=DIRECTION('',(-0.52991926423319,-0.848048096156435,0.)) ;
#56640=DIRECTION('center_axis',(0.,0.,1.)) ;
#56641=DIRECTION('ref_axis',(-1.,0.,0.)) ;
#56642=DIRECTION('',(0.,0.,1.)) ;
#56643=DIRECTION('center_axis',(-1.09763027743844E-32,-3.07546720254364E-67,
1.)) ;
#56644=DIRECTION('ref_axis',(-1.,1.74482680966927E-115,-1.09763027743844E-32)) ;
#56645=DIRECTION('center_axis',(-1.,0.,0.)) ;
#56646=DIRECTION('ref_axis',(0.,-1.,0.)) ;
#56647=DIRECTION('',(0.,0.,1.)) ;
#56648=DIRECTION('',(0.,-1.,0.)) ;
#56649=DIRECTION('center_axis',(-7.18398817372806E-49,4.73470448533E-50,
1.)) ;
#56650=DIRECTION('ref_axis',(1.,0.,0.)) ;
#56651=DIRECTION('center_axis',(-7.18398817372806E-49,4.73470448533E-50,
1.)) ;
#56652=DIRECTION('ref_axis',(0.382998231470488,-0.923749075610081,3.1888226546038E-49)) ;
#56653=DIRECTION('center_axis',(0.995319431851992,-0.096639684280469,0.)) ;
#56654=DIRECTION('ref_axis',(0.096639684280469,0.995319431851992,0.)) ;
#56655=DIRECTION('center_axis',(-0.205129249961233,0.978734893017686,-3.0494635128401E-13)) ;
#56656=DIRECTION('ref_axis',(-7.40148683083438E-14,2.96059473233375E-13,
1.)) ;
#56657=DIRECTION('center_axis',(-0.823739491888484,0.435623967792083,0.362884290357663)) ;
#56658=DIRECTION('ref_axis',(-0.566968473112313,-0.632911145682689,-0.527228823346485)) ;
#56659=DIRECTION('center_axis',(-0.205129249960219,0.978734893017899,6.14991217244375E-10)) ;
#56660=DIRECTION('ref_axis',(-0.978734893017899,-0.205129249960219,-7.97116905459272E-27)) ;
#56661=DIRECTION('center_axis',(0.,0.,1.)) ;
#56662=DIRECTION('ref_axis',(-0.096639684280469,-0.995319431851992,0.)) ;
#56663=DIRECTION('center_axis',(0.995319431884589,-0.0966396839447406,0.)) ;
#56664=DIRECTION('ref_axis',(0.,0.,-1.)) ;
#56665=DIRECTION('',(0.,0.,-1.)) ;
#56666=DIRECTION('',(0.,0.,1.)) ;
#56667=DIRECTION('center_axis',(-0.103428412047358,0.99463690037187,0.)) ;
#56668=DIRECTION('ref_axis',(-0.99463690037187,-0.103428412047358,0.)) ;
#56669=DIRECTION('center_axis',(-0.995319431851992,0.096639684280469,0.)) ;
#56670=DIRECTION('ref_axis',(0.,0.,1.)) ;
#56671=DIRECTION('center_axis',(-0.369434341203981,-0.833228591457252,0.411398082053555)) ;
#56672=DIRECTION('ref_axis',(0.556714224316335,-0.552928670244287,-0.619950931982319)) ;
#56673=DIRECTION('center_axis',(-0.995319431851991,0.096639684280469,-2.15264418689913E-8)) ;
#56674=DIRECTION('ref_axis',(-0.0966396842804691,-0.995319431851992,-1.81350378306141E-24)) ;
#56675=DIRECTION('center_axis',(0.,0.,1.)) ;
#56676=DIRECTION('ref_axis',(0.99463690037187,0.103428412047358,0.)) ;
#56677=DIRECTION('center_axis',(0.,0.,1.)) ;
#56678=DIRECTION('ref_axis',(0.99463690037187,0.103428412047358,0.)) ;
#56679=DIRECTION('center_axis',(-0.103428467957002,0.994636894558043,0.)) ;
#56680=DIRECTION('ref_axis',(0.,0.,-1.)) ;
#56681=DIRECTION('',(0.,0.,-1.)) ;
#56682=DIRECTION('',(0.,0.,1.)) ;
#56683=DIRECTION('center_axis',(0.0757934708266429,0.997123537872841,0.)) ;
#56684=DIRECTION('ref_axis',(0.997123537872841,-0.0757934708266429,0.)) ;
#56685=DIRECTION('center_axis',(0.,0.,1.)) ;
#56686=DIRECTION('ref_axis',(-0.556954524428844,-0.830542989687012,0.)) ;
#56687=DIRECTION('center_axis',(0.0327072745977339,-0.999464973967767,0.)) ;
#56688=DIRECTION('ref_axis',(0.,0.,-1.)) ;
#56689=DIRECTION('center_axis',(0.,0.,-1.)) ;
#56690=DIRECTION('ref_axis',(0.548199354674537,0.836347695360262,0.)) ;
#56691=DIRECTION('center_axis',(0.,0.,-1.)) ;
#56692=DIRECTION('ref_axis',(0.499475161905295,0.866328207228461,0.)) ;
#56693=DIRECTION('center_axis',(0.,0.,1.)) ;
#56694=DIRECTION('ref_axis',(-0.498945449405617,-0.866633393377746,0.)) ;
#56695=DIRECTION('center_axis',(-0.995319431851989,0.0966396842804928,-1.09249274412357E-32)) ;
#56696=DIRECTION('ref_axis',(-0.0683345760864603,-0.703797119709251,-0.70710678118658)) ;
#56697=DIRECTION('',(0.995319431851989,-0.0966396842804928,1.09249274412357E-32)) ;
#56698=DIRECTION('',(-0.995319431851989,0.0966396842804928,-1.09249274412357E-32)) ;
#56699=DIRECTION('center_axis',(-0.995319431851989,0.0966396842804928,-7.19611906216879E-49)) ;
#56700=DIRECTION('ref_axis',(0.0683345760864578,0.703797119709225,0.707106781186606)) ;
#56701=DIRECTION('',(-0.995319431851989,0.0966396842804928,-7.19611906216879E-49)) ;
#56702=DIRECTION('center_axis',(0.,0.,1.)) ;
#56703=DIRECTION('ref_axis',(-0.543457078351713,-0.839436956530638,0.)) ;
#56704=DIRECTION('center_axis',(0.0757934708213221,0.997123537873245,0.)) ;
#56705=DIRECTION('ref_axis',(-0.997123537873245,0.0757934708213221,0.)) ;
#56706=DIRECTION('center_axis',(-0.032707310967753,0.999464972777565,0.)) ;
#56707=DIRECTION('ref_axis',(-0.999464972777565,-0.032707310967753,0.)) ;
#56708=DIRECTION('center_axis',(0.,0.,1.)) ;
#56709=DIRECTION('ref_axis',(-0.568977005763106,-0.822353431872726,0.)) ;
#56710=DIRECTION('center_axis',(0.,0.,1.)) ;
#56711=DIRECTION('ref_axis',(-0.501869373976784,-0.864943426741975,0.)) ;
#56712=DIRECTION('center_axis',(0.,0.,-1.)) ;
#56713=DIRECTION('ref_axis',(0.711895385472461,0.702285526081106,0.)) ;
#56714=DIRECTION('center_axis',(-0.198321321731455,0.980137058449832,0.)) ;
#56715=DIRECTION('ref_axis',(0.,0.,-1.)) ;
#56716=DIRECTION('center_axis',(0.,0.,1.)) ;
#56717=DIRECTION('ref_axis',(0.7258408460618,0.687862679746684,0.)) ;
#56718=DIRECTION('center_axis',(-2.96059473233386E-13,1.,0.)) ;
#56719=DIRECTION('ref_axis',(0.,0.,-1.)) ;
#56720=DIRECTION('center_axis',(0.,0.,1.)) ;
#56721=DIRECTION('ref_axis',(-0.980153473557867,-0.198240178249636,0.)) ;
#56722=DIRECTION('center_axis',(0.,0.,-1.)) ;
#56723=DIRECTION('ref_axis',(-0.99999999657314,-8.2787195019415E-5,0.)) ;
#56724=DIRECTION('center_axis',(0.,1.,3.07546720254364E-67)) ;
#56725=DIRECTION('ref_axis',(-0.707106781186574,2.17468371423535E-67,-0.707106781186521)) ;
#56726=DIRECTION('',(0.,-1.,-3.07546720254364E-67)) ;
#56727=DIRECTION('',(0.,1.,3.07546720254364E-67)) ;
#56728=DIRECTION('center_axis',(0.992304006159154,-0.123825519827269,7.18732796940279E-49)) ;
#56729=DIRECTION('ref_axis',(-0.087557864753804,-0.701664891753657,0.707106781186606)) ;
#56730=DIRECTION('',(0.992304006159154,-0.123825519827269,7.18732796940279E-49)) ;
#56731=DIRECTION('center_axis',(0.,0.,-1.)) ;
#56732=DIRECTION('ref_axis',(0.695398896812718,0.718623944989071,0.)) ;
#56733=DIRECTION('center_axis',(0.198321321723131,-0.980137058451516,0.)) ;
#56734=DIRECTION('ref_axis',(0.980137058451516,0.198321321723131,0.)) ;
#56735=DIRECTION('center_axis',(0.,0.,-1.)) ;
#56736=DIRECTION('ref_axis',(-0.99999999657314,-8.27871951115587E-5,0.)) ;
#56737=DIRECTION('center_axis',(2.96059473233364E-13,-1.,0.)) ;
#56738=DIRECTION('ref_axis',(1.,2.96059473233364E-13,0.)) ;
#56739=DIRECTION('center_axis',(0.,1.,-4.73470448533E-50)) ;
#56740=DIRECTION('ref_axis',(0.707106781186547,3.34794164849121E-50,0.707106781186547)) ;
#56741=DIRECTION('',(0.,1.,-4.73470448533E-50)) ;
#56742=DIRECTION('center_axis',(0.,0.,1.)) ;
#56743=DIRECTION('ref_axis',(-0.250389541446926,-0.968145173790583,0.)) ;
#56744=DIRECTION('center_axis',(-1.09763027743844E-32,-3.07546720254364E-67,
1.)) ;
#56745=DIRECTION('ref_axis',(-1.,1.74482680966927E-115,-1.09763027743844E-32)) ;
#56746=DIRECTION('',(-0.707106781186472,0.707106781186623,-1.01994663078385E-65)) ;
#56747=DIRECTION('',(0.992304006159154,-0.123825519827269,1.08918292158375E-32)) ;
#56748=DIRECTION('center_axis',(-1.09763027743844E-32,-3.07546720254364E-67,
1.)) ;
#56749=DIRECTION('ref_axis',(-1.,3.3757259187808E-99,-1.09763027743844E-32)) ;
#56750=DIRECTION('',(0.,0.,1.)) ;
#56751=DIRECTION('',(0.,0.,1.)) ;
#56752=DIRECTION('center_axis',(0.,0.,-1.)) ;
#56753=DIRECTION('ref_axis',(-0.996836376575686,0.0794810564566027,0.)) ;
#56754=DIRECTION('',(0.,0.,1.)) ;
#56755=DIRECTION('center_axis',(0.,0.,1.)) ;
#56756=DIRECTION('ref_axis',(0.988785171592188,0.149344850729469,0.)) ;
#56757=DIRECTION('',(0.,0.,1.)) ;
#56758=DIRECTION('center_axis',(0.0966396842804928,0.995319431851989,0.)) ;
#56759=DIRECTION('ref_axis',(-0.995319431851989,0.0966396842804928,-5.45822738711604E-33)) ;
#56760=DIRECTION('center_axis',(0.248948925327991,-0.968516614508,0.)) ;
#56761=DIRECTION('ref_axis',(-0.968516614508,-0.248948925327991,0.)) ;
#56762=DIRECTION('center_axis',(0.995319431851992,-0.096639684280469,0.)) ;
#56763=DIRECTION('ref_axis',(0.,0.,-1.)) ;
#56764=DIRECTION('center_axis',(0.517399992172731,-0.855743681308637,0.)) ;
#56765=DIRECTION('ref_axis',(-0.855743681308637,-0.517399992172731,0.)) ;
#56766=DIRECTION('center_axis',(0.,0.,-1.)) ;
#56767=DIRECTION('ref_axis',(0.560035503521478,0.828468608213639,0.)) ;
#56768=DIRECTION('center_axis',(1.,0.,0.)) ;
#56769=DIRECTION('ref_axis',(0.,-1.,0.)) ;
#56770=DIRECTION('center_axis',(0.,0.,-1.)) ;
#56771=DIRECTION('ref_axis',(0.871033866220507,-0.491222967599191,0.)) ;
#56772=DIRECTION('center_axis',(-1.,0.,0.)) ;
#56773=DIRECTION('ref_axis',(0.,-0.707106781186574,-0.707106781186521)) ;
#56774=DIRECTION('center_axis',(1.,0.,0.)) ;
#56775=DIRECTION('ref_axis',(0.,-1.,0.)) ;
#56776=DIRECTION('',(-1.,0.,0.)) ;
#56777=DIRECTION('center_axis',(-0.45978265173519,0.888031482078962,0.)) ;
#56778=DIRECTION('ref_axis',(0.888031482078962,0.45978265173519,0.)) ;
#56779=DIRECTION('center_axis',(0.,0.,-1.)) ;
#56780=DIRECTION('ref_axis',(0.707405248487832,-0.706808187850048,0.)) ;
#56781=DIRECTION('center_axis',(-0.164953742105275,0.986301304351498,0.)) ;
#56782=DIRECTION('ref_axis',(0.986301304351498,0.164953742105275,0.)) ;
#56783=DIRECTION('center_axis',(-0.995319431851992,0.096639684280469,0.)) ;
#56784=DIRECTION('ref_axis',(0.096639684280469,0.995319431851992,0.)) ;
#56785=DIRECTION('center_axis',(0.995319431851989,-0.0966396842804928,0.)) ;
#56786=DIRECTION('ref_axis',(0.0683345760864603,0.703797119709251,-0.70710678118658)) ;
#56787=DIRECTION('',(-0.995319431851989,0.0966396842804928,0.)) ;
#56788=DIRECTION('',(0.995319431851989,-0.0966396842804928,0.)) ;
#56789=DIRECTION('center_axis',(0.,0.,1.)) ;
#56790=DIRECTION('ref_axis',(-1.,0.,0.)) ;
#56791=DIRECTION('center_axis',(0.583094656822871,-0.81240422277621,0.)) ;
#56792=DIRECTION('ref_axis',(-0.81240422277621,-0.583094656822871,0.)) ;
#56793=DIRECTION('center_axis',(1.,0.,0.)) ;
#56794=DIRECTION('ref_axis',(0.,0.,-1.)) ;
#56795=DIRECTION('center_axis',(0.805994027221688,-0.591923667446204,0.)) ;
#56796=DIRECTION('ref_axis',(-0.591923667446204,-0.805994027221688,0.)) ;
#56797=DIRECTION('center_axis',(1.,0.,0.)) ;
#56798=DIRECTION('ref_axis',(0.,-1.,0.)) ;
#56799=DIRECTION('center_axis',(0.,0.,-1.)) ;
#56800=DIRECTION('ref_axis',(0.950261550112188,-0.311453024352601,0.)) ;
#56801=DIRECTION('center_axis',(-1.,0.,0.)) ;
#56802=DIRECTION('ref_axis',(0.,-0.707106781186574,-0.707106781186521)) ;
#56803=DIRECTION('center_axis',(1.,0.,0.)) ;
#56804=DIRECTION('ref_axis',(0.,-1.,0.)) ;
#56805=DIRECTION('',(-1.,0.,0.)) ;
#56806=DIRECTION('center_axis',(-0.686781523075266,0.726863907180992,0.)) ;
#56807=DIRECTION('ref_axis',(0.726863907180992,0.686781523075266,0.)) ;
#56808=DIRECTION('center_axis',(-0.515397663572599,0.856951135353648,0.)) ;
#56809=DIRECTION('ref_axis',(0.856951135353648,0.515397663572599,0.)) ;
#56810=DIRECTION('center_axis',(-1.,0.,0.)) ;
#56811=DIRECTION('ref_axis',(0.,1.,0.)) ;
#56812=DIRECTION('center_axis',(0.,0.,-1.)) ;
#56813=DIRECTION('ref_axis',(0.870458977666652,-0.492240965584466,0.)) ;
#56814=DIRECTION('center_axis',(0.,0.,1.)) ;
#56815=DIRECTION('ref_axis',(0.870458977653571,-0.492240965607597,0.)) ;
#56816=DIRECTION('center_axis',(1.,0.,0.)) ;
#56817=DIRECTION('ref_axis',(0.,0.707106781186574,-0.707106781186521)) ;
#56818=DIRECTION('',(-1.,0.,0.)) ;
#56819=DIRECTION('',(1.,0.,0.)) ;
#56820=DIRECTION('',(0.,0.,-1.)) ;
#56821=DIRECTION('',(0.,0.,1.)) ;
#56822=DIRECTION('center_axis',(0.,0.,1.)) ;
#56823=DIRECTION('ref_axis',(-1.,0.,0.)) ;
#56824=DIRECTION('center_axis',(-0.9039126820276,0.356838437056911,0.235813895070778)) ;
#56825=DIRECTION('ref_axis',(0.427717036450173,0.754121910522067,0.49835557667275)) ;
#56826=DIRECTION('center_axis',(-1.,0.,-2.96059473233375E-13)) ;
#56827=DIRECTION('ref_axis',(0.,1.,0.)) ;
#56828=DIRECTION('center_axis',(0.,0.,-1.)) ;
#56829=DIRECTION('ref_axis',(0.858256747734086,0.513220571459202,0.)) ;
#56830=DIRECTION('center_axis',(0.513220571458668,-0.858256747734405,0.)) ;
#56831=DIRECTION('ref_axis',(0.,0.,1.)) ;
#56832=DIRECTION('center_axis',(0.513220571458983,-0.858256747734216,-5.08190081266363E-13)) ;
#56833=DIRECTION('ref_axis',(-0.858256747734216,-0.513220571458983,-2.16500831402799E-29)) ;
#56834=DIRECTION('center_axis',(0.,0.,1.)) ;
#56835=DIRECTION('ref_axis',(-0.557171124810912,-0.830397698501714,0.)) ;
#56836=DIRECTION('center_axis',(-1.,0.,0.)) ;
#56837=DIRECTION('ref_axis',(0.,0.,-1.)) ;
#56838=DIRECTION('',(0.,0.,1.)) ;
#56839=DIRECTION('',(0.,0.,-1.)) ;
#56840=DIRECTION('center_axis',(-0.198151110421921,-0.949811551695269,0.242062293025544)) ;
#56841=DIRECTION('ref_axis',(-0.601638685605581,0.312822659451454,0.734964540448387)) ;
#56842=DIRECTION('center_axis',(0.,0.,-1.)) ;
#56843=DIRECTION('ref_axis',(0.,1.,0.)) ;
#56844=DIRECTION('center_axis',(1.,-2.81256499571696E-12,0.)) ;
#56845=DIRECTION('ref_axis',(0.,0.,1.)) ;
#56846=DIRECTION('center_axis',(0.57437040532927,-0.818595527401592,2.78906268328281E-12)) ;
#56847=DIRECTION('ref_axis',(-0.818595527401592,-0.57437040532927,1.14085547468979E-28)) ;
#56848=DIRECTION('center_axis',(0.,0.,-1.)) ;
#56849=DIRECTION('ref_axis',(0.,1.,0.)) ;
#56850=DIRECTION('center_axis',(0.,0.,-1.)) ;
#56851=DIRECTION('ref_axis',(0.,1.,0.)) ;
#56852=DIRECTION('center_axis',(-1.,0.,0.)) ;
#56853=DIRECTION('ref_axis',(0.,0.707106781186561,0.707106781186534)) ;
#56854=DIRECTION('',(1.,0.,0.)) ;
#56855=DIRECTION('',(-1.,0.,0.)) ;
#56856=DIRECTION('center_axis',(0.805994027221583,-0.591923667446348,0.)) ;
#56857=DIRECTION('ref_axis',(0.,0.,1.)) ;
#56858=DIRECTION('center_axis',(0.,0.,1.)) ;
#56859=DIRECTION('ref_axis',(0.95026155011525,-0.311453024343258,0.)) ;
#56860=DIRECTION('center_axis',(1.,0.,0.)) ;
#56861=DIRECTION('ref_axis',(0.,0.,1.)) ;
#56862=DIRECTION('center_axis',(0.,0.,-1.)) ;
#56863=DIRECTION('ref_axis',(0.95026155010268,-0.311453024381611,0.)) ;
#56864=DIRECTION('center_axis',(1.,0.,0.)) ;
#56865=DIRECTION('ref_axis',(0.,-0.707106781186561,0.707106781186534)) ;
#56866=DIRECTION('center_axis',(1.,0.,0.)) ;
#56867=DIRECTION('ref_axis',(0.,0.,1.)) ;
#56868=DIRECTION('',(-1.,0.,0.)) ;
#56869=DIRECTION('',(1.,0.,0.)) ;
#56870=DIRECTION('center_axis',(-0.686781523075266,0.726863907180992,0.)) ;
#56871=DIRECTION('ref_axis',(0.,0.,1.)) ;
#56872=DIRECTION('center_axis',(0.,0.,-1.)) ;
#56873=DIRECTION('ref_axis',(0.327194307029667,0.944957081272677,0.)) ;
#56874=DIRECTION('center_axis',(1.,0.,0.)) ;
#56875=DIRECTION('ref_axis',(0.,-1.,0.)) ;
#56876=DIRECTION('center_axis',(0.574370405327453,-0.818595527402866,5.3993661000774E-13)) ;
#56877=DIRECTION('ref_axis',(5.18104078158406E-13,-2.96059473233376E-13,
-1.)) ;
#56878=DIRECTION('',(0.,0.,-1.)) ;
#56879=DIRECTION('',(0.,0.,1.)) ;
#56880=DIRECTION('center_axis',(-0.805994027221724,0.591923667446156,0.)) ;
#56881=DIRECTION('ref_axis',(0.591923667446156,0.805994027221724,0.)) ;
#56882=DIRECTION('center_axis',(0.,0.,1.)) ;
#56883=DIRECTION('ref_axis',(0.95026155010112,-0.311453024386369,0.)) ;
#56884=DIRECTION('center_axis',(-1.,0.,0.)) ;
#56885=DIRECTION('ref_axis',(0.,1.,0.)) ;
#56886=DIRECTION('center_axis',(0.,0.,-1.)) ;
#56887=DIRECTION('ref_axis',(0.950261550111873,-0.311453024353561,0.)) ;
#56888=DIRECTION('center_axis',(1.,0.,0.)) ;
#56889=DIRECTION('ref_axis',(0.,0.707106781186561,-0.707106781186534)) ;
#56890=DIRECTION('center_axis',(-1.,0.,0.)) ;
#56891=DIRECTION('ref_axis',(0.,1.,0.)) ;
#56892=DIRECTION('',(-1.,0.,0.)) ;
#56893=DIRECTION('',(1.,0.,0.)) ;
#56894=DIRECTION('center_axis',(0.686781523075266,-0.726863907180992,0.)) ;
#56895=DIRECTION('ref_axis',(-0.726863907180992,-0.686781523075266,0.)) ;
#56896=DIRECTION('center_axis',(-1.,0.,0.)) ;
#56897=DIRECTION('ref_axis',(0.,-0.707106781186561,-0.707106781186534)) ;
#56898=DIRECTION('',(1.,0.,0.)) ;
#56899=DIRECTION('',(-1.,0.,0.)) ;
#56900=DIRECTION('',(0.,0.,1.)) ;
#56901=DIRECTION('',(0.,0.,-1.)) ;
#56902=DIRECTION('',(0.,0.,1.)) ;
#56903=DIRECTION('center_axis',(0.,1.,0.)) ;
#56904=DIRECTION('ref_axis',(-1.,0.,7.51759117411176E-34)) ;
#56905=DIRECTION('',(0.,0.,-1.)) ;
#56906=DIRECTION('center_axis',(0.,0.,1.)) ;
#56907=DIRECTION('ref_axis',(-1.,0.,0.)) ;
#56908=DIRECTION('center_axis',(0.,0.,1.)) ;
#56909=DIRECTION('ref_axis',(0.721343829160339,0.692577129374266,0.)) ;
#56910=DIRECTION('',(-0.995319431851989,0.0966396842804928,0.)) ;
#56911=DIRECTION('',(1.,0.,0.)) ;
#56912=DIRECTION('center_axis',(0.,0.,1.)) ;
#56913=DIRECTION('ref_axis',(0.951152389067664,-0.308721772427659,0.)) ;
#56914=DIRECTION('center_axis',(0.,0.,1.)) ;
#56915=DIRECTION('ref_axis',(-0.836344563545471,-0.548204132625737,0.)) ;
#56916=DIRECTION('center_axis',(0.,0.,1.)) ;
#56917=DIRECTION('ref_axis',(-0.58830708113082,-0.808637606280671,0.)) ;
#56918=DIRECTION('',(-1.,0.,0.)) ;
#56919=DIRECTION('',(0.995319431851989,-0.0966396842804928,0.)) ;
#56920=DIRECTION('center_axis',(0.,-1.,0.)) ;
#56921=DIRECTION('ref_axis',(1.,0.,0.)) ;
#56922=DIRECTION('center_axis',(0.,0.,1.)) ;
#56923=DIRECTION('ref_axis',(-1.,0.,0.)) ;
#56924=DIRECTION('center_axis',(-1.,0.,0.)) ;
#56925=DIRECTION('ref_axis',(0.,1.,0.)) ;
#56926=DIRECTION('center_axis',(-0.467163988180043,0.884170689486887,4.00075432832064E-13)) ;
#56927=DIRECTION('ref_axis',(-2.96059473233375E-13,2.96059473233375E-13,
-1.)) ;
#56928=DIRECTION('center_axis',(-0.245569634402396,-0.928738932586164,-0.277740075895048)) ;
#56929=DIRECTION('ref_axis',(0.615184564295696,-0.37073439967014,0.695775794889083)) ;
#56930=DIRECTION('center_axis',(-0.467163988180506,0.884170689486642,1.72376051565199E-12)) ;
#56931=DIRECTION('ref_axis',(0.884170689486642,0.467163988180506,2.87117640726933E-30)) ;
#56932=DIRECTION('center_axis',(0.,0.,-1.)) ;
#56933=DIRECTION('ref_axis',(0.,-1.,0.)) ;
#56934=DIRECTION('center_axis',(-1.,6.66133814775069E-13,0.)) ;
#56935=DIRECTION('ref_axis',(0.,0.,1.)) ;
#56936=DIRECTION('',(0.,0.,1.)) ;
#56937=DIRECTION('',(0.,0.,-1.)) ;
#56938=DIRECTION('center_axis',(-0.520123256650074,0.854091211693295,-5.05723588454344E-13)) ;
#56939=DIRECTION('ref_axis',(0.854091211693295,0.520123256650074,1.77749193559808E-29)) ;
#56940=DIRECTION('center_axis',(0.,0.,1.)) ;
#56941=DIRECTION('ref_axis',(-0.553419070298074,-0.832902955109666,0.)) ;
#56942=DIRECTION('center_axis',(1.,0.,0.)) ;
#56943=DIRECTION('ref_axis',(0.,0.,-1.)) ;
#56944=DIRECTION('center_axis',(0.160503998606273,-0.987035190067405,-1.18796823198059E-14)) ;
#56945=DIRECTION('ref_axis',(-0.987035190067405,-0.160503998606273,-9.21627772871048E-32)) ;
#56946=DIRECTION('center_axis',(-0.995319431851992,0.096639684280469,0.)) ;
#56947=DIRECTION('ref_axis',(0.,0.,-1.)) ;
#56948=DIRECTION('center_axis',(-0.905234052991426,0.354988520804968,-0.233526142865029)) ;
#56949=DIRECTION('ref_axis',(-0.424913296220226,-0.756266514397689,0.497503416969204)) ;
#56950=DIRECTION('center_axis',(1.,0.,-7.40148683083437E-14)) ;
#56951=DIRECTION('ref_axis',(0.,-1.,0.)) ;
#56952=DIRECTION('center_axis',(0.,0.,-1.)) ;
#56953=DIRECTION('ref_axis',(-0.854091211693295,-0.520123256650074,0.)) ;
#56954=DIRECTION('center_axis',(-0.520123256651582,0.854091211692377,-2.528617942269E-13)) ;
#56955=DIRECTION('ref_axis',(5.49867212303732E-29,2.96059473233375E-13,
1.)) ;
#56956=DIRECTION('',(0.,0.,1.)) ;
#56957=DIRECTION('',(8.45884209238215E-14,0.,-1.)) ;
#56958=DIRECTION('center_axis',(-0.815753560152279,0.437411293584229,0.378440866376576)) ;
#56959=DIRECTION('ref_axis',(0.578399627505853,0.616908799770245,0.533739078264957)) ;
#56960=DIRECTION('center_axis',(0.,0.,-1.)) ;
#56961=DIRECTION('ref_axis',(0.987035190067405,0.160503998606273,0.)) ;
#56962=DIRECTION('center_axis',(0.160504422009498,-0.987035121216767,0.)) ;
#56963=DIRECTION('ref_axis',(0.,0.,1.)) ;
#56964=DIRECTION('center_axis',(-0.995319431851971,0.096639684280467,2.05513535042918E-7)) ;
#56965=DIRECTION('ref_axis',(0.096639684280469,0.995319431851992,-7.31253112867355E-24)) ;
#56966=DIRECTION('center_axis',(0.995319431851992,-0.096639684280469,0.)) ;
#56967=DIRECTION('ref_axis',(-0.096639684280469,-0.995319431851992,0.)) ;
#56968=DIRECTION('center_axis',(0.2434402440985,-0.969915897154626,-2.69134591984373E-13)) ;
#56969=DIRECTION('ref_axis',(7.40148683083438E-14,2.96059473233375E-13,
-1.)) ;
#56970=DIRECTION('center_axis',(-0.324142602044054,-0.870147708379737,0.371179928257984)) ;
#56971=DIRECTION('ref_axis',(-0.572356119989909,0.492790995860895,0.655412470363911)) ;
#56972=DIRECTION('center_axis',(0.243440244098866,-0.969915897154534,1.80181976079286E-14)) ;
#56973=DIRECTION('ref_axis',(-0.969915897154534,-0.243440244098866,7.08310863902769E-31)) ;
#56974=DIRECTION('center_axis',(0.,0.,-1.)) ;
#56975=DIRECTION('ref_axis',(0.0966396842805139,0.995319431851987,0.)) ;
#56976=DIRECTION('center_axis',(0.,0.,-1.)) ;
#56977=DIRECTION('ref_axis',(0.0966396842805139,0.995319431851987,0.)) ;
#56978=DIRECTION('center_axis',(0.995319431851956,-0.0966396842808356,0.)) ;
#56979=DIRECTION('ref_axis',(0.,0.,1.)) ;
#56980=DIRECTION('',(0.,0.,1.)) ;
#56981=DIRECTION('',(0.,0.,-1.)) ;
#56982=DIRECTION('center_axis',(-0.995319431851989,0.0966396842804928,0.)) ;
#56983=DIRECTION('ref_axis',(0.068334576086459,0.703797119709238,0.707106781186593)) ;
#56984=DIRECTION('',(0.995319431851989,-0.0966396842804928,0.)) ;
#56985=DIRECTION('',(-0.995319431851989,0.0966396842804928,0.)) ;
#56986=DIRECTION('center_axis',(0.,0.,1.)) ;
#56987=DIRECTION('ref_axis',(-0.56271407713106,-0.826651599767725,0.)) ;
#56988=DIRECTION('center_axis',(0.,0.,1.)) ;
#56989=DIRECTION('ref_axis',(-0.562088660145462,-0.827076984407062,0.)) ;
#56990=DIRECTION('center_axis',(-0.995319431851989,0.0966396842804928,0.)) ;
#56991=DIRECTION('ref_axis',(-0.068334576086459,-0.703797119709238,-0.707106781186593)) ;
#56992=DIRECTION('',(-0.995319431851989,0.0966396842804928,0.)) ;
#56993=DIRECTION('',(0.,0.,-1.)) ;
#56994=DIRECTION('',(0.,0.,1.)) ;
#56995=DIRECTION('center_axis',(1.,0.,0.)) ;
#56996=DIRECTION('ref_axis',(0.,-0.707106781186561,0.707106781186534)) ;
#56997=DIRECTION('',(-1.,0.,0.)) ;
#56998=DIRECTION('',(1.,0.,0.)) ;
#56999=DIRECTION('center_axis',(1.,0.,0.)) ;
#57000=DIRECTION('ref_axis',(0.,0.707106781186561,-0.707106781186534)) ;
#57001=DIRECTION('',(1.,0.,0.)) ;
#57002=DIRECTION('center_axis',(0.,1.,0.)) ;
#57003=DIRECTION('ref_axis',(-1.,0.,0.)) ;
#57004=DIRECTION('center_axis',(0.,0.,1.)) ;
#57005=DIRECTION('ref_axis',(-1.,0.,0.)) ;
#57006=DIRECTION('center_axis',(-0.0966396842804928,-0.995319431851989,
0.)) ;
#57007=DIRECTION('ref_axis',(0.995319431851989,-0.0966396842804928,5.45822738711604E-33)) ;
#57008=DIRECTION('center_axis',(0.,0.,1.)) ;
#57009=DIRECTION('ref_axis',(-0.999001662609301,0.0446730131494725,0.)) ;
#57010=DIRECTION('center_axis',(0.0446052839665837,0.999004688999136,0.)) ;
#57011=DIRECTION('ref_axis',(0.999004688999136,-0.0446052839665837,0.)) ;
#57012=DIRECTION('center_axis',(0.,0.,-1.)) ;
#57013=DIRECTION('ref_axis',(0.575679505269549,0.81767542901362,0.)) ;
#57014=DIRECTION('center_axis',(0.,0.,1.)) ;
#57015=DIRECTION('ref_axis',(-0.56680837807234,-0.823849660160762,0.)) ;
#57016=DIRECTION('',(0.,0.,1.)) ;
#57017=DIRECTION('',(0.,0.,1.)) ;
#57018=DIRECTION('',(0.,0.,1.)) ;
#57019=DIRECTION('',(0.,0.,1.)) ;
#57020=DIRECTION('center_axis',(0.597732795757345,0.801695394071906,0.)) ;
#57021=DIRECTION('ref_axis',(-0.801695394071906,0.597732795757345,-4.49124931094878E-33)) ;
#57022=DIRECTION('',(0.801695394071906,-0.597732795757345,4.49124931094878E-33)) ;
#57023=DIRECTION('',(0.,0.,1.)) ;
#57024=DIRECTION('center_axis',(-0.338065775749409,-0.859650876406611,-0.383029896953615)) ;
#57025=DIRECTION('ref_axis',(-0.568856539673029,0.510881953775375,-0.644516769818974)) ;
#57026=DIRECTION('center_axis',(-0.202660578497202,0.979249043871464,4.76011490716992E-8)) ;
#57027=DIRECTION('ref_axis',(-0.979249043871465,-0.202660578497202,-8.65153100789119E-24)) ;
#57028=DIRECTION('center_axis',(0.,0.,-1.)) ;
#57029=DIRECTION('ref_axis',(0.0966396842805423,0.995319431851984,0.)) ;
#57030=DIRECTION('center_axis',(0.,0.,-1.)) ;
#57031=DIRECTION('ref_axis',(0.0966396842805423,0.995319431851984,0.)) ;
#57032=DIRECTION('center_axis',(-0.995319429345644,0.0966397100940514,0.)) ;
#57033=DIRECTION('ref_axis',(0.,0.,-1.)) ;
#57034=DIRECTION('center_axis',(-0.23112769823868,0.972923423043607,0.)) ;
#57035=DIRECTION('ref_axis',(0.,0.,-1.)) ;
#57036=DIRECTION('center_axis',(-0.503089999562018,0.864234026372885,0.)) ;
#57037=DIRECTION('ref_axis',(0.,0.,-1.)) ;
#57038=DIRECTION('center_axis',(-0.548205483816164,0.836343677870459,0.)) ;
#57039=DIRECTION('ref_axis',(0.,0.,-1.)) ;
#57040=DIRECTION('center_axis',(-0.809381734448836,0.587282902816516,0.)) ;
#57041=DIRECTION('ref_axis',(0.,0.,-1.)) ;
#57042=DIRECTION('center_axis',(-1.,0.,0.)) ;
#57043=DIRECTION('ref_axis',(0.,0.,-1.)) ;
#57044=DIRECTION('center_axis',(0.,0.,-1.)) ;
#57045=DIRECTION('ref_axis',(0.951152389067135,-0.308721772429289,0.)) ;
#57046=DIRECTION('center_axis',(-1.,0.,0.)) ;
#57047=DIRECTION('ref_axis',(0.,-0.707106781186561,-0.707106781186534)) ;
#57048=DIRECTION('center_axis',(-1.,0.,0.)) ;
#57049=DIRECTION('ref_axis',(0.,0.,-1.)) ;
#57050=DIRECTION('',(-1.,0.,0.)) ;
#57051=DIRECTION('center_axis',(0.707983649981651,-0.706228823653254,0.)) ;
#57052=DIRECTION('ref_axis',(0.,0.,-1.)) ;
#57053=DIRECTION('center_axis',(0.488003536616536,-0.872841651303232,0.)) ;
#57054=DIRECTION('ref_axis',(0.,0.,-1.)) ;
#57055=DIRECTION('center_axis',(0.124324416828667,-0.992241623487048,0.)) ;
#57056=DIRECTION('ref_axis',(0.,0.,-1.)) ;
#57057=DIRECTION('center_axis',(0.995319431851992,-0.096639684280469,0.)) ;
#57058=DIRECTION('ref_axis',(0.,0.,-1.)) ;
#57059=DIRECTION('center_axis',(0.995319431851989,-0.0966396842804928,0.)) ;
#57060=DIRECTION('ref_axis',(0.068334576086459,0.703797119709238,-0.707106781186593)) ;
#57061=DIRECTION('center_axis',(0.,-1.,0.)) ;
#57062=DIRECTION('ref_axis',(1.,0.,0.)) ;
#57063=DIRECTION('',(0.,0.,1.)) ;
#57064=DIRECTION('',(-7.24452218352468E-15,0.,-1.)) ;
#57065=DIRECTION('',(0.,0.,1.)) ;
#57066=DIRECTION('',(0.,0.,1.)) ;
#57067=DIRECTION('center_axis',(0.707106781186623,0.707106781186472,0.)) ;
#57068=DIRECTION('ref_axis',(-0.707106781186472,0.707106781186623,-1.01994663078385E-65)) ;
#57069=DIRECTION('',(-0.707106781186472,0.707106781186623,-1.01994663078385E-65)) ;
#57070=DIRECTION('',(0.,0.,-1.)) ;
#57071=DIRECTION('',(0.,0.,-1.)) ;
#57072=DIRECTION('',(0.,0.,1.)) ;
#57073=DIRECTION('',(0.,0.,-1.)) ;
#57074=DIRECTION('',(0.,0.,1.)) ;
#57075=DIRECTION('center_axis',(-0.0966396842804928,-0.995319431851989,
0.)) ;
#57076=DIRECTION('ref_axis',(0.995319431851989,-0.0966396842804928,5.45822738711604E-33)) ;
#57077=DIRECTION('',(0.,0.,-1.)) ;
#57078=DIRECTION('',(0.,0.,-1.)) ;
#57079=DIRECTION('center_axis',(0.,-1.,0.)) ;
#57080=DIRECTION('ref_axis',(1.,0.,0.)) ;
#57081=DIRECTION('center_axis',(1.,0.,0.)) ;
#57082=DIRECTION('ref_axis',(0.,1.,-7.30021430143246E-35)) ;
#57083=DIRECTION('',(0.,0.,1.)) ;
#57084=DIRECTION('center_axis',(-7.18398817372806E-49,4.73470448533E-50,
1.)) ;
#57085=DIRECTION('ref_axis',(-1.,-8.69145204082858E-115,-7.18398817372806E-49)) ;
#57086=DIRECTION('center_axis',(-1.09763027743844E-32,-3.07546720254364E-67,
1.)) ;
#57087=DIRECTION('ref_axis',(-1.,1.74482680966927E-115,-1.09763027743844E-32)) ;
#57088=DIRECTION('',(-0.992304006159154,0.123825519827269,-1.05251895471164E-32)) ;
#57089=DIRECTION('center_axis',(-0.123825519827269,-0.992304006159154,0.)) ;
#57090=DIRECTION('ref_axis',(0.992304006159154,-0.123825519827269,1.05251895471164E-32)) ;
#57091=DIRECTION('',(0.,0.,1.)) ;
#57092=DIRECTION('center_axis',(0.,0.,1.)) ;
#57093=DIRECTION('ref_axis',(-1.,0.,0.)) ;
#57094=DIRECTION('center_axis',(0.,0.,1.)) ;
#57095=DIRECTION('ref_axis',(-1.,0.,0.)) ;
#75311=CARTESIAN_POINT('',(0.,0.,0.)) ;
#75312=CARTESIAN_POINT('Ctrl Pts',(70.5067868147823,213.020459099211,23.9913203435596)) ;
#75313=CARTESIAN_POINT('Ctrl Pts',(70.5067452742029,213.0207906374,23.991193676059)) ;
#75314=CARTESIAN_POINT('Ctrl Pts',(70.506703653514,213.021122089189,23.9910669545086)) ;
#75315=CARTESIAN_POINT('Ctrl Pts',(70.4963561265166,213.102640079496,23.959944850052)) ;
#75316=CARTESIAN_POINT('Ctrl Pts',(70.4746411868221,213.183771458413,23.9281127081016)) ;
#75317=CARTESIAN_POINT('Ctrl Pts',(70.4402575595134,213.25405758073,23.9037686560088)) ;
#75318=CARTESIAN_POINT('Ctrl Pts',(70.5067868147823,213.020459099211,23.9913203435596)) ;
#75319=CARTESIAN_POINT('Ctrl Pts',(70.5067494667161,213.020757176667,23.9911502797591)) ;
#75320=CARTESIAN_POINT('Ctrl Pts',(70.5067013154789,213.021058548912,23.990983638255)) ;
#75321=CARTESIAN_POINT('Ctrl Pts',(70.4976711916085,213.094714614612,23.9494396875279)) ;
#75322=CARTESIAN_POINT('Ctrl Pts',(70.4671561080278,213.166896466404,23.9072539242599)) ;
#75323=CARTESIAN_POINT('Ctrl Pts',(70.4230475766717,213.224660710976,23.8845404570733)) ;
#75324=CARTESIAN_POINT('Ctrl Pts',(70.5067868147823,213.020459099211,23.9913203435596)) ;
#75325=CARTESIAN_POINT('Ctrl Pts',(70.5067533055873,213.020726538375,23.9911092906124)) ;
#75326=CARTESIAN_POINT('Ctrl Pts',(70.5067104186199,213.020993688966,23.9908979379349)) ;
#75327=CARTESIAN_POINT('Ctrl Pts',(70.4985845474206,213.086845209486,23.939048435049)) ;
#75328=CARTESIAN_POINT('Ctrl Pts',(70.4676741716718,213.150728655563,23.8858637118865)) ;
#75329=CARTESIAN_POINT('Ctrl Pts',(70.4200182523278,213.197323890113,23.8506292595553)) ;
#75330=CARTESIAN_POINT('Ctrl Pts',(70.5067868147823,213.020459099211,23.9913203435596)) ;
#75331=CARTESIAN_POINT('Ctrl Pts',(70.5067572623466,213.02069495921,23.9910670085588)) ;
#75332=CARTESIAN_POINT('Ctrl Pts',(70.5067275799083,213.020930748899,23.9908135654576)) ;
#75333=CARTESIAN_POINT('Ctrl Pts',(70.4992716079751,213.078911615354,23.928569356544)) ;
#75334=CARTESIAN_POINT('Ctrl Pts',(70.4754045229177,213.13557710162,23.8649050726435)) ;
#75335=CARTESIAN_POINT('Ctrl Pts',(70.4324364715585,213.183479571871,23.816216968458)) ;
#75336=CARTESIAN_POINT('',(70.4324364715585,213.183479571871,23.816216968458)) ;
#75337=CARTESIAN_POINT('',(70.4402575591012,213.254057580026,23.9037686555483)) ;
#75338=CARTESIAN_POINT('Origin',(70.5217653290874,213.263606690954,23.816216968458)) ;
#75339=CARTESIAN_POINT('',(70.5064330146391,213.023239669833,23.9902583635613)) ;
#75340=CARTESIAN_POINT('Ctrl Pts',(70.4402575595134,213.25405758073,23.9037686560088)) ;
#75341=CARTESIAN_POINT('Ctrl Pts',(70.4743890527587,213.184286864349,23.9279341939291)) ;
#75342=CARTESIAN_POINT('Ctrl Pts',(70.4960369753435,213.103829364047,23.9594784045025)) ;
#75343=CARTESIAN_POINT('Ctrl Pts',(70.5064330146391,213.023239669833,23.9902583635613)) ;
#75344=CARTESIAN_POINT('',(70.5067868147824,213.020459099211,23.9913203435596)) ;
#75345=CARTESIAN_POINT('Ctrl Pts',(70.5064330146391,213.023239669833,23.9902583635613)) ;
#75346=CARTESIAN_POINT('Ctrl Pts',(70.5065098116199,213.022644342611,23.9904857393779)) ;
#75347=CARTESIAN_POINT('Ctrl Pts',(70.5065859945876,213.022049008174,23.9907130734895)) ;
#75348=CARTESIAN_POINT('Ctrl Pts',(70.506703653514,213.021122089189,23.9910669545086)) ;
#75349=CARTESIAN_POINT('Ctrl Pts',(70.5067452742029,213.0207906374,23.991193676059)) ;
#75350=CARTESIAN_POINT('Ctrl Pts',(70.5067868147823,213.020459099211,23.9913203435596)) ;
#75351=CARTESIAN_POINT('Ctrl Pts',(70.5067868147823,213.020459099211,23.9913203435596)) ;
#75352=CARTESIAN_POINT('Ctrl Pts',(70.5067572623466,213.02069495921,23.9910670085588)) ;
#75353=CARTESIAN_POINT('Ctrl Pts',(70.5067275799083,213.020930748899,23.9908135654576)) ;
#75354=CARTESIAN_POINT('Ctrl Pts',(70.4992716079751,213.078911615354,23.928569356544)) ;
#75355=CARTESIAN_POINT('Ctrl Pts',(70.4754045229177,213.13557710162,23.8649050726435)) ;
#75356=CARTESIAN_POINT('Ctrl Pts',(70.4324364715585,213.183479571871,23.816216968458)) ;
#75357=CARTESIAN_POINT('Ctrl Pts',(70.3430483908416,213.381234213224,23.8713203435596)) ;
#75358=CARTESIAN_POINT('Ctrl Pts',(70.3128258349002,213.391402788884,23.8713203435596)) ;
#75359=CARTESIAN_POINT('Ctrl Pts',(70.281441089983,213.398114352515,23.8713203435596)) ;
#75360=CARTESIAN_POINT('Ctrl Pts',(70.249702995134,213.401195935541,23.8713203435596)) ;
#75361=CARTESIAN_POINT('Ctrl Pts',(70.3315989685636,213.347204786009,23.8713203435596)) ;
#75362=CARTESIAN_POINT('Ctrl Pts',(70.3039711975011,213.356500329407,23.8713203435596)) ;
#75363=CARTESIAN_POINT('Ctrl Pts',(70.2752464440296,213.362643059298,23.8713203435596)) ;
#75364=CARTESIAN_POINT('Ctrl Pts',(70.2462332520234,213.365460070225,23.8713203435596)) ;
#75365=CARTESIAN_POINT('Ctrl Pts',(70.3117855159125,213.288316186349,23.8411618094987)) ;
#75366=CARTESIAN_POINT('Ctrl Pts',(70.2886148214212,213.296112117325,23.8411618094987)) ;
#75367=CARTESIAN_POINT('Ctrl Pts',(70.2645614037344,213.301255891594,23.8411618094987)) ;
#75368=CARTESIAN_POINT('Ctrl Pts',(70.2402287926573,213.303618445541,23.8411618094987)) ;
#75369=CARTESIAN_POINT('Ctrl Pts',(70.3047815156687,213.267499230635,23.7782482805904)) ;
#75370=CARTESIAN_POINT('Ctrl Pts',(70.2832009937725,213.274760137691,23.7782482805904)) ;
#75371=CARTESIAN_POINT('Ctrl Pts',(70.2607689307802,213.279557188569,23.7782482805904)) ;
#75372=CARTESIAN_POINT('Ctrl Pts',(70.2381062330204,213.281757603718,23.7782482805904)) ;
#75373=CARTESIAN_POINT('Ctrl Pts',(70.3047815156687,213.267499230635,23.7513203435596)) ;
#75374=CARTESIAN_POINT('Ctrl Pts',(70.2831939757105,213.274762498963,23.7513203435596)) ;
#75375=CARTESIAN_POINT('Ctrl Pts',(70.2607763007697,213.279556472986,23.7513203435596)) ;
#75376=CARTESIAN_POINT('Ctrl Pts',(70.2381062330204,213.281757603718,23.7513203435596)) ;
#75377=CARTESIAN_POINT('',(70.2381062330204,213.281757603718,23.7513203435596)) ;
#75378=CARTESIAN_POINT('',(70.249702995134,213.401195935541,23.8713203435596)) ;
#75379=CARTESIAN_POINT('Origin',(70.249702995134,213.401195935541,23.7513203435596)) ;
#75380=CARTESIAN_POINT('',(70.343048519498,213.381234190268,23.8713203435596)) ;
#75381=CARTESIAN_POINT('Origin',(70.2090187857755,212.982714998987,23.8713203435596)) ;
#75382=CARTESIAN_POINT('',(70.3047803801335,213.267495861574,23.7513203435596)) ;
#75383=CARTESIAN_POINT('Origin',(70.3430483908416,213.381234213224,23.7513203435596)) ;
#75384=CARTESIAN_POINT('Origin',(70.2090460834845,212.982842649052,23.7513203435596)) ;
#75385=CARTESIAN_POINT('Origin',(69.2693585135591,213.496381639902,23.7513203435596)) ;
#75386=CARTESIAN_POINT('',(60.9673257563026,214.181896061416,23.7513203435596)) ;
#75387=CARTESIAN_POINT('',(60.9789225184162,214.301334393238,23.8713203435596)) ;
#75388=CARTESIAN_POINT('Origin',(60.9789225184162,214.301334393238,23.7513203435596)) ;
#75389=CARTESIAN_POINT('',(69.2693585135591,213.496381639902,23.8713203435596)) ;
#75390=CARTESIAN_POINT('',(69.2577617514454,213.37694330808,23.7513203435596)) ;
#75391=CARTESIAN_POINT('Ctrl Pts',(60.8382191089244,214.038138460174,23.7513203435596)) ;
#75392=CARTESIAN_POINT('Ctrl Pts',(60.8349680037942,214.053847689931,23.7513203435596)) ;
#75393=CARTESIAN_POINT('Ctrl Pts',(60.8347810847976,214.092067656972,23.7513203435596)) ;
#75394=CARTESIAN_POINT('Ctrl Pts',(60.8596053972971,214.141559512008,23.7513203435596)) ;
#75395=CARTESIAN_POINT('Ctrl Pts',(60.9078636356518,214.177314552193,23.7513203435596)) ;
#75396=CARTESIAN_POINT('Ctrl Pts',(60.9460363791904,214.183963135178,23.7513203435596)) ;
#75397=CARTESIAN_POINT('Ctrl Pts',(60.9673257563026,214.181896061416,23.7513203435596)) ;
#75398=CARTESIAN_POINT('Ctrl Pts',(60.8382191089244,214.038138460174,23.7872242596007)) ;
#75399=CARTESIAN_POINT('Ctrl Pts',(60.8349783938156,214.0537974857,23.7872242596007)) ;
#75400=CARTESIAN_POINT('Ctrl Pts',(60.8348926282557,214.092007322074,23.7872242596007)) ;
#75401=CARTESIAN_POINT('Ctrl Pts',(60.8597441877997,214.141459678259,23.7872242596007)) ;
#75402=CARTESIAN_POINT('Ctrl Pts',(60.9079021315186,214.177160517204,23.7872242596007)) ;
#75403=CARTESIAN_POINT('Ctrl Pts',(60.9461044166959,214.183956529135,23.7872242596007)) ;
#75404=CARTESIAN_POINT('Ctrl Pts',(60.9673257563026,214.181896061416,23.7872242596007)) ;
#75405=CARTESIAN_POINT('Ctrl Pts',(60.8086864986605,214.032026536023,23.8493568285239)) ;
#75406=CARTESIAN_POINT('Ctrl Pts',(60.8046159279154,214.051695395846,23.8493568285239)) ;
#75407=CARTESIAN_POINT('Ctrl Pts',(60.8043586945544,214.099523150747,23.8493568285239)) ;
#75408=CARTESIAN_POINT('Ctrl Pts',(60.8354155723799,214.161462422765,23.8493568285239)) ;
#75409=CARTESIAN_POINT('Ctrl Pts',(60.8958252215348,214.206215932689,23.8493568285239)) ;
#75410=CARTESIAN_POINT('Ctrl Pts',(60.9435847316276,214.214501424618,23.8493568285239)) ;
#75411=CARTESIAN_POINT('Ctrl Pts',(60.9702402571129,214.211913329294,23.8493568285239)) ;
#75412=CARTESIAN_POINT('Ctrl Pts',(60.7470783802507,214.01927642205,23.8713203435596)) ;
#75413=CARTESIAN_POINT('Ctrl Pts',(60.741304223938,214.047176949573,23.8713203435596)) ;
#75414=CARTESIAN_POINT('Ctrl Pts',(60.7409578016198,214.115041798193,23.8713203435596)) ;
#75415=CARTESIAN_POINT('Ctrl Pts',(60.7850319503784,214.202925235258,23.8713203435596)) ;
#75416=CARTESIAN_POINT('Ctrl Pts',(60.8707337092228,214.266419688393,23.8713203435596)) ;
#75417=CARTESIAN_POINT('Ctrl Pts',(60.9385090095622,214.278203740347,23.8713203435596)) ;
#75418=CARTESIAN_POINT('Ctrl Pts',(60.9763202110832,214.274532494252,23.8713203435596)) ;
#75419=CARTESIAN_POINT('Ctrl Pts',(60.7207092236599,214.013819190754,23.8713203435596)) ;
#75420=CARTESIAN_POINT('Ctrl Pts',(60.7142070133995,214.045237650267,23.8713203435596)) ;
#75421=CARTESIAN_POINT('Ctrl Pts',(60.7138331754062,214.12167758435,23.8713203435596)) ;
#75422=CARTESIAN_POINT('Ctrl Pts',(60.7634818004053,214.220661294423,23.8713203435596)) ;
#75423=CARTESIAN_POINT('Ctrl Pts',(60.8599982771146,214.292171374792,23.8713203435596)) ;
#75424=CARTESIAN_POINT('Ctrl Pts',(60.9363437641918,214.305468540763,23.8713203435596)) ;
#75425=CARTESIAN_POINT('Ctrl Pts',(60.9789225184162,214.301334393238,23.8713203435596)) ;
#75426=CARTESIAN_POINT('',(60.8382191089243,214.038138460174,23.7513203435596)) ;
#75427=CARTESIAN_POINT('',(60.7964818927896,214.241986587567,23.8713203435593)) ;
#75428=CARTESIAN_POINT('Ctrl Pts',(60.8382191089244,214.038138460174,23.7513203435598)) ;
#75429=CARTESIAN_POINT('Ctrl Pts',(60.838173023382,214.038361143952,23.7515407958386)) ;
#75430=CARTESIAN_POINT('Ctrl Pts',(60.8381269353183,214.03858384766,23.7517613397707)) ;
#75431=CARTESIAN_POINT('Ctrl Pts',(60.832437970542,214.066074644562,23.7789935900481)) ;
#75432=CARTESIAN_POINT('Ctrl Pts',(60.8266291834655,214.094252337735,23.8078858434553)) ;
#75433=CARTESIAN_POINT('Ctrl Pts',(60.8172426770213,214.140025265548,23.8402029453431)) ;
#75434=CARTESIAN_POINT('Ctrl Pts',(60.8134587671683,214.158506292337,23.8514672560685)) ;
#75435=CARTESIAN_POINT('Ctrl Pts',(60.8048771688427,214.20059701627,23.8670015141976)) ;
#75436=CARTESIAN_POINT('Ctrl Pts',(60.8006691257539,214.221299002739,23.871320410552)) ;
#75437=CARTESIAN_POINT('Ctrl Pts',(60.7964789537465,214.24198307187,23.8713203435588)) ;
#75438=CARTESIAN_POINT('Ctrl Pts',(60.7964883386305,214.241990816335,23.8713203435596)) ;
#75439=CARTESIAN_POINT('Ctrl Pts',(60.8137096104711,214.257238073522,23.8713203435596)) ;
#75440=CARTESIAN_POINT('Ctrl Pts',(60.869265568141,214.293785467669,23.8713203435596)) ;
#75441=CARTESIAN_POINT('Ctrl Pts',(60.9363437641918,214.305468540763,23.8713203435596)) ;
#75442=CARTESIAN_POINT('Ctrl Pts',(60.9789225184162,214.301334393238,23.8713203435596)) ;
#75443=CARTESIAN_POINT('Ctrl Pts',(60.9673257563026,214.181896061416,23.7513203435596)) ;
#75444=CARTESIAN_POINT('Ctrl Pts',(60.9300677412812,214.185513596343,23.7513203435596)) ;
#75445=CARTESIAN_POINT('Ctrl Pts',(60.8750422973704,214.163785096389,23.7513203435596)) ;
#75446=CARTESIAN_POINT('Ctrl Pts',(60.8364976384102,214.097504784634,23.7513203435596)) ;
#75447=CARTESIAN_POINT('Ctrl Pts',(60.8338841153326,214.059085002227,23.7513203435596)) ;
#75448=CARTESIAN_POINT('Ctrl Pts',(60.8382191089243,214.038138460174,23.7513203435596)) ;
#75449=CARTESIAN_POINT('Ctrl Pts',(70.4402575595134,213.25405758073,23.9037686560088)) ;
#75450=CARTESIAN_POINT('Ctrl Pts',(70.4293130460961,213.276430072202,23.8960197991948)) ;
#75451=CARTESIAN_POINT('Ctrl Pts',(70.400744289201,213.326037220728,23.8797940397281)) ;
#75452=CARTESIAN_POINT('Ctrl Pts',(70.364672058518,213.365172858634,23.8713203435596)) ;
#75453=CARTESIAN_POINT('Ctrl Pts',(70.3430483908423,213.381234213224,23.8713203435596)) ;
#75454=CARTESIAN_POINT('Ctrl Pts',(70.4304232836038,213.237259369442,23.8927811137599)) ;
#75455=CARTESIAN_POINT('Ctrl Pts',(70.4177874014361,213.257356621761,23.8853350385388)) ;
#75456=CARTESIAN_POINT('Ctrl Pts',(70.3853635668498,213.301250711437,23.8712650795695)) ;
#75457=CARTESIAN_POINT('Ctrl Pts',(70.3501402667773,213.333862218516,23.8687526857235)) ;
#75458=CARTESIAN_POINT('Ctrl Pts',(70.3315989685643,213.347204786009,23.8713203435596)) ;
#75459=CARTESIAN_POINT('Ctrl Pts',(70.4208736085904,213.208806061158,23.8653880989702)) ;
#75460=CARTESIAN_POINT('Ctrl Pts',(70.4061885733414,213.225063832397,23.8559692034752)) ;
#75461=CARTESIAN_POINT('Ctrl Pts',(70.3684654232861,213.259117705828,23.8385706022235)) ;
#75462=CARTESIAN_POINT('Ctrl Pts',(70.3300695353271,213.280024504393,23.8372025575081)) ;
#75463=CARTESIAN_POINT('Ctrl Pts',(70.3117855159529,213.288316186467,23.8411618093945)) ;
#75464=CARTESIAN_POINT('Ctrl Pts',(70.4271143776025,213.189412851118,23.8309650932139)) ;
#75465=CARTESIAN_POINT('Ctrl Pts',(70.4128585336131,213.204484036889,23.8172879160337)) ;
#75466=CARTESIAN_POINT('Ctrl Pts',(70.3754254077714,213.236754374851,23.7893499112497)) ;
#75467=CARTESIAN_POINT('Ctrl Pts',(70.3304143111952,213.258897564795,23.7770689833929)) ;
#75468=CARTESIAN_POINT('Ctrl Pts',(70.3047815156691,213.267499230635,23.7782482805904)) ;
#75469=CARTESIAN_POINT('Ctrl Pts',(70.4324364715585,213.183479571871,23.816216968458)) ;
#75470=CARTESIAN_POINT('Ctrl Pts',(70.4187594848231,213.198727213537,23.80071925483)) ;
#75471=CARTESIAN_POINT('Ctrl Pts',(70.3822800164705,213.232206696606,23.7682677358966)) ;
#75472=CARTESIAN_POINT('Ctrl Pts',(70.3342045609418,213.257599655543,23.7513203435596)) ;
#75473=CARTESIAN_POINT('Ctrl Pts',(70.3047815156691,213.267499230635,23.7513203435596)) ;
#75474=CARTESIAN_POINT('Ctrl Pts',(70.3430484847436,213.381234143477,23.8713203435596)) ;
#75475=CARTESIAN_POINT('Ctrl Pts',(70.3646721181921,213.365172793892,23.8713203575776)) ;
#75476=CARTESIAN_POINT('Ctrl Pts',(70.4007443128316,213.326037179696,23.8797940531492)) ;
#75477=CARTESIAN_POINT('Ctrl Pts',(70.4293130460961,213.276430072202,23.8960197991948)) ;
#75478=CARTESIAN_POINT('Ctrl Pts',(70.4402575595134,213.25405758073,23.9037686560088)) ;
#75479=CARTESIAN_POINT('Ctrl Pts',(70.4322999468881,213.183358207456,23.8162169311491)) ;
#75480=CARTESIAN_POINT('Ctrl Pts',(70.4234535753444,213.193304216735,23.8061394650786)) ;
#75481=CARTESIAN_POINT('Ctrl Pts',(70.4137714926804,213.202867974732,23.7967342679728)) ;
#75482=CARTESIAN_POINT('Ctrl Pts',(70.4031984556939,213.211886624186,23.7883471637087)) ;
#75483=CARTESIAN_POINT('Ctrl Pts',(70.4010445153906,213.213723904484,23.7866385418695)) ;
#75484=CARTESIAN_POINT('Ctrl Pts',(70.3988535830009,213.215538390765,23.7849721728023)) ;
#75485=CARTESIAN_POINT('Ctrl Pts',(70.3966251713264,213.217328431485,23.7833509803679)) ;
#75486=CARTESIAN_POINT('Ctrl Pts',(70.3929701868672,213.220264410992,23.7806919415464)) ;
#75487=CARTESIAN_POINT('Ctrl Pts',(70.3892143573437,213.223134648899,23.7781544356857)) ;
#75488=CARTESIAN_POINT('Ctrl Pts',(70.3853580260576,213.225933855895,23.7757513638946)) ;
#75489=CARTESIAN_POINT('Ctrl Pts',(70.3751864666561,213.233317116854,23.7694129594228)) ;
#75490=CARTESIAN_POINT('Ctrl Pts',(70.364316085825,213.240200699965,23.7640098222587)) ;
#75491=CARTESIAN_POINT('Ctrl Pts',(70.3528777612805,213.246426228203,23.7599089338264)) ;
#75492=CARTESIAN_POINT('Ctrl Pts',(70.3412021188436,213.252780921271,23.7557229617618)) ;
#75493=CARTESIAN_POINT('Ctrl Pts',(70.3289354346888,213.258449285322,23.752893836096)) ;
#75494=CARTESIAN_POINT('Ctrl Pts',(70.3162582762205,213.263297580557,23.7518118574086)) ;
#75495=CARTESIAN_POINT('Ctrl Pts',(70.3124600132869,213.264750201042,23.7514876806971)) ;
#75496=CARTESIAN_POINT('Ctrl Pts',(70.308625136255,213.266129475579,23.7513203435596)) ;
#75497=CARTESIAN_POINT('Ctrl Pts',(70.3047590365879,213.267432536623,23.7513203435596)) ;
#75498=CARTESIAN_POINT('Origin',(69.2569276623894,213.37702429324,23.8713203435596)) ;
#75499=CARTESIAN_POINT('',(70.2381062330204,213.281757603718,17.9913203435596)) ;
#75500=CARTESIAN_POINT('',(70.2381062330204,213.281757603718,17.9913203435596)) ;
#75501=CARTESIAN_POINT('',(60.9673257563026,214.181896061416,17.9913203435596)) ;
#75502=CARTESIAN_POINT('',(67.5441762598793,213.543322417734,17.9913203435596)) ;
#75503=CARTESIAN_POINT('',(60.9673257563026,214.181896061416,23.7513203435596)) ;
#75504=CARTESIAN_POINT('Ctrl Pts',(70.5067868147823,213.020459099211,23.9913203435596)) ;
#75505=CARTESIAN_POINT('Ctrl Pts',(70.5067868147823,213.020459099211,16.7913203435596)) ;
#75506=CARTESIAN_POINT('Ctrl Pts',(70.4972006303894,213.096967088613,23.9913203435596)) ;
#75507=CARTESIAN_POINT('Ctrl Pts',(70.4972006303894,213.096967088613,16.7913203435596)) ;
#75508=CARTESIAN_POINT('Ctrl Pts',(70.4262160126144,213.22323691339,23.9913203435596)) ;
#75509=CARTESIAN_POINT('Ctrl Pts',(70.4262160126144,213.22323691339,16.7913203435596)) ;
#75510=CARTESIAN_POINT('Ctrl Pts',(70.2956652136715,213.276168963992,23.9913203435596)) ;
#75511=CARTESIAN_POINT('Ctrl Pts',(70.2956652136715,213.276168963992,16.7913203435596)) ;
#75512=CARTESIAN_POINT('Ctrl Pts',(70.2381062330204,213.281757603718,23.9913203435596)) ;
#75513=CARTESIAN_POINT('Ctrl Pts',(70.2381062330204,213.281757603718,16.7913203435596)) ;
#75514=CARTESIAN_POINT('',(70.5067868147823,213.020459099211,17.9913203435596)) ;
#75515=CARTESIAN_POINT('',(70.5067868147823,213.020459099211,23.9913203435596)) ;
#75516=CARTESIAN_POINT('Ctrl Pts',(70.2381062330204,213.281757603718,17.9913203435596)) ;
#75517=CARTESIAN_POINT('Ctrl Pts',(70.2956652136715,213.276168963992,17.9913203435596)) ;
#75518=CARTESIAN_POINT('Ctrl Pts',(70.4262160126144,213.22323691339,17.9913203435596)) ;
#75519=CARTESIAN_POINT('Ctrl Pts',(70.4972006303894,213.096967088613,17.9913203435596)) ;
#75520=CARTESIAN_POINT('Ctrl Pts',(70.5067868147823,213.020459099211,17.9913203435596)) ;
#75521=CARTESIAN_POINT('Ctrl Pts',(70.4779346423502,213.258471670562,23.9913203435596)) ;
#75522=CARTESIAN_POINT('Ctrl Pts',(70.4872340585151,213.179095199652,23.9913203435596)) ;
#75523=CARTESIAN_POINT('Ctrl Pts',(70.4968510871259,213.099756817164,23.9913203435596)) ;
#75524=CARTESIAN_POINT('Ctrl Pts',(70.5067868147824,213.020459099211,23.9913203435596)) ;
#75525=CARTESIAN_POINT('Ctrl Pts',(70.4779346423502,213.258471670562,23.9586110212513)) ;
#75526=CARTESIAN_POINT('Ctrl Pts',(70.4872340122281,213.179095594742,23.9586110212513)) ;
#75527=CARTESIAN_POINT('Ctrl Pts',(70.4968511367978,213.099756420729,23.9586110212512)) ;
#75528=CARTESIAN_POINT('Ctrl Pts',(70.5067868147824,213.020459099211,23.9586110212512)) ;
#75529=CARTESIAN_POINT('Ctrl Pts',(70.4639600858961,213.256834469831,23.9261378065485)) ;
#75530=CARTESIAN_POINT('Ctrl Pts',(70.4732638269676,213.177421083075,23.9261378065485)) ;
#75531=CARTESIAN_POINT('Ctrl Pts',(70.4828854739267,213.098044597579,23.9261378065485)) ;
#75532=CARTESIAN_POINT('Ctrl Pts',(70.4928258427598,213.01870983808,23.9261378065485)) ;
#75533=CARTESIAN_POINT('Ctrl Pts',(70.4402575595134,213.25405758073,23.9037686560088)) ;
#75534=CARTESIAN_POINT('Ctrl Pts',(70.4495687541354,213.174580573148,23.9037686560088)) ;
#75535=CARTESIAN_POINT('Ctrl Pts',(70.4591979897609,213.095141478033,23.9037686560088)) ;
#75536=CARTESIAN_POINT('Ctrl Pts',(70.4691463572047,213.015742881078,23.9037686560088)) ;
#75537=CARTESIAN_POINT('',(70.4779346423502,213.258471670562,23.9913203435596)) ;
#75538=CARTESIAN_POINT('Origin',(70.3587497899394,213.244508470506,23.9913203435596)) ;
#75539=CARTESIAN_POINT('Origin',(97.0052522373154,221.373828808523,23.9913203435596)) ;
#75540=CARTESIAN_POINT('Ctrl Pts',(70.2813572214291,216.003852832275,23.9913203435596)) ;
#75541=CARTESIAN_POINT('Ctrl Pts',(70.3063010559943,215.086315128482,23.9913203435596)) ;
#75542=CARTESIAN_POINT('Ctrl Pts',(70.3711537499325,214.169914953712,23.9913203435596)) ;
#75543=CARTESIAN_POINT('Ctrl Pts',(70.4779346423502,213.258471670562,23.9913203435596)) ;
#75544=CARTESIAN_POINT('Ctrl Pts',(70.2813572214291,216.003852832275,23.9554164275186)) ;
#75545=CARTESIAN_POINT('Ctrl Pts',(70.3063007540173,215.086326236448,23.9554164275186)) ;
#75546=CARTESIAN_POINT('Ctrl Pts',(70.3711551172063,214.169903283155,23.9554164275186)) ;
#75547=CARTESIAN_POINT('Ctrl Pts',(70.4779346423502,213.258471670562,23.9554164275186)) ;
#75548=CARTESIAN_POINT('Ctrl Pts',(70.2512097926781,216.003033255628,23.8932840272914)) ;
#75549=CARTESIAN_POINT('Ctrl Pts',(70.2761774443025,215.084619461598,23.8932840272914)) ;
#75550=CARTESIAN_POINT('Ctrl Pts',(70.3410922094225,214.167326164876,23.8932840272914)) ;
#75551=CARTESIAN_POINT('Ctrl Pts',(70.4479809393324,213.254962419687,23.8932840272914)) ;
#75552=CARTESIAN_POINT('Ctrl Pts',(70.1883195322401,216.001323544685,23.8713203435596)) ;
#75553=CARTESIAN_POINT('Ctrl Pts',(70.2133366971056,215.081088448267,23.8713203435596)) ;
#75554=CARTESIAN_POINT('Ctrl Pts',(70.2783818952035,214.161919097311,23.8713203435596)) ;
#75555=CARTESIAN_POINT('Ctrl Pts',(70.3854948082789,213.247641805271,23.8713203435596)) ;
#75556=CARTESIAN_POINT('Ctrl Pts',(70.1614015403525,216.000591762292,23.8713203435596)) ;
#75557=CARTESIAN_POINT('Ctrl Pts',(70.1864398654763,215.079578303801,23.8713203435596)) ;
#75558=CARTESIAN_POINT('Ctrl Pts',(70.2515410686805,214.159603546732,23.8713203435596)) ;
#75559=CARTESIAN_POINT('Ctrl Pts',(70.3587497899394,213.244508470506,23.8713203435596)) ;
#75560=CARTESIAN_POINT('',(70.1614015403524,216.000591762293,23.8713203435596)) ;
#75561=CARTESIAN_POINT('Origin',(97.3863035375064,222.371901130348,23.8713203435596)) ;
#75562=CARTESIAN_POINT('',(70.2813572214291,216.003852832276,23.9913203435596)) ;
#75563=CARTESIAN_POINT('Origin',(70.1614015403524,216.000591762293,23.9913203435596)) ;
#75564=CARTESIAN_POINT('Origin',(97.5077297430571,222.403214886601,23.9913203435596)) ;
#75565=CARTESIAN_POINT('Ctrl Pts',(73.7436956568154,200.410454788892,30.2513203435596)) ;
#75566=CARTESIAN_POINT('Ctrl Pts',(75.7987505865357,196.993517189618,30.2513203435596)) ;
#75567=CARTESIAN_POINT('Ctrl Pts',(78.3337590639418,193.889658425843,30.2513203435596)) ;
#75568=CARTESIAN_POINT('Ctrl Pts',(81.068251094894,190.995574215667,30.2513203435596)) ;
#75569=CARTESIAN_POINT('Ctrl Pts',(73.7436956568154,200.410454788892,30.2872242596007)) ;
#75570=CARTESIAN_POINT('Ctrl Pts',(75.7987702584097,196.993484481214,30.2872242596007)) ;
#75571=CARTESIAN_POINT('Ctrl Pts',(78.3337453944066,193.889672893168,30.2872242596007)) ;
#75572=CARTESIAN_POINT('Ctrl Pts',(81.068251094894,190.995574215667,30.2872242596007)) ;
#75573=CARTESIAN_POINT('Ctrl Pts',(73.769540015645,200.425998408134,30.3493567430526)) ;
#75574=CARTESIAN_POINT('Ctrl Pts',(75.8230434158966,197.011640535222,30.3493567430526)) ;
#75575=CARTESIAN_POINT('Ctrl Pts',(78.3567583097309,193.909229680419,30.3493567430526)) ;
#75576=CARTESIAN_POINT('Ctrl Pts',(81.0901722183543,191.016286514639,30.3493567430526)) ;
#75577=CARTESIAN_POINT('Ctrl Pts',(73.8234538668466,200.45842391269,30.3713203435596)) ;
#75578=CARTESIAN_POINT('Ctrl Pts',(75.8737317953243,197.049429028193,30.3713203435596)) ;
#75579=CARTESIAN_POINT('Ctrl Pts',(78.4047292161471,193.9500654395,30.3713203435596)) ;
#75580=CARTESIAN_POINT('Ctrl Pts',(81.1359018182332,191.059494388828,30.3713203435596)) ;
#75581=CARTESIAN_POINT('Ctrl Pts',(73.8465297930579,200.47230250852,30.3713203435596)) ;
#75582=CARTESIAN_POINT('Ctrl Pts',(75.8954292657049,197.065599581035,30.3713203435596)) ;
#75583=CARTESIAN_POINT('Ctrl Pts',(78.4252600190873,193.9675452886,30.3713203435596)) ;
#75584=CARTESIAN_POINT('Ctrl Pts',(81.1554747637557,191.077987998436,30.3713203435596)) ;
#75585=CARTESIAN_POINT('',(81.068251094894,190.995574215667,30.2513203435596)) ;
#75586=CARTESIAN_POINT('',(81.1554747637557,191.077987998436,30.3713203435596)) ;
#75587=CARTESIAN_POINT('Origin',(81.1554747637557,191.077987998436,30.2513203435596)) ;
#75588=CARTESIAN_POINT('',(73.8465297930579,200.47230250852,30.3713203435596)) ;
#75589=CARTESIAN_POINT('Ctrl Pts',(81.1554747637557,191.077987998436,30.3713203435596)) ;
#75590=CARTESIAN_POINT('Ctrl Pts',(78.4252600190873,193.9675452886,30.3713203435596)) ;
#75591=CARTESIAN_POINT('Ctrl Pts',(75.8954292657049,197.065599581035,30.3713203435596)) ;
#75592=CARTESIAN_POINT('Ctrl Pts',(73.8465297930579,200.47230250852,30.3713203435596)) ;
#75593=CARTESIAN_POINT('',(73.7436956568154,200.410454788892,30.2513203435596)) ;
#75594=CARTESIAN_POINT('Origin',(73.8465297930579,200.47230250852,30.2513203435596)) ;
#75595=CARTESIAN_POINT('Ctrl Pts',(73.7436956568154,200.410454788892,30.2513203435596)) ;
#75596=CARTESIAN_POINT('Ctrl Pts',(75.7987505865357,196.993517189618,30.2513203435596)) ;
#75597=CARTESIAN_POINT('Ctrl Pts',(78.3337590639418,193.889658425843,30.2513203435596)) ;
#75598=CARTESIAN_POINT('Ctrl Pts',(81.068251094894,190.995574215667,30.2513203435596)) ;
#75599=CARTESIAN_POINT('Ctrl Pts',(80.8501919227397,190.369539758744,30.3713203435596)) ;
#75600=CARTESIAN_POINT('Ctrl Pts',(80.989856244946,190.369539758744,30.3713203435596)) ;
#75601=CARTESIAN_POINT('Ctrl Pts',(81.2186255309631,190.49593104996,30.3713203435596)) ;
#75602=CARTESIAN_POINT('Ctrl Pts',(81.299864395013,190.831780335431,30.3713203435596)) ;
#75603=CARTESIAN_POINT('Ctrl Pts',(81.2194206810384,191.01031002848,30.3713203435596)) ;
#75604=CARTESIAN_POINT('Ctrl Pts',(81.1554747637557,191.077987998436,30.3713203435596)) ;
#75605=CARTESIAN_POINT('Ctrl Pts',(80.8501919227397,190.405443674785,30.3713203435596)) ;
#75606=CARTESIAN_POINT('Ctrl Pts',(80.9778652382259,190.405443674785,30.3713203435596)) ;
#75607=CARTESIAN_POINT('Ctrl Pts',(81.1870720669225,190.521166083618,30.3713203435596)) ;
#75608=CARTESIAN_POINT('Ctrl Pts',(81.2613364057291,190.82818145774,30.3713203435596)) ;
#75609=CARTESIAN_POINT('Ctrl Pts',(81.1878332857695,190.991462435668,30.3713203435596)) ;
#75610=CARTESIAN_POINT('Ctrl Pts',(81.129377503059,191.053329852293,30.3713203435596)) ;
#75611=CARTESIAN_POINT('Ctrl Pts',(80.8501919227397,190.467576190064,30.3411618724029)) ;
#75612=CARTESIAN_POINT('Ctrl Pts',(80.9572682185845,190.467576190064,30.3411618724029)) ;
#75613=CARTESIAN_POINT('Ctrl Pts',(81.1326396018592,190.564432599516,30.3411618724029)) ;
#75614=CARTESIAN_POINT('Ctrl Pts',(81.1949228397646,190.821917634261,30.3411618724029)) ;
#75615=CARTESIAN_POINT('Ctrl Pts',(81.1332409679373,190.958771792307,30.3411618724029)) ;
#75616=CARTESIAN_POINT('Ctrl Pts',(81.0842156202403,191.010658388817,30.3411618724029)) ;
#75617=CARTESIAN_POINT('Ctrl Pts',(80.8501919227397,190.489539758744,30.2782482805904)) ;
#75618=CARTESIAN_POINT('Ctrl Pts',(80.9499197210544,190.489539758744,30.2782482805904)) ;
#75619=CARTESIAN_POINT('Ctrl Pts',(81.1133225940155,190.579904354768,30.2782482805904)) ;
#75620=CARTESIAN_POINT('Ctrl Pts',(81.1713316842795,190.819719172513,30.2782482805904)) ;
#75621=CARTESIAN_POINT('Ctrl Pts',(81.1139119010403,190.947248524242,30.2782482805904)) ;
#75622=CARTESIAN_POINT('Ctrl Pts',(81.068251094894,190.995574215667,30.2782482805904)) ;
#75623=CARTESIAN_POINT('Ctrl Pts',(80.8501919227397,190.489539758744,30.2513203435596)) ;
#75624=CARTESIAN_POINT('Ctrl Pts',(80.9499521528871,190.489539758744,30.2513203435596)) ;
#75625=CARTESIAN_POINT('Ctrl Pts',(81.1133587857564,190.579819252469,30.2513203435596)) ;
#75626=CARTESIAN_POINT('Ctrl Pts',(81.1713865457921,190.819711599235,30.2513203435597)) ;
#75627=CARTESIAN_POINT('Ctrl Pts',(81.1139267500959,190.947232808556,30.2513203435596)) ;
#75628=CARTESIAN_POINT('Ctrl Pts',(81.068251094894,190.995574215667,30.2513203435596)) ;
#75629=CARTESIAN_POINT('',(80.8501919227397,190.489539758744,30.2513203435596)) ;
#75630=CARTESIAN_POINT('Ctrl Pts',(81.068251094894,190.995574215667,30.2513203435596)) ;
#75631=CARTESIAN_POINT('Ctrl Pts',(81.1139267500959,190.947232808556,30.2513203435596)) ;
#75632=CARTESIAN_POINT('Ctrl Pts',(81.1713865457921,190.819711599235,30.2513203435597)) ;
#75633=CARTESIAN_POINT('Ctrl Pts',(81.1133587857564,190.579819252469,30.2513203435596)) ;
#75634=CARTESIAN_POINT('Ctrl Pts',(80.9499521528871,190.489539758744,30.2513203435596)) ;
#75635=CARTESIAN_POINT('Ctrl Pts',(80.8501919227397,190.489539758744,30.2513203435596)) ;
#75636=CARTESIAN_POINT('',(80.8501919227397,190.369539758744,30.3713203435596)) ;
#75637=CARTESIAN_POINT('Origin',(80.8501919227397,190.369539758744,30.2513203435596)) ;
#75638=CARTESIAN_POINT('Ctrl Pts',(80.8501919227397,190.369539758744,30.3713203435596)) ;
#75639=CARTESIAN_POINT('Ctrl Pts',(80.989856244946,190.369539758744,30.3713203435596)) ;
#75640=CARTESIAN_POINT('Ctrl Pts',(81.2186255309631,190.49593104996,30.3713203435596)) ;
#75641=CARTESIAN_POINT('Ctrl Pts',(81.299864395013,190.831780335431,30.3713203435596)) ;
#75642=CARTESIAN_POINT('Ctrl Pts',(81.2194206810384,191.01031002848,30.3713203435596)) ;
#75643=CARTESIAN_POINT('Ctrl Pts',(81.1554747637557,191.077987998436,30.3713203435596)) ;
#75644=CARTESIAN_POINT('Origin',(75.6106165726094,190.369539758744,30.2513203435596)) ;
#75645=CARTESIAN_POINT('',(78.1546571314538,190.489539758744,30.2513203435596)) ;
#75646=CARTESIAN_POINT('',(78.1546571314538,190.369539758744,30.3713203435596)) ;
#75647=CARTESIAN_POINT('Origin',(78.1546571314538,190.369539758744,30.2513203435596)) ;
#75648=CARTESIAN_POINT('',(75.6106165726094,190.369539758744,30.3713203435596)) ;
#75649=CARTESIAN_POINT('',(75.6106165726094,190.489539758744,30.2513203435596)) ;
#75650=CARTESIAN_POINT('Ctrl Pts',(77.491702623914,190.586826448256,30.3713203435596)) ;
#75651=CARTESIAN_POINT('Ctrl Pts',(77.6823045866468,190.44684797572,30.3713203435596)) ;
#75652=CARTESIAN_POINT('Ctrl Pts',(77.9181765170879,190.369539758744,30.3713203435596)) ;
#75653=CARTESIAN_POINT('Ctrl Pts',(78.1546571314538,190.369539758744,30.3713203435596)) ;
#75654=CARTESIAN_POINT('Ctrl Pts',(77.5129550015727,190.615764790139,30.3713203435596)) ;
#75655=CARTESIAN_POINT('Ctrl Pts',(77.6974203503338,190.480293059496,30.3713203435596)) ;
#75656=CARTESIAN_POINT('Ctrl Pts',(77.9257902384858,190.405443674785,30.3713203435596)) ;
#75657=CARTESIAN_POINT('Ctrl Pts',(78.1546571314538,190.405443674785,30.3713203435596)) ;
#75658=CARTESIAN_POINT('Ctrl Pts',(77.5497327415575,190.665843272201,30.3411619198148)) ;
#75659=CARTESIAN_POINT('Ctrl Pts',(77.723657194007,190.538112797439,30.3411619198148)) ;
#75660=CARTESIAN_POINT('Ctrl Pts',(77.9388683705258,190.467576246952,30.3411619198148)) ;
#75661=CARTESIAN_POINT('Ctrl Pts',(78.1546571314538,190.467576246952,30.3411619198148)) ;
#75662=CARTESIAN_POINT('Ctrl Pts',(77.5627334640076,190.683545731522,30.2782482805904)) ;
#75663=CARTESIAN_POINT('Ctrl Pts',(77.7328971903007,190.558577141766,30.2782482805904)) ;
#75664=CARTESIAN_POINT('Ctrl Pts',(77.9435343184476,190.489539758744,30.2782482805904)) ;
#75665=CARTESIAN_POINT('Ctrl Pts',(78.1546571314538,190.489539758744,30.2782482805904)) ;
#75666=CARTESIAN_POINT('Ctrl Pts',(77.5627334640076,190.683545731522,30.2513203435596)) ;
#75667=CARTESIAN_POINT('Ctrl Pts',(77.732913787876,190.558564952473,30.2513203435596)) ;
#75668=CARTESIAN_POINT('Ctrl Pts',(77.9435137257698,190.489539758744,30.2513203435596)) ;
#75669=CARTESIAN_POINT('Ctrl Pts',(78.1546571314538,190.489539758744,30.2513203435596)) ;
#75670=CARTESIAN_POINT('',(77.5627334640076,190.683545731522,30.2513203435596)) ;
#75671=CARTESIAN_POINT('Origin',(78.0776054738973,191.254450606239,30.2513203435596)) ;
#75672=CARTESIAN_POINT('',(77.491702623914,190.586826448256,30.3713203435596)) ;
#75673=CARTESIAN_POINT('Origin',(77.491702623914,190.586826448256,30.2513203435596)) ;
#75674=CARTESIAN_POINT('Origin',(78.0683592750124,191.226239907973,30.3713203435596)) ;
#75675=CARTESIAN_POINT('Ctrl Pts',(77.5627334640075,190.683545731522,30.2513203435596)) ;
#75676=CARTESIAN_POINT('Ctrl Pts',(73.9385194970161,193.345175905566,30.2513203435596)) ;
#75677=CARTESIAN_POINT('Ctrl Pts',(70.594189416785,196.433476943649,30.2513203435596)) ;
#75678=CARTESIAN_POINT('Ctrl Pts',(67.9762844730848,200.080907092773,30.2513203435596)) ;
#75679=CARTESIAN_POINT('Ctrl Pts',(77.5627334640075,190.683545731522,30.2872242596007)) ;
#75680=CARTESIAN_POINT('Ctrl Pts',(73.9385438761009,193.345158001516,30.2872242596007)) ;
#75681=CARTESIAN_POINT('Ctrl Pts',(70.594158916818,196.433519438125,30.2872242596007)) ;
#75682=CARTESIAN_POINT('Ctrl Pts',(67.9762844730848,200.080907092773,30.2872242596007)) ;
#75683=CARTESIAN_POINT('Ctrl Pts',(77.544881982401,190.659238226445,30.3493568382152)) ;
#75684=CARTESIAN_POINT('Ctrl Pts',(73.9187452261289,193.322280500881,30.3493568382152)) ;
#75685=CARTESIAN_POINT('Ctrl Pts',(70.5720941363296,196.412540172779,30.3493568382152)) ;
#75686=CARTESIAN_POINT('Ctrl Pts',(67.951783646648,200.063321880163,30.3493568382152)) ;
#75687=CARTESIAN_POINT('Ctrl Pts',(77.507641907158,190.608530204668,30.3713203435596)) ;
#75688=CARTESIAN_POINT('Ctrl Pts',(73.8775078677682,193.274508092028,30.3713203435596)) ;
#75689=CARTESIAN_POINT('Ctrl Pts',(70.5259837109279,196.368888014437,30.3713203435596)) ;
#75690=CARTESIAN_POINT('Ctrl Pts',(67.9006723361061,200.026637270156,30.3713203435596)) ;
#75691=CARTESIAN_POINT('Ctrl Pts',(77.491702623914,190.586826448256,30.3713203435596)) ;
#75692=CARTESIAN_POINT('Ctrl Pts',(73.8598602830395,193.254058915732,30.3713203435596)) ;
#75693=CARTESIAN_POINT('Ctrl Pts',(70.5062445476854,196.350208787435,30.3713203435596)) ;
#75694=CARTESIAN_POINT('Ctrl Pts',(67.8787959663517,200.010935733954,30.3713203435596)) ;
#75695=CARTESIAN_POINT('',(67.9762844730848,200.080907092773,30.2513203435596)) ;
#75696=CARTESIAN_POINT('',(67.8787959663517,200.010935733954,30.3713203435596)) ;
#75697=CARTESIAN_POINT('Origin',(67.8787959663517,200.010935733954,30.2513203435596)) ;
#75698=CARTESIAN_POINT('Ctrl Pts',(67.8787959663517,200.010935733954,30.3713203435596)) ;
#75699=CARTESIAN_POINT('Ctrl Pts',(70.5062445476854,196.350208787435,30.3713203435596)) ;
#75700=CARTESIAN_POINT('Ctrl Pts',(73.8598602830395,193.254058915732,30.3713203435596)) ;
#75701=CARTESIAN_POINT('Ctrl Pts',(77.491702623914,190.586826448256,30.3713203435596)) ;
#75702=CARTESIAN_POINT('Ctrl Pts',(77.5627334640075,190.683545731522,30.2513203435596)) ;
#75703=CARTESIAN_POINT('Ctrl Pts',(73.9385194970161,193.345175905566,30.2513203435596)) ;
#75704=CARTESIAN_POINT('Ctrl Pts',(70.594189416785,196.433476943649,30.2513203435596)) ;
#75705=CARTESIAN_POINT('Ctrl Pts',(67.9762844730848,200.080907092773,30.2513203435596)) ;
#75706=CARTESIAN_POINT('Ctrl Pts',(68.2200057399177,200.67583548982,30.3713203435596)) ;
#75707=CARTESIAN_POINT('Ctrl Pts',(68.0884112603097,200.67583548982,30.3713203435596)) ;
#75708=CARTESIAN_POINT('Ctrl Pts',(67.8720857272373,200.564584339121,30.3713203435596)) ;
#75709=CARTESIAN_POINT('Ctrl Pts',(67.7720303794687,200.257091150086,30.3713203435596)) ;
#75710=CARTESIAN_POINT('Ctrl Pts',(67.8276412744005,200.082207674573,30.3713203435596)) ;
#75711=CARTESIAN_POINT('Ctrl Pts',(67.8787959663517,200.010935733954,30.3713203435596)) ;
#75712=CARTESIAN_POINT('Ctrl Pts',(68.2200057399177,200.639931573779,30.3713203435596)) ;
#75713=CARTESIAN_POINT('Ctrl Pts',(68.0997094233937,200.639931573779,30.3713203435596)) ;
#75714=CARTESIAN_POINT('Ctrl Pts',(67.9018687303379,200.538060654086,30.3713203435596)) ;
#75715=CARTESIAN_POINT('Ctrl Pts',(67.8104033772253,200.256966885486,30.3713203435596)) ;
#75716=CARTESIAN_POINT('Ctrl Pts',(67.8612016997572,200.097023939243,30.3713203435596)) ;
#75717=CARTESIAN_POINT('Ctrl Pts',(67.9079644593576,200.031871115557,30.3713203435596)) ;
#75718=CARTESIAN_POINT('Ctrl Pts',(68.2200057399177,200.577799006671,30.3411619155991)) ;
#75719=CARTESIAN_POINT('Ctrl Pts',(68.1191163416272,200.577799006671,30.3411619155991)) ;
#75720=CARTESIAN_POINT('Ctrl Pts',(67.9532874484581,200.492547433761,30.341161915599)) ;
#75721=CARTESIAN_POINT('Ctrl Pts',(67.8765782061601,200.256802125843,30.3411619155991)) ;
#75722=CARTESIAN_POINT('Ctrl Pts',(67.9192225065329,200.122742265589,30.3411619155991)) ;
#75723=CARTESIAN_POINT('Ctrl Pts',(67.9584412192484,200.068100283452,30.3411619155991)) ;
#75724=CARTESIAN_POINT('Ctrl Pts',(68.2200057399177,200.55583548982,30.2782482805904)) ;
#75725=CARTESIAN_POINT('Ctrl Pts',(68.1260402409674,200.55583548982,30.2782482805904)) ;
#75726=CARTESIAN_POINT('Ctrl Pts',(67.9715170756471,200.476288797847,30.2782482805904)) ;
#75727=CARTESIAN_POINT('Ctrl Pts',(67.900071986214,200.256721779767,30.2782482805904)) ;
#75728=CARTESIAN_POINT('Ctrl Pts',(67.9397572861757,200.131799071535,30.2782482805904)) ;
#75729=CARTESIAN_POINT('Ctrl Pts',(67.9762844730848,200.080907092773,30.2782482805904)) ;
#75730=CARTESIAN_POINT('Ctrl Pts',(68.2200057399177,200.55583548982,30.2513203435596)) ;
#75731=CARTESIAN_POINT('Ctrl Pts',(68.1260096830549,200.55583548982,30.2513203435596)) ;
#75732=CARTESIAN_POINT('Ctrl Pts',(67.9714914451459,200.476370382178,30.2513203435596)) ;
#75733=CARTESIAN_POINT('Ctrl Pts',(67.900023339597,200.25673239001,30.2513203435596)) ;
#75734=CARTESIAN_POINT('Ctrl Pts',(67.9397454074054,200.131815621786,30.2513203435596)) ;
#75735=CARTESIAN_POINT('Ctrl Pts',(67.9762844730848,200.080907092773,30.2513203435596)) ;
#75736=CARTESIAN_POINT('',(68.2200057399177,200.55583548982,30.2513203435596)) ;
#75737=CARTESIAN_POINT('Ctrl Pts',(67.9762844730848,200.080907092773,30.2513203435596)) ;
#75738=CARTESIAN_POINT('Ctrl Pts',(67.9397454074054,200.131815621786,30.2513203435596)) ;
#75739=CARTESIAN_POINT('Ctrl Pts',(67.900023339597,200.25673239001,30.2513203435596)) ;
#75740=CARTESIAN_POINT('Ctrl Pts',(67.9714914451459,200.476370382178,30.2513203435596)) ;
#75741=CARTESIAN_POINT('Ctrl Pts',(68.1260096830549,200.55583548982,30.2513203435596)) ;
#75742=CARTESIAN_POINT('Ctrl Pts',(68.2200057399177,200.55583548982,30.2513203435596)) ;
#75743=CARTESIAN_POINT('',(68.2200057399177,200.67583548982,30.3713203435596)) ;
#75744=CARTESIAN_POINT('Origin',(68.2200057399177,200.67583548982,30.2513203435596)) ;
#75745=CARTESIAN_POINT('Ctrl Pts',(68.2200057399177,200.67583548982,30.3713203435596)) ;
#75746=CARTESIAN_POINT('Ctrl Pts',(68.0884112603097,200.67583548982,30.3713203435596)) ;
#75747=CARTESIAN_POINT('Ctrl Pts',(67.8720857272373,200.564584339121,30.3713203435596)) ;
#75748=CARTESIAN_POINT('Ctrl Pts',(67.7720303794687,200.257091150086,30.3713203435596)) ;
#75749=CARTESIAN_POINT('Ctrl Pts',(67.8276412744005,200.082207674573,30.3713203435596)) ;
#75750=CARTESIAN_POINT('Ctrl Pts',(67.8787959663517,200.010935733954,30.3713203435596)) ;
#75751=CARTESIAN_POINT('Origin',(68.6561288592431,200.67583548982,30.2513203435596)) ;
#75752=CARTESIAN_POINT('',(73.4866103162092,200.55583548982,30.2513203435596)) ;
#75753=CARTESIAN_POINT('',(73.4866103162092,200.67583548982,30.3713203435596)) ;
#75754=CARTESIAN_POINT('Origin',(73.4866103162092,200.67583548982,30.2513203435596)) ;
#75755=CARTESIAN_POINT('',(68.6561288592431,200.67583548982,30.3713203435596)) ;
#75756=CARTESIAN_POINT('',(68.6561288592431,200.55583548982,30.2513203435596)) ;
#75757=CARTESIAN_POINT('Ctrl Pts',(73.8469698134568,200.47159949769,30.371320342471)) ;
#75758=CARTESIAN_POINT('Ctrl Pts',(73.7726721832933,200.595732430761,30.371320342471)) ;
#75759=CARTESIAN_POINT('Ctrl Pts',(73.6304497677198,200.676158620816,30.371320342471)) ;
#75760=CARTESIAN_POINT('Ctrl Pts',(73.4857810847946,200.675850235661,30.371320342471)) ;
#75761=CARTESIAN_POINT('Ctrl Pts',(73.8161607140537,200.453153015436,30.3713253446552)) ;
#75762=CARTESIAN_POINT('Ctrl Pts',(73.7482432100789,200.566626907111,30.3713253446551)) ;
#75763=CARTESIAN_POINT('Ctrl Pts',(73.6180983919013,200.640223265598,30.3713253446551)) ;
#75764=CARTESIAN_POINT('Ctrl Pts',(73.4858522887322,200.639941069093,30.3713253446551)) ;
#75765=CARTESIAN_POINT('Ctrl Pts',(73.7628460214403,200.421230580689,30.3411670622856)) ;
#75766=CARTESIAN_POINT('Ctrl Pts',(73.7058860185115,200.516396497646,30.3411670622856)) ;
#75767=CARTESIAN_POINT('Ctrl Pts',(73.5968841830501,200.578036586515,30.3411670622856)) ;
#75768=CARTESIAN_POINT('Ctrl Pts',(73.4859745900404,200.577800234443,30.3411670622856)) ;
#75769=CARTESIAN_POINT('Ctrl Pts',(73.7440002787433,200.40994706903,30.2782482805904)) ;
#75770=CARTESIAN_POINT('Ctrl Pts',(73.6909501011225,200.498581129447,30.2782482805904)) ;
#75771=CARTESIAN_POINT('Ctrl Pts',(73.5893152199704,200.556055236005,30.2782482805904)) ;
#75772=CARTESIAN_POINT('Ctrl Pts',(73.4860182236672,200.555834858296,30.2782482805904)) ;
#75773=CARTESIAN_POINT('Ctrl Pts',(73.7440003787313,200.409946903396,30.2513203435596)) ;
#75774=CARTESIAN_POINT('Ctrl Pts',(73.6909326264421,200.49860997033,30.2513203435596)) ;
#75775=CARTESIAN_POINT('Ctrl Pts',(73.5893489416074,200.556055125582,30.2513203435596)) ;
#75776=CARTESIAN_POINT('Ctrl Pts',(73.4860180301928,200.555834858614,30.2513203435596)) ;
#75777=CARTESIAN_POINT('Origin',(73.5222221716454,200.318810051956,30.2513203435596)) ;
#75778=CARTESIAN_POINT('Origin',(73.5364669138164,200.343999876809,30.3713203435596)) ;
#75779=CARTESIAN_POINT('Ctrl Pts',(78.1546571314538,190.489539758744,23.4913203435596)) ;
#75780=CARTESIAN_POINT('Ctrl Pts',(78.1546571314538,190.489539758744,31.6033203435596)) ;
#75781=CARTESIAN_POINT('Ctrl Pts',(77.9435093125031,190.489539758744,23.4913203435596)) ;
#75782=CARTESIAN_POINT('Ctrl Pts',(77.9435093125031,190.489539758744,31.6033203435596)) ;
#75783=CARTESIAN_POINT('Ctrl Pts',(77.7329173449427,190.558562340156,23.4913203435596)) ;
#75784=CARTESIAN_POINT('Ctrl Pts',(77.7329173449427,190.558562340156,31.6033203435596)) ;
#75785=CARTESIAN_POINT('Ctrl Pts',(77.5627334640076,190.683545731522,23.4913203435596)) ;
#75786=CARTESIAN_POINT('Ctrl Pts',(77.5627334640076,190.683545731522,31.6033203435596)) ;
#75787=CARTESIAN_POINT('',(78.1546571314538,190.489539758744,23.4913203435596)) ;
#75788=CARTESIAN_POINT('',(78.1546571314538,190.489539758744,30.2513203435596)) ;
#75789=CARTESIAN_POINT('',(77.5627334640076,190.683545731522,23.4913203435596)) ;
#75790=CARTESIAN_POINT('Origin',(78.077605473898,191.254450606248,23.4913203435596)) ;
#75791=CARTESIAN_POINT('',(77.5627334640076,190.683545731522,23.4913203435596)) ;
#75792=CARTESIAN_POINT('Origin',(81.5507230003364,190.489539758744,23.8713203435596)) ;
#75793=CARTESIAN_POINT('',(80.8501919227397,190.489539758744,23.4913203435596)) ;
#75794=CARTESIAN_POINT('',(80.8501919227397,190.489539758744,23.4913203435596)) ;
#75795=CARTESIAN_POINT('',(78.07353074889,190.489539758744,23.4913203435596)) ;
#75796=CARTESIAN_POINT('Ctrl Pts',(81.068251094894,190.995574215667,23.4913203435596)) ;
#75797=CARTESIAN_POINT('Ctrl Pts',(81.068251094894,190.995574215667,31.6033203435596)) ;
#75798=CARTESIAN_POINT('Ctrl Pts',(81.1139288980579,190.947230535233,23.4913203435596)) ;
#75799=CARTESIAN_POINT('Ctrl Pts',(81.1139288980579,190.947230535233,31.6033203435596)) ;
#75800=CARTESIAN_POINT('Ctrl Pts',(81.1716384658622,190.819103522118,23.4913203435596)) ;
#75801=CARTESIAN_POINT('Ctrl Pts',(81.1716384658622,190.819103522118,31.6033203435596)) ;
#75802=CARTESIAN_POINT('Ctrl Pts',(81.1216272012763,190.614215654147,23.4913203435596)) ;
#75803=CARTESIAN_POINT('Ctrl Pts',(81.1216272012763,190.614215654147,31.6033203435596)) ;
#75804=CARTESIAN_POINT('Ctrl Pts',(80.983303578287,190.505926367357,23.4913203435596)) ;
#75805=CARTESIAN_POINT('Ctrl Pts',(80.983303578287,190.505926367357,31.6033203435596)) ;
#75806=CARTESIAN_POINT('Ctrl Pts',(80.8834468965772,190.489539758744,23.4913203435596)) ;
#75807=CARTESIAN_POINT('Ctrl Pts',(80.8834468965772,190.489539758744,31.6033203435596)) ;
#75808=CARTESIAN_POINT('Ctrl Pts',(80.8501919227397,190.489539758744,23.4913203435596)) ;
#75809=CARTESIAN_POINT('Ctrl Pts',(80.8501919227397,190.489539758744,31.6033203435596)) ;
#75810=CARTESIAN_POINT('',(81.068251094894,190.995574215667,23.4913203435596)) ;
#75811=CARTESIAN_POINT('',(81.068251094894,190.995574215667,30.2513203435596)) ;
#75812=CARTESIAN_POINT('Ctrl Pts',(80.8501919227397,190.489539758744,23.4913203435596)) ;
#75813=CARTESIAN_POINT('Ctrl Pts',(80.8834468965772,190.489539758744,23.4913203435596)) ;
#75814=CARTESIAN_POINT('Ctrl Pts',(80.983303578287,190.505926367357,23.4913203435596)) ;
#75815=CARTESIAN_POINT('Ctrl Pts',(81.1216272012763,190.614215654147,23.4913203435596)) ;
#75816=CARTESIAN_POINT('Ctrl Pts',(81.1716384658622,190.819103522118,23.4913203435596)) ;
#75817=CARTESIAN_POINT('Ctrl Pts',(81.1139288980579,190.947230535233,23.4913203435596)) ;
#75818=CARTESIAN_POINT('Ctrl Pts',(81.068251094894,190.995574215667,23.4913203435596)) ;
#75819=CARTESIAN_POINT('Ctrl Pts',(73.6566785252795,200.55583548982,17.854339447693)) ;
#75820=CARTESIAN_POINT('Ctrl Pts',(73.6566785252795,200.55583548982,32.8747165227329)) ;
#75821=CARTESIAN_POINT('Ctrl Pts',(75.7001422864503,197.125245060908,17.854339447693)) ;
#75822=CARTESIAN_POINT('Ctrl Pts',(75.7001422864503,197.125245060908,32.8747165227329)) ;
#75823=CARTESIAN_POINT('Ctrl Pts',(78.3842768400396,193.78102322923,17.854339447693)) ;
#75824=CARTESIAN_POINT('Ctrl Pts',(78.3842768400396,193.78102322923,32.8747165227329)) ;
#75825=CARTESIAN_POINT('Ctrl Pts',(81.5507230003364,190.489539758744,17.854339447693)) ;
#75826=CARTESIAN_POINT('Ctrl Pts',(81.5507230003364,190.489539758744,32.8747165227329)) ;
#75827=CARTESIAN_POINT('',(73.7436956568153,200.410454788892,23.4913203435596)) ;
#75828=CARTESIAN_POINT('',(73.7436956568153,200.410454788892,23.4913203435596)) ;
#75829=CARTESIAN_POINT('Ctrl Pts',(81.0682510948939,190.995574215667,23.4913203435596)) ;
#75830=CARTESIAN_POINT('Ctrl Pts',(78.3304755598256,193.893133563934,23.4913203435596)) ;
#75831=CARTESIAN_POINT('Ctrl Pts',(75.7953376765802,196.999191831293,23.4913203435596)) ;
#75832=CARTESIAN_POINT('Ctrl Pts',(73.7436956568154,200.410454788892,23.4913203435596)) ;
#75833=CARTESIAN_POINT('Origin',(69.6705101448823,217.61928420644,30.3713203435596)) ;
#75834=CARTESIAN_POINT('',(60.7116108526749,219.655485092203,30.3713203435596)) ;
#75835=CARTESIAN_POINT('',(60.7116108526749,220.636977801421,30.3713203435596)) ;
#75836=CARTESIAN_POINT('',(60.7116108526749,219.132346607579,30.3713203435596)) ;
#75837=CARTESIAN_POINT('',(60.7297059832955,219.541923491104,30.3713203435596)) ;
#75838=CARTESIAN_POINT('Origin',(64.1568347953872,220.146231446812,30.3713203435596)) ;
#75839=CARTESIAN_POINT('',(60.7116108526749,219.512965228765,30.3713203435596)) ;
#75840=CARTESIAN_POINT('',(61.5409585020332,220.840198908612,30.3713203435596)) ;
#75841=CARTESIAN_POINT('',(60.7116108526749,216.156773929576,30.3713203435596)) ;
#75842=CARTESIAN_POINT('',(60.7116108526749,218.583329440748,30.3713203435596)) ;
#75843=CARTESIAN_POINT('',(60.882803220617,214.421530538057,30.3713203435596)) ;
#75844=CARTESIAN_POINT('Origin',(69.59874093474,216.157477355757,30.3713203435596)) ;
#75845=CARTESIAN_POINT('',(60.9230784080337,214.221542284825,30.3713203435596)) ;
#75846=CARTESIAN_POINT('Origin',(144.68997749936,269.113837772005,30.3713203435596)) ;
#75847=CARTESIAN_POINT('',(61.2615982170421,212.685341204894,30.3713203435596)) ;
#75848=CARTESIAN_POINT('Origin',(181.381319461017,301.79529262085,30.3713203435596)) ;
#75849=CARTESIAN_POINT('',(65.371678614805,202.116206289766,30.3713203435596)) ;
#75850=CARTESIAN_POINT('Origin',(136.119542118133,279.889814321862,30.3713203435596)) ;
#75851=CARTESIAN_POINT('',(66.2956301826426,200.621620147878,30.3713203435596)) ;
#75852=CARTESIAN_POINT('Origin',(94.003679466687,218.783592840218,30.3713203435596)) ;
#75853=CARTESIAN_POINT('',(77.1942359127804,189.615407485539,30.3713203435596)) ;
#75854=CARTESIAN_POINT('Ctrl Pts',(77.1942359127805,189.615407485539,30.3713203435596)) ;
#75855=CARTESIAN_POINT('Ctrl Pts',(74.7931595483741,191.357615194406,30.3713203435596)) ;
#75856=CARTESIAN_POINT('Ctrl Pts',(70.8082383262559,194.719115063076,30.3713203435596)) ;
#75857=CARTESIAN_POINT('Ctrl Pts',(67.5153419459542,198.760824785205,30.3713203435596)) ;
#75858=CARTESIAN_POINT('Ctrl Pts',(66.2956301826426,200.621620147878,30.3713203435596)) ;
#75859=CARTESIAN_POINT('',(77.8285014478222,189.409539758744,30.3713203435596)) ;
#75860=CARTESIAN_POINT('Origin',(77.7459982214618,190.235352500614,30.3713203435596)) ;
#75861=CARTESIAN_POINT('',(83.2194473860052,189.409539758744,30.3713203435596)) ;
#75862=CARTESIAN_POINT('',(73.5558661461117,189.409539758744,30.3713203435596)) ;
#75863=CARTESIAN_POINT('',(83.4878143389934,190.058573545737,30.3713203435596)) ;
#75864=CARTESIAN_POINT('Ctrl Pts',(83.4878143389935,190.058573545737,30.3713203435596)) ;
#75865=CARTESIAN_POINT('Ctrl Pts',(83.5482147548369,189.998322839904,30.3713203435596)) ;
#75866=CARTESIAN_POINT('Ctrl Pts',(83.6266011938506,189.835494820776,30.3713203435596)) ;
#75867=CARTESIAN_POINT('Ctrl Pts',(83.576428513561,189.615885650627,30.3713203435596)) ;
#75868=CARTESIAN_POINT('Ctrl Pts',(83.4319195690048,189.454561122737,30.3713203435596)) ;
#75869=CARTESIAN_POINT('Ctrl Pts',(83.3047606779792,189.409539758744,30.3713203435596)) ;
#75870=CARTESIAN_POINT('Ctrl Pts',(83.2194473860052,189.409539758744,30.3713203435596)) ;
#75871=CARTESIAN_POINT('',(74.0713631125318,201.997275065426,30.3713203435596)) ;
#75872=CARTESIAN_POINT('Ctrl Pts',(74.071363112532,201.997275065426,30.3713203435596)) ;
#75873=CARTESIAN_POINT('Ctrl Pts',(75.4893853751038,199.461004730524,30.3713203435596)) ;
#75874=CARTESIAN_POINT('Ctrl Pts',(78.4869236645555,195.326452202177,30.3713203435596)) ;
#75875=CARTESIAN_POINT('Ctrl Pts',(81.9448902074828,191.59767334615,30.3713203435596)) ;
#75876=CARTESIAN_POINT('Ctrl Pts',(83.4878143389934,190.058573545737,30.3713203435596)) ;
#75877=CARTESIAN_POINT('',(70.3587497899394,213.244508470505,30.3713203435596)) ;
#75878=CARTESIAN_POINT('Ctrl Pts',(70.3587497899395,213.244508470505,30.3713203435596)) ;
#75879=CARTESIAN_POINT('Ctrl Pts',(70.6230150970638,210.988834878587,30.3713203435596)) ;
#75880=CARTESIAN_POINT('Ctrl Pts',(71.5450141265831,207.094613224745,30.3713203435596)) ;
#75881=CARTESIAN_POINT('Ctrl Pts',(73.2401341423739,203.484008690256,30.3713203435596)) ;
#75882=CARTESIAN_POINT('Ctrl Pts',(74.0713631125318,201.997275065426,30.3713203435596)) ;
#75883=CARTESIAN_POINT('',(70.1614015403524,216.000591762293,30.3713203435596)) ;
#75884=CARTESIAN_POINT('Origin',(97.4802149293723,222.398003042729,30.3713203435596)) ;
#75885=CARTESIAN_POINT('',(70.1824009080094,218.33629382542,30.3713203435596)) ;
#75886=CARTESIAN_POINT('Origin',(99.3986297237061,223.018122277912,30.3713203435596)) ;
#75887=CARTESIAN_POINT('',(70.2600011794933,219.566058197824,30.3713203435596)) ;
#75888=CARTESIAN_POINT('Origin',(103.749334371737,216.83549248614,30.3713203435596)) ;
#75889=CARTESIAN_POINT('',(64.9314996085946,223.538913929329,30.3713203435596)) ;
#75890=CARTESIAN_POINT('',(70.5636770849813,219.33964171939,30.3713203435596)) ;
#75891=CARTESIAN_POINT('Origin',(64.1568347953872,220.146231446812,30.3713203435596)) ;
#75892=CARTESIAN_POINT('',(66.8340607823661,201.93583548982,30.3713203435596)) ;
#75893=CARTESIAN_POINT('',(72.3111547045756,201.93583548982,30.3713203435596)) ;
#75894=CARTESIAN_POINT('',(71.2393508060962,201.93583548982,30.3713203435596)) ;
#75895=CARTESIAN_POINT('',(66.4746484362165,202.138527493107,30.3713203435596)) ;
#75896=CARTESIAN_POINT('Origin',(66.7842973113484,202.267595176532,30.3713203435596)) ;
#75897=CARTESIAN_POINT('',(62.39752314559,212.090513424339,30.3713203435596)) ;
#75898=CARTESIAN_POINT('Origin',(123.304723958797,266.258739720462,30.3713203435596)) ;
#75899=CARTESIAN_POINT('',(62.8448887910812,212.613106134355,30.3713203435596)) ;
#75900=CARTESIAN_POINT('Ctrl Pts',(62.8448887910812,212.613106134355,30.3713203435596)) ;
#75901=CARTESIAN_POINT('Ctrl Pts',(62.7302820487196,212.624233777445,30.3713203435596)) ;
#75902=CARTESIAN_POINT('Ctrl Pts',(62.5327477139549,212.559161211515,30.3713203435596)) ;
#75903=CARTESIAN_POINT('Ctrl Pts',(62.3821824103364,212.323740151324,30.3713203435596)) ;
#75904=CARTESIAN_POINT('Ctrl Pts',(62.3784128818005,212.164860433323,30.3713203435596)) ;
#75905=CARTESIAN_POINT('Ctrl Pts',(62.39752314559,212.090513424339,30.3713203435596)) ;
#75906=CARTESIAN_POINT('',(69.2431719411391,211.991870334298,30.3713203435596)) ;
#75907=CARTESIAN_POINT('',(65.7730634668025,212.328797532388,30.3713203435596)) ;
#75908=CARTESIAN_POINT('',(69.6168298215689,211.643116744604,30.3713203435596)) ;
#75909=CARTESIAN_POINT('Ctrl Pts',(69.6168298215689,211.643116744604,30.3713203435596)) ;
#75910=CARTESIAN_POINT('Ctrl Pts',(69.6038817585733,211.72053657915,30.3713203435596)) ;
#75911=CARTESIAN_POINT('Ctrl Pts',(69.5217274044295,211.89264098624,30.3713203435596)) ;
#75912=CARTESIAN_POINT('Ctrl Pts',(69.3473422258095,211.981756010092,30.3713203435596)) ;
#75913=CARTESIAN_POINT('Ctrl Pts',(69.2431719411391,211.991870334298,30.3713203435596)) ;
#75914=CARTESIAN_POINT('',(72.6841279270487,202.548944203549,30.3713203435596)) ;
#75915=CARTESIAN_POINT('Origin',(95.7743907326708,211.507553737734,30.3713203435596)) ;
#75916=CARTESIAN_POINT('Ctrl Pts',(72.3111547045756,201.93583548982,30.3713203435596)) ;
#75917=CARTESIAN_POINT('Ctrl Pts',(72.434062830227,201.93583548982,30.3713203435596)) ;
#75918=CARTESIAN_POINT('Ctrl Pts',(72.6367193429415,202.032109677482,30.3713203435596)) ;
#75919=CARTESIAN_POINT('Ctrl Pts',(72.7529836107094,202.308661221514,30.3713203435596)) ;
#75920=CARTESIAN_POINT('Ctrl Pts',(72.7218019430032,202.476180013561,30.3713203435596)) ;
#75921=CARTESIAN_POINT('Ctrl Pts',(72.6841279270486,202.548944203549,30.3713203435596)) ;
#75922=CARTESIAN_POINT('',(69.2883239479992,219.455458322081,30.3713203435596)) ;
#75923=CARTESIAN_POINT('',(69.3183833051634,219.827104833273,30.3713203435596)) ;
#75924=CARTESIAN_POINT('Ctrl Pts',(69.2883239479992,219.455458322081,30.3713203435596)) ;
#75925=CARTESIAN_POINT('Ctrl Pts',(69.2948338469246,219.541101232703,30.3713203435596)) ;
#75926=CARTESIAN_POINT('Ctrl Pts',(69.3016608747709,219.626720035554,30.3713203435596)) ;
#75927=CARTESIAN_POINT('Ctrl Pts',(69.3119969022076,219.750576599373,30.3713203435596)) ;
#75928=CARTESIAN_POINT('Ctrl Pts',(69.3151901036855,219.788840716323,30.3713203435596)) ;
#75929=CARTESIAN_POINT('Ctrl Pts',(69.3183833051634,219.827104833273,30.3713203435596)) ;
#75930=CARTESIAN_POINT('',(69.2071742804062,215.793615651063,30.3713203435596)) ;
#75931=CARTESIAN_POINT('Origin',(98.9242731431935,222.80312748053,30.3713203435596)) ;
#75932=CARTESIAN_POINT('',(69.360748483532,213.535508647726,30.3713203435596)) ;
#75933=CARTESIAN_POINT('Origin',(97.2384671995787,222.414143143253,30.3713203435596)) ;
#75934=CARTESIAN_POINT('',(69.0988421032155,213.27180916519,30.3713203435596)) ;
#75935=CARTESIAN_POINT('Ctrl Pts',(69.0988421032155,213.27180916519,30.3713203435596)) ;
#75936=CARTESIAN_POINT('Ctrl Pts',(69.1391356985346,213.267896893205,30.3713203435596)) ;
#75937=CARTESIAN_POINT('Ctrl Pts',(69.2113031834343,213.279382916547,30.3713203435596)) ;
#75938=CARTESIAN_POINT('Ctrl Pts',(69.3050219266113,213.343266910648,30.3713203435596)) ;
#75939=CARTESIAN_POINT('Ctrl Pts',(69.3577597203562,213.433390646791,30.3713203435596)) ;
#75940=CARTESIAN_POINT('Ctrl Pts',(69.3638888089739,213.505309174469,30.3713203435596)) ;
#75941=CARTESIAN_POINT('Ctrl Pts',(69.360748483532,213.535508647726,30.3713203435596)) ;
#75942=CARTESIAN_POINT('',(62.1323260763097,213.948217047756,30.3713203435596)) ;
#75943=CARTESIAN_POINT('',(69.2461649893318,213.257504976258,30.3713203435596)) ;
#75944=CARTESIAN_POINT('',(61.9206232262128,214.13786269141,30.3713203435596)) ;
#75945=CARTESIAN_POINT('Ctrl Pts',(61.9206232262128,214.13786269141,30.3713203435596)) ;
#75946=CARTESIAN_POINT('Ctrl Pts',(61.932507773129,214.081157854061,30.3713203435596)) ;
#75947=CARTESIAN_POINT('Ctrl Pts',(61.9908074934658,213.990274993108,30.3713203435596)) ;
#75948=CARTESIAN_POINT('Ctrl Pts',(62.0890768060814,213.952416298455,30.3713203435596)) ;
#75949=CARTESIAN_POINT('Ctrl Pts',(62.1323260763097,213.948217047756,30.3713203435596)) ;
#75950=CARTESIAN_POINT('',(61.8527608796043,214.467362912516,30.3713203435596)) ;
#75951=CARTESIAN_POINT('Origin',(157.009443961964,279.366832786929,30.3713203435596)) ;
#75952=CARTESIAN_POINT('',(61.6716108526749,216.276053366666,30.3713203435596)) ;
#75953=CARTESIAN_POINT('Origin',(70.7991555701787,216.276809010494,30.3713203435596)) ;
#75954=CARTESIAN_POINT('',(61.6716108526749,217.7102384348,30.3713203435596)) ;
#75955=CARTESIAN_POINT('',(61.6716108526749,216.520093569003,30.3713203435596)) ;
#75956=CARTESIAN_POINT('',(67.635124836556,220.037151707603,30.3713203435596)) ;
#75957=CARTESIAN_POINT('Origin',(64.1568347953872,220.146231446812,30.3713203435596)) ;
#75958=CARTESIAN_POINT('',(68.8498979833486,219.885565182264,30.3713203435596)) ;
#75959=CARTESIAN_POINT('',(66.2768347953872,220.146231446812,30.3713203435596)) ;
#75960=CARTESIAN_POINT('Origin',(64.1568347953872,220.146231446812,30.3713203435596)) ;
#75961=CARTESIAN_POINT('Origin',(71.2393508060962,201.93583548982,30.2513203435596)) ;
#75962=CARTESIAN_POINT('',(72.3111547045756,202.05583548982,30.2513203435596)) ;
#75963=CARTESIAN_POINT('Origin',(72.3111547045756,201.93583548982,30.2513203435596)) ;
#75964=CARTESIAN_POINT('',(66.8340607823661,202.05583548982,30.2513203435596)) ;
#75965=CARTESIAN_POINT('',(71.2393508060962,202.05583548982,30.2513203435596)) ;
#75966=CARTESIAN_POINT('Origin',(66.8340607823661,201.93583548982,30.2513203435596)) ;
#75967=CARTESIAN_POINT('Ctrl Pts',(66.4742123255349,202.139220627159,30.3713203424983)) ;
#75968=CARTESIAN_POINT('Ctrl Pts',(66.5486309050821,202.015550475992,30.3713203424983)) ;
#75969=CARTESIAN_POINT('Ctrl Pts',(66.6905454482115,201.935517212387,30.3713203424982)) ;
#75970=CARTESIAN_POINT('Ctrl Pts',(66.8348795711143,201.935820918413,30.3713203424982)) ;
#75971=CARTESIAN_POINT('Ctrl Pts',(66.5049776890707,202.157739831051,30.3713252816721)) ;
#75972=CARTESIAN_POINT('Ctrl Pts',(66.5730057722082,202.044688964891,30.3713252816721)) ;
#75973=CARTESIAN_POINT('Ctrl Pts',(66.7028689699091,201.97145210484,30.371325281672)) ;
#75974=CARTESIAN_POINT('Ctrl Pts',(66.8348092639751,201.97173001981,30.371325281672)) ;
#75975=CARTESIAN_POINT('Ctrl Pts',(66.5582167817037,202.189788148438,30.3411670675354)) ;
#75976=CARTESIAN_POINT('Ctrl Pts',(66.6152695314146,202.094976983773,30.3411670675354)) ;
#75977=CARTESIAN_POINT('Ctrl Pts',(66.7240353556309,202.033638070306,30.3411670675354)) ;
#75978=CARTESIAN_POINT('Ctrl Pts',(66.834688502964,202.033870836095,30.3411670675354)) ;
#75979=CARTESIAN_POINT('Ctrl Pts',(66.5770357137958,202.201116109631,30.2782482805904)) ;
#75980=CARTESIAN_POINT('Ctrl Pts',(66.6301722813347,202.112812443701,30.2782482805904)) ;
#75981=CARTESIAN_POINT('Ctrl Pts',(66.7315872550755,202.055619071211,30.2782482805904)) ;
#75982=CARTESIAN_POINT('Ctrl Pts',(66.8346454188596,202.055836105354,30.2782482805904)) ;
#75983=CARTESIAN_POINT('Ctrl Pts',(66.5770356146924,202.201116272943,30.2513203435596)) ;
#75984=CARTESIAN_POINT('Ctrl Pts',(66.6301897811885,202.112783710585,30.2513203435596)) ;
#75985=CARTESIAN_POINT('Ctrl Pts',(66.7315536124682,202.055619180086,30.2513203435596)) ;
#75986=CARTESIAN_POINT('Ctrl Pts',(66.8346456098891,202.055836105045,30.2513203435596)) ;
#75987=CARTESIAN_POINT('',(66.5773388238817,202.200616184912,30.2513203435596)) ;
#75988=CARTESIAN_POINT('Origin',(66.7985154459214,202.29280669461,30.2513203435596)) ;
#75989=CARTESIAN_POINT('Origin',(66.4746484362165,202.138527493107,30.2513203435596)) ;
#75990=CARTESIAN_POINT('Ctrl Pts',(66.5773376779735,202.200615492168,30.2513203435596)) ;
#75991=CARTESIAN_POINT('Ctrl Pts',(64.7228248908566,205.267850945375,30.2513203435596)) ;
#75992=CARTESIAN_POINT('Ctrl Pts',(63.4070162709899,208.645184776903,30.2513203435596)) ;
#75993=CARTESIAN_POINT('Ctrl Pts',(62.513745139331,212.120387295379,30.2513203435596)) ;
#75994=CARTESIAN_POINT('Ctrl Pts',(66.5773376779735,202.200615492168,30.2872242596007)) ;
#75995=CARTESIAN_POINT('Ctrl Pts',(64.7228470996252,205.267814213613,30.2872242596007)) ;
#75996=CARTESIAN_POINT('Ctrl Pts',(63.407008670507,208.645214345997,30.2872242596007)) ;
#75997=CARTESIAN_POINT('Ctrl Pts',(62.513745139331,212.120387295379,30.2872242596007)) ;
#75998=CARTESIAN_POINT('Ctrl Pts',(66.5515297315697,202.185011484147,30.3493567394431)) ;
#75999=CARTESIAN_POINT('Ctrl Pts',(64.6952653289755,205.255143987797,30.3493567394431)) ;
#76000=CARTESIAN_POINT('Ctrl Pts',(63.3784067154828,208.635344722984,30.3493567394431)) ;
#76001=CARTESIAN_POINT('Ctrl Pts',(62.4845361303434,212.112879369042,30.3493567394431)) ;
#76002=CARTESIAN_POINT('Ctrl Pts',(66.4976918481812,202.152460007516,30.3713203435596)) ;
#76003=CARTESIAN_POINT('Ctrl Pts',(64.6377860153758,205.228615184033,30.3713203435596)) ;
#76004=CARTESIAN_POINT('Ctrl Pts',(63.3187200878819,208.614834203502,30.3713203435596)) ;
#76005=CARTESIAN_POINT('Ctrl Pts',(62.4236032999988,212.097217105324,30.3713203435596)) ;
#76006=CARTESIAN_POINT('Ctrl Pts',(66.4746484362164,202.138527493107,30.3713203435596)) ;
#76007=CARTESIAN_POINT('Ctrl Pts',(64.6131863812338,205.217256553109,30.3713203435596)) ;
#76008=CARTESIAN_POINT('Ctrl Pts',(63.2931725177147,208.606058544556,30.3713203435596)) ;
#76009=CARTESIAN_POINT('Ctrl Pts',(62.39752314559,212.090513424339,30.3713203435596)) ;
#76010=CARTESIAN_POINT('',(62.5137204444978,212.120380950715,30.2513203435596)) ;
#76011=CARTESIAN_POINT('Origin',(62.39752314559,212.090513424339,30.2513203435596)) ;
#76012=CARTESIAN_POINT('Ctrl Pts',(66.5773422616064,202.200618263143,30.2513203435596)) ;
#76013=CARTESIAN_POINT('Ctrl Pts',(64.7467490262501,205.228710003766,30.2513203435596)) ;
#76014=CARTESIAN_POINT('Ctrl Pts',(63.430846523082,208.550723522602,30.2513203435596)) ;
#76015=CARTESIAN_POINT('Ctrl Pts',(62.5137204444978,212.120380950715,30.2513203435596)) ;
#76016=CARTESIAN_POINT('Ctrl Pts',(62.8448887910812,212.613106134355,30.3713203435596)) ;
#76017=CARTESIAN_POINT('Ctrl Pts',(62.7302820487196,212.624233777445,30.3713203435596)) ;
#76018=CARTESIAN_POINT('Ctrl Pts',(62.5327477139549,212.559161211515,30.3713203435596)) ;
#76019=CARTESIAN_POINT('Ctrl Pts',(62.3821824103364,212.323740151324,30.3713203435596)) ;
#76020=CARTESIAN_POINT('Ctrl Pts',(62.3784128818005,212.164860433323,30.3713203435596)) ;
#76021=CARTESIAN_POINT('Ctrl Pts',(62.39752314559,212.090513424339,30.3713203435596)) ;
#76022=CARTESIAN_POINT('Ctrl Pts',(62.8414190479705,212.57737026904,30.3713203435596)) ;
#76023=CARTESIAN_POINT('Ctrl Pts',(62.736651971145,212.587542538266,30.3713203435596)) ;
#76024=CARTESIAN_POINT('Ctrl Pts',(62.5559796234245,212.527942988847,30.3713203435596)) ;
#76025=CARTESIAN_POINT('Ctrl Pts',(62.4183338664848,212.312725587393,30.3713203435596)) ;
#76026=CARTESIAN_POINT('Ctrl Pts',(62.4148271499965,212.167415544927,30.3713203435596)) ;
#76027=CARTESIAN_POINT('Ctrl Pts',(62.4322966848017,212.099451665653,30.3713203435596)) ;
#76028=CARTESIAN_POINT('Ctrl Pts',(62.8354145860493,212.515528618039,30.3411618315345)) ;
#76029=CARTESIAN_POINT('Ctrl Pts',(62.7475491580212,212.524059836211,30.3411618315345)) ;
#76030=CARTESIAN_POINT('Ctrl Pts',(62.5961291195913,212.47419804225,30.3411618315345)) ;
#76031=CARTESIAN_POINT('Ctrl Pts',(62.480697149514,212.293710101782,30.3411618315345)) ;
#76032=CARTESIAN_POINT('Ctrl Pts',(62.4778217652515,212.171919017848,30.3411618315345)) ;
#76033=CARTESIAN_POINT('Ctrl Pts',(62.4924730106581,212.114919476352,30.3411618315345)) ;
#76034=CARTESIAN_POINT('Ctrl Pts',(62.8332920289675,212.493667802533,30.2782482805904)) ;
#76035=CARTESIAN_POINT('Ctrl Pts',(62.7514566832816,212.501613535045,30.2782482805904)) ;
#76036=CARTESIAN_POINT('Ctrl Pts',(62.6103454719125,212.455076865844,30.2782482805904)) ;
#76037=CARTESIAN_POINT('Ctrl Pts',(62.5028291668008,212.286968223387,30.2782482805904)) ;
#76038=CARTESIAN_POINT('Ctrl Pts',(62.5000993885563,212.173475037474,30.2782482805904)) ;
#76039=CARTESIAN_POINT('Ctrl Pts',(62.513745139331,212.120387295379,30.2782482805904)) ;
#76040=CARTESIAN_POINT('Ctrl Pts',(62.8332920289675,212.493667802533,30.2513203435596)) ;
#76041=CARTESIAN_POINT('Ctrl Pts',(62.7514300701379,212.501616119025,30.2513203435596)) ;
#76042=CARTESIAN_POINT('Ctrl Pts',(62.6103341167345,212.45513571479,30.2513203435596)) ;
#76043=CARTESIAN_POINT('Ctrl Pts',(62.5027874712927,212.286977814653,30.2513203435596)) ;
#76044=CARTESIAN_POINT('Ctrl Pts',(62.5000949509099,212.173492301795,30.2513203435596)) ;
#76045=CARTESIAN_POINT('Ctrl Pts',(62.513745139331,212.120387295379,30.2513203435596)) ;
#76046=CARTESIAN_POINT('',(62.8332920289675,212.493667802533,30.2513203435596)) ;
#76047=CARTESIAN_POINT('Ctrl Pts',(62.513745139331,212.120387295379,30.2513203435596)) ;
#76048=CARTESIAN_POINT('Ctrl Pts',(62.5000949509099,212.173492301795,30.2513203435596)) ;
#76049=CARTESIAN_POINT('Ctrl Pts',(62.5027874712927,212.286977814653,30.2513203435596)) ;
#76050=CARTESIAN_POINT('Ctrl Pts',(62.6103341167345,212.45513571479,30.2513203435596)) ;
#76051=CARTESIAN_POINT('Ctrl Pts',(62.7514300701379,212.501616119025,30.2513203435596)) ;
#76052=CARTESIAN_POINT('Ctrl Pts',(62.8332920289675,212.493667802533,30.2513203435596)) ;
#76053=CARTESIAN_POINT('Origin',(62.8448887910812,212.613106134355,30.2513203435596)) ;
#76054=CARTESIAN_POINT('Origin',(65.7730634668025,212.328797532388,30.2513203435596)) ;
#76055=CARTESIAN_POINT('',(69.2315751790255,211.872432002476,30.2513203435596)) ;
#76056=CARTESIAN_POINT('Origin',(69.2431719411391,211.991870334298,30.2513203435596)) ;
#76057=CARTESIAN_POINT('',(65.7614667046888,212.209359200566,30.2513203435596)) ;
#76058=CARTESIAN_POINT('Ctrl Pts',(69.6168298215689,211.643116744604,30.3713203435596)) ;
#76059=CARTESIAN_POINT('Ctrl Pts',(69.6038817585733,211.72053657915,30.3713203435596)) ;
#76060=CARTESIAN_POINT('Ctrl Pts',(69.5217274044295,211.89264098624,30.3713203435596)) ;
#76061=CARTESIAN_POINT('Ctrl Pts',(69.3473422258095,211.981756010092,30.3713203435596)) ;
#76062=CARTESIAN_POINT('Ctrl Pts',(69.2431719411391,211.991870334298,30.3713203435596)) ;
#76063=CARTESIAN_POINT('Ctrl Pts',(69.5814177423463,211.637194259297,30.3713203435596)) ;
#76064=CARTESIAN_POINT('Ctrl Pts',(69.5695813470117,211.707967143915,30.3713203435596)) ;
#76065=CARTESIAN_POINT('Ctrl Pts',(69.4944320015214,211.865340586305,30.3713203435596)) ;
#76066=CARTESIAN_POINT('Ctrl Pts',(69.3349288486785,211.946888519231,30.3713203435596)) ;
#76067=CARTESIAN_POINT('Ctrl Pts',(69.2397021980285,211.956134468983,30.3713203435596)) ;
#76068=CARTESIAN_POINT('Ctrl Pts',(69.5201364960134,211.626945290895,30.3411617587246)) ;
#76069=CARTESIAN_POINT('Ctrl Pts',(69.5102096184685,211.686300672263,30.3411617587246)) ;
#76070=CARTESIAN_POINT('Ctrl Pts',(69.4472360221651,211.818236948212,30.3411617587246)) ;
#76071=CARTESIAN_POINT('Ctrl Pts',(69.3135618647732,211.886538566864,30.3411617587246)) ;
#76072=CARTESIAN_POINT('Ctrl Pts',(69.2336977445498,211.894292904935,30.3411617587246)) ;
#76073=CARTESIAN_POINT('Ctrl Pts',(69.4984736650468,211.623322295552,30.2782482805904)) ;
#76074=CARTESIAN_POINT('Ctrl Pts',(69.4892280553263,211.678604199499,30.2782482805904)) ;
#76075=CARTESIAN_POINT('Ctrl Pts',(69.4305350897576,211.801524301052,30.2782482805904)) ;
#76076=CARTESIAN_POINT('Ctrl Pts',(69.3059583355531,211.865209833861,30.2782482805904)) ;
#76077=CARTESIAN_POINT('Ctrl Pts',(69.2315751790255,211.872432002476,30.2782482805904)) ;
#76078=CARTESIAN_POINT('Ctrl Pts',(69.4984736650468,211.623322295552,30.2513203435596)) ;
#76079=CARTESIAN_POINT('Ctrl Pts',(69.4892250486213,211.67862217737,30.2513203435596)) ;
#76080=CARTESIAN_POINT('Ctrl Pts',(69.43054336709,211.80155389672,30.2513203435596)) ;
#76081=CARTESIAN_POINT('Ctrl Pts',(69.3059825252186,211.865207485186,30.2513203435596)) ;
#76082=CARTESIAN_POINT('Ctrl Pts',(69.2315751790255,211.872432002476,30.2513203435596)) ;
#76083=CARTESIAN_POINT('',(69.4984736650468,211.623322295552,30.2513203435596)) ;
#76084=CARTESIAN_POINT('Ctrl Pts',(69.2315751790255,211.872432002476,30.2513203435596)) ;
#76085=CARTESIAN_POINT('Ctrl Pts',(69.3059825252186,211.865207485186,30.2513203435596)) ;
#76086=CARTESIAN_POINT('Ctrl Pts',(69.43054336709,211.80155389672,30.2513203435596)) ;
#76087=CARTESIAN_POINT('Ctrl Pts',(69.4892250486213,211.67862217737,30.2513203435596)) ;
#76088=CARTESIAN_POINT('Ctrl Pts',(69.4984736650468,211.623322295552,30.2513203435596)) ;
#76089=CARTESIAN_POINT('Origin',(69.6168298215689,211.643116744604,30.2513203435596)) ;
#76090=CARTESIAN_POINT('Ctrl Pts',(69.4984736650468,211.623322295552,30.2513203435596)) ;
#76091=CARTESIAN_POINT('Ctrl Pts',(70.0304244797463,208.442650091984,30.2513203435596)) ;
#76092=CARTESIAN_POINT('Ctrl Pts',(71.0956312780117,205.355998860028,30.2513203435596)) ;
#76093=CARTESIAN_POINT('Ctrl Pts',(72.5775641491993,202.49377028534,30.2513203435596)) ;
#76094=CARTESIAN_POINT('Ctrl Pts',(69.4984736650468,211.623322295552,30.2872242596007)) ;
#76095=CARTESIAN_POINT('Ctrl Pts',(70.0304311821308,208.442610016684,30.2872242596007)) ;
#76096=CARTESIAN_POINT('Ctrl Pts',(71.095615141615,205.35603002612,30.2872242596007)) ;
#76097=CARTESIAN_POINT('Ctrl Pts',(72.5775641491993,202.49377028534,30.2872242596007)) ;
#76098=CARTESIAN_POINT('Ctrl Pts',(69.5282191152938,211.628297066757,30.3493566400793)) ;
#76099=CARTESIAN_POINT('Ctrl Pts',(70.059641309941,208.450785619898,30.3493566400793)) ;
#76100=CARTESIAN_POINT('Ctrl Pts',(71.1236857344122,205.367407169992,30.3493566400794)) ;
#76101=CARTESIAN_POINT('Ctrl Pts',(72.6043459208053,202.507636678836,30.3493566400794)) ;
#76102=CARTESIAN_POINT('Ctrl Pts',(69.590270762152,211.638674880624,30.3713203435596)) ;
#76103=CARTESIAN_POINT('Ctrl Pts',(70.1205940095398,208.467734325105,30.3713203435596)) ;
#76104=CARTESIAN_POINT('Ctrl Pts',(71.1822006669159,205.391223591054,30.3713203435596)) ;
#76105=CARTESIAN_POINT('Ctrl Pts',(72.660215071218,202.536563205255,30.3713203435596)) ;
#76106=CARTESIAN_POINT('Ctrl Pts',(69.616829821569,211.643116744604,30.3713203435596)) ;
#76107=CARTESIAN_POINT('Ctrl Pts',(70.1466834166504,208.474984362312,30.3713203435596)) ;
#76108=CARTESIAN_POINT('Ctrl Pts',(71.207244239121,205.401420705868,30.3713203435596)) ;
#76109=CARTESIAN_POINT('Ctrl Pts',(72.6841279270487,202.548944203549,30.3713203435596)) ;
#76110=CARTESIAN_POINT('',(72.5775641491992,202.49377028534,30.2513203435596)) ;
#76111=CARTESIAN_POINT('Origin',(72.6841279270487,202.548944203549,30.2513203435596)) ;
#76112=CARTESIAN_POINT('Ctrl Pts',(69.4984736650468,211.623322295552,30.2513203435596)) ;
#76113=CARTESIAN_POINT('Ctrl Pts',(70.0304244797463,208.442650091984,30.2513203435596)) ;
#76114=CARTESIAN_POINT('Ctrl Pts',(71.0956312780117,205.355998860028,30.2513203435596)) ;
#76115=CARTESIAN_POINT('Ctrl Pts',(72.5775641491993,202.49377028534,30.2513203435596)) ;
#76116=CARTESIAN_POINT('Ctrl Pts',(72.3111547045756,201.93583548982,30.3713203435596)) ;
#76117=CARTESIAN_POINT('Ctrl Pts',(72.434062830227,201.93583548982,30.3713203435596)) ;
#76118=CARTESIAN_POINT('Ctrl Pts',(72.6367193429415,202.032109677482,30.3713203435596)) ;
#76119=CARTESIAN_POINT('Ctrl Pts',(72.7529836107094,202.308661221514,30.3713203435596)) ;
#76120=CARTESIAN_POINT('Ctrl Pts',(72.7218019430032,202.476180013561,30.3713203435596)) ;
#76121=CARTESIAN_POINT('Ctrl Pts',(72.6841279270486,202.548944203549,30.3713203435596)) ;
#76122=CARTESIAN_POINT('Ctrl Pts',(72.3111547045756,201.971739405861,30.3713203435596)) ;
#76123=CARTESIAN_POINT('Ctrl Pts',(72.4235104419194,201.971739405861,30.3713203435596)) ;
#76124=CARTESIAN_POINT('Ctrl Pts',(72.6088489992096,202.05988145465,30.3713203435596)) ;
#76125=CARTESIAN_POINT('Ctrl Pts',(72.7151374364996,202.312699539834,30.3713203435596)) ;
#76126=CARTESIAN_POINT('Ctrl Pts',(72.6866835985101,202.465919251188,30.3713203435596)) ;
#76127=CARTESIAN_POINT('Ctrl Pts',(72.6522441192743,202.532436205824,30.3713203435596)) ;
#76128=CARTESIAN_POINT('Ctrl Pts',(72.3111547045756,202.033871875492,30.3411618343582)) ;
#76129=CARTESIAN_POINT('Ctrl Pts',(72.4053845452112,202.033871875492,30.3411618343582)) ;
#76130=CARTESIAN_POINT('Ctrl Pts',(72.5607354838846,202.107650247836,30.3411618343582)) ;
#76131=CARTESIAN_POINT('Ctrl Pts',(72.6498702107552,202.319671293231,30.3411618343582)) ;
#76132=CARTESIAN_POINT('Ctrl Pts',(72.6259520275162,202.448082730821,30.3411618343582)) ;
#76133=CARTESIAN_POINT('Ctrl Pts',(72.5970685301829,202.503868774178,30.3411618343582)) ;
#76134=CARTESIAN_POINT('Ctrl Pts',(72.3111547045756,202.05583548982,30.2782482805904)) ;
#76135=CARTESIAN_POINT('Ctrl Pts',(72.3989176820674,202.05583548982,30.2782482805904)) ;
#76136=CARTESIAN_POINT('Ctrl Pts',(72.5436762466237,202.124664150233,30.2782482805904)) ;
#76137=CARTESIAN_POINT('Ctrl Pts',(72.6266990056788,202.322143095839,30.2782482805904)) ;
#76138=CARTESIAN_POINT('Ctrl Pts',(72.6044654122095,202.441812760691,30.2782482805904)) ;
#76139=CARTESIAN_POINT('Ctrl Pts',(72.5775641491992,202.49377028534,30.2782482805904)) ;
#76140=CARTESIAN_POINT('Ctrl Pts',(72.3111547045756,202.05583548982,30.2513203435596)) ;
#76141=CARTESIAN_POINT('Ctrl Pts',(72.398946222898,202.05583548982,30.2513203435596)) ;
#76142=CARTESIAN_POINT('Ctrl Pts',(72.543700874837,202.124602766721,30.2513203435596)) ;
#76143=CARTESIAN_POINT('Ctrl Pts',(72.6267467803854,202.322139583887,30.2513203435596)) ;
#76144=CARTESIAN_POINT('Ctrl Pts',(72.6044741605953,202.44179586392,30.2513203435596)) ;
#76145=CARTESIAN_POINT('Ctrl Pts',(72.5775641491992,202.49377028534,30.2513203435596)) ;
#76146=CARTESIAN_POINT('Ctrl Pts',(72.5775641491992,202.49377028534,30.2513203435596)) ;
#76147=CARTESIAN_POINT('Ctrl Pts',(72.6044741605953,202.44179586392,30.2513203435596)) ;
#76148=CARTESIAN_POINT('Ctrl Pts',(72.6267467803854,202.322139583887,30.2513203435596)) ;
#76149=CARTESIAN_POINT('Ctrl Pts',(72.543700874837,202.124602766721,30.2513203435596)) ;
#76150=CARTESIAN_POINT('Ctrl Pts',(72.398946222898,202.05583548982,30.2513203435596)) ;
#76151=CARTESIAN_POINT('Ctrl Pts',(72.3111547045756,202.05583548982,30.2513203435596)) ;
#76152=CARTESIAN_POINT('Ctrl Pts',(62.8332920289675,212.493667802533,30.2513203435596)) ;
#76153=CARTESIAN_POINT('Ctrl Pts',(62.8332920289675,212.493667802533,22.1393203435596)) ;
#76154=CARTESIAN_POINT('Ctrl Pts',(62.7787149126794,212.498966920703,30.2513203435596)) ;
#76155=CARTESIAN_POINT('Ctrl Pts',(62.7787149126794,212.498966920703,22.1393203435596)) ;
#76156=CARTESIAN_POINT('Ctrl Pts',(62.6669957149089,212.478811797326,30.2513203435596)) ;
#76157=CARTESIAN_POINT('Ctrl Pts',(62.6669957149089,212.478811797326,22.1393203435596)) ;
#76158=CARTESIAN_POINT('Ctrl Pts',(62.5174244243077,212.346623344547,30.2513203435596)) ;
#76159=CARTESIAN_POINT('Ctrl Pts',(62.5174244243077,212.346623344547,22.1393203435596)) ;
#76160=CARTESIAN_POINT('Ctrl Pts',(62.4932689273543,212.200048420549,30.2513203435596)) ;
#76161=CARTESIAN_POINT('Ctrl Pts',(62.4932689273543,212.200048420549,22.1393203435596)) ;
#76162=CARTESIAN_POINT('Ctrl Pts',(62.513745139331,212.120387295379,30.2513203435596)) ;
#76163=CARTESIAN_POINT('Ctrl Pts',(62.513745139331,212.120387295379,22.1393203435596)) ;
#76164=CARTESIAN_POINT('',(62.5137204444978,212.120380950715,23.4913203435596)) ;
#76165=CARTESIAN_POINT('',(62.513745139331,212.120387295379,30.2513203435596)) ;
#76166=CARTESIAN_POINT('',(62.8332920289675,212.493667802533,23.4913203435596)) ;
#76167=CARTESIAN_POINT('Ctrl Pts',(62.8332920289675,212.493667802533,23.4913203435596)) ;
#76168=CARTESIAN_POINT('Ctrl Pts',(62.7787149126794,212.498966920703,23.4913203435596)) ;
#76169=CARTESIAN_POINT('Ctrl Pts',(62.6669957149089,212.478811797326,23.4913203435596)) ;
#76170=CARTESIAN_POINT('Ctrl Pts',(62.5174244243077,212.346623344547,23.4913203435596)) ;
#76171=CARTESIAN_POINT('Ctrl Pts',(62.4932689273543,212.200048420549,23.4913203435596)) ;
#76172=CARTESIAN_POINT('Ctrl Pts',(62.513745139331,212.120387295379,23.4913203435596)) ;
#76173=CARTESIAN_POINT('',(62.8332920289675,212.493667802533,23.4913203435596)) ;
#76174=CARTESIAN_POINT('Ctrl Pts',(66.6653986331397,202.05583548982,17.8547522895864)) ;
#76175=CARTESIAN_POINT('Ctrl Pts',(66.6653986331397,202.05583548982,32.8746339543542)) ;
#76176=CARTESIAN_POINT('Ctrl Pts',(64.7175672988148,205.239235006074,17.8547522895864)) ;
#76177=CARTESIAN_POINT('Ctrl Pts',(64.7175672988148,205.239235006074,32.8746339543542)) ;
#76178=CARTESIAN_POINT('Ctrl Pts',(63.3441806268929,208.750326110011,17.8547522895864)) ;
#76179=CARTESIAN_POINT('Ctrl Pts',(63.3441806268929,208.750326110011,32.8746339543542)) ;
#76180=CARTESIAN_POINT('Ctrl Pts',(62.4092970952969,212.53483522599,17.8547522895864)) ;
#76181=CARTESIAN_POINT('Ctrl Pts',(62.4092970952969,212.53483522599,32.8746339543542)) ;
#76182=CARTESIAN_POINT('',(66.5773388238817,202.200616184912,23.4913203435596)) ;
#76183=CARTESIAN_POINT('',(66.5773376779735,202.200615492168,23.4913203435596)) ;
#76184=CARTESIAN_POINT('Ctrl Pts',(62.5137204444978,212.120380950715,23.4913203435596)) ;
#76185=CARTESIAN_POINT('Ctrl Pts',(63.430846523082,208.550723522602,23.4913203435596)) ;
#76186=CARTESIAN_POINT('Ctrl Pts',(64.7467490262501,205.228710003766,23.4913203435596)) ;
#76187=CARTESIAN_POINT('Ctrl Pts',(66.5773422616064,202.200618263143,23.4913203435596)) ;
#76188=CARTESIAN_POINT('Ctrl Pts',(66.5773376779735,202.200615492168,30.2513203435596)) ;
#76189=CARTESIAN_POINT('Ctrl Pts',(66.5773376779735,202.200615492168,22.1393203435596)) ;
#76190=CARTESIAN_POINT('Ctrl Pts',(66.6304739575799,202.112731773171,30.2513203435596)) ;
#76191=CARTESIAN_POINT('Ctrl Pts',(66.6304739575799,202.112731773171,22.1393203435596)) ;
#76192=CARTESIAN_POINT('Ctrl Pts',(66.7313621344916,202.05583548982,30.2513203435596)) ;
#76193=CARTESIAN_POINT('Ctrl Pts',(66.7313621344916,202.05583548982,22.1393203435596)) ;
#76194=CARTESIAN_POINT('Ctrl Pts',(66.8340607823661,202.05583548982,30.2513203435596)) ;
#76195=CARTESIAN_POINT('Ctrl Pts',(66.8340607823661,202.05583548982,22.1393203435596)) ;
#76196=CARTESIAN_POINT('',(66.8340607823661,202.05583548982,23.4913203435596)) ;
#76197=CARTESIAN_POINT('',(66.8340607823661,202.05583548982,30.2513203435596)) ;
#76198=CARTESIAN_POINT('Origin',(66.7985154459218,202.29280669461,23.4913203435596)) ;
#76199=CARTESIAN_POINT('Origin',(72.8081914673101,202.05583548982,23.8713203435596)) ;
#76200=CARTESIAN_POINT('',(72.3111547045756,202.05583548982,23.4913203435596)) ;
#76201=CARTESIAN_POINT('',(72.3111547045756,202.05583548982,23.4913203435596)) ;
#76202=CARTESIAN_POINT('',(70.2085194795435,202.05583548982,23.4913203435596)) ;
#76203=CARTESIAN_POINT('Origin',(64.1568347953872,220.146231446812,30.2513203435596)) ;
#76204=CARTESIAN_POINT('',(66.1568347953872,220.146231446812,30.2513203435596)) ;
#76205=CARTESIAN_POINT('Origin',(66.2768347953872,220.146231446812,30.2513203435596)) ;
#76206=CARTESIAN_POINT('Origin',(64.1568347953872,220.146231446812,30.2513203435596)) ;
#76207=CARTESIAN_POINT('Origin',(64.1568347953872,220.146231446812,23.8713203435596)) ;
#76208=CARTESIAN_POINT('',(66.1568347953872,220.146231446812,23.8713203435596)) ;
#76209=CARTESIAN_POINT('Origin',(64.1568347953872,220.146231446812,23.8713203435596)) ;
#76210=CARTESIAN_POINT('',(66.1568347953872,220.146231446812,23.8713203435596)) ;
#76211=CARTESIAN_POINT('Origin',(60.7116108526749,219.132346607579,30.2513203435596)) ;
#76212=CARTESIAN_POINT('',(60.5916108526749,220.645409008718,30.2513203435596)) ;
#76213=CARTESIAN_POINT('Origin',(60.711617364105,220.636941531386,30.2513105111323)) ;
#76214=CARTESIAN_POINT('',(60.5916108526749,219.647053884905,30.2513203435596)) ;
#76215=CARTESIAN_POINT('',(60.5916108526749,219.132346607579,30.2513203435596)) ;
#76216=CARTESIAN_POINT('Origin',(60.7116173641052,219.655521362237,30.251310511132)) ;
#76217=CARTESIAN_POINT('Origin',(64.1568347953872,220.146231446812,30.2513203435596)) ;
#76218=CARTESIAN_POINT('',(64.9830939940346,223.650128668,30.2513203435596)) ;
#76219=CARTESIAN_POINT('Ctrl Pts',(64.9314996085946,223.538913929329,30.3713203435596)) ;
#76220=CARTESIAN_POINT('Ctrl Pts',(64.9317215230365,223.539394529153,30.3713203435596)) ;
#76221=CARTESIAN_POINT('Ctrl Pts',(64.9319434468761,223.539875119568,30.3713169902839)) ;
#76222=CARTESIAN_POINT('Ctrl Pts',(64.9321653661535,223.540355670364,30.3713102838073)) ;
#76223=CARTESIAN_POINT('Ctrl Pts',(64.9390997545165,223.555371607189,30.3711007242144)) ;
#76224=CARTESIAN_POINT('Ctrl Pts',(64.945967748304,223.570213670412,30.3676189963526)) ;
#76225=CARTESIAN_POINT('Ctrl Pts',(64.9523490912924,223.583980936494,30.3610416978447)) ;
#76226=CARTESIAN_POINT('Ctrl Pts',(64.9584600142363,223.59716479173,30.3547431233232)) ;
#76227=CARTESIAN_POINT('Ctrl Pts',(64.9640174018536,223.609132151157,30.3457154332298)) ;
#76228=CARTESIAN_POINT('Ctrl Pts',(64.9686896141286,223.619182598841,30.3344093373863)) ;
#76229=CARTESIAN_POINT('Ctrl Pts',(64.9732616895214,223.629017640966,30.3233455586983)) ;
#76230=CARTESIAN_POINT('Ctrl Pts',(64.9768987673375,223.636829737302,30.3103090834608)) ;
#76231=CARTESIAN_POINT('Ctrl Pts',(64.9793767861943,223.6421501932,30.295975639056)) ;
#76232=CARTESIAN_POINT('Ctrl Pts',(64.9818281519998,223.647413423391,30.2817963621737)) ;
#76233=CARTESIAN_POINT('Ctrl Pts',(64.9830939940349,223.650128668,30.2666404537853)) ;
#76234=CARTESIAN_POINT('Ctrl Pts',(64.9830939940347,223.650128668,30.2513203435596)) ;
#76235=CARTESIAN_POINT('Origin',(64.1568347953872,220.146231446812,30.2513203435596)) ;
#76236=CARTESIAN_POINT('Origin',(70.5636770849813,219.33964171939,30.2513203435596)) ;
#76237=CARTESIAN_POINT('',(70.3850625789433,219.622496965577,30.2513203435596)) ;
#76238=CARTESIAN_POINT('Ctrl Pts',(70.260001179114,219.566058198626,30.3713203435596)) ;
#76239=CARTESIAN_POINT('Ctrl Pts',(70.2603043870942,219.566201490721,30.3713203435588)) ;
#76240=CARTESIAN_POINT('Ctrl Pts',(70.2606076475466,219.566344671311,30.3713192475164)) ;
#76241=CARTESIAN_POINT('Ctrl Pts',(70.2756119803025,219.573422118245,30.3712108698978)) ;
#76242=CARTESIAN_POINT('Ctrl Pts',(70.2904565326987,219.580094181022,30.3685339483272)) ;
#76243=CARTESIAN_POINT('Ctrl Pts',(70.3148096110176,219.590914525823,30.3596445675472)) ;
#76244=CARTESIAN_POINT('Ctrl Pts',(70.3303650868265,219.597736373691,30.3526122298557)) ;
#76245=CARTESIAN_POINT('Ctrl Pts',(70.3569751848126,219.610042404231,30.3283757793828)) ;
#76246=CARTESIAN_POINT('Ctrl Pts',(70.366511706138,219.614483226237,30.3157125984337)) ;
#76247=CARTESIAN_POINT('Ctrl Pts',(70.3771460617663,219.619205734236,30.2935959336947)) ;
#76248=CARTESIAN_POINT('Ctrl Pts',(70.3800723202718,219.620457756702,30.2854122779805)) ;
#76249=CARTESIAN_POINT('Ctrl Pts',(70.3840287602576,219.622101846434,30.2685540701959)) ;
#76250=CARTESIAN_POINT('Ctrl Pts',(70.3850625789433,219.622496965577,30.2599631560588)) ;
#76251=CARTESIAN_POINT('Ctrl Pts',(70.3850625789433,219.622496965577,30.2513203435596)) ;
#76252=CARTESIAN_POINT('',(70.6354050204722,219.435845166679,30.2513203435596)) ;
#76253=CARTESIAN_POINT('Ctrl Pts',(70.3022814706893,218.330941191344,30.2513203435596)) ;
#76254=CARTESIAN_POINT('Ctrl Pts',(70.3215247358121,218.761924034176,30.2513203435596)) ;
#76255=CARTESIAN_POINT('Ctrl Pts',(70.3491825816751,219.192547142136,30.2513203435596)) ;
#76256=CARTESIAN_POINT('Ctrl Pts',(70.3850625789433,219.622496965577,30.2513203435596)) ;
#76257=CARTESIAN_POINT('Ctrl Pts',(70.3022814706893,218.330941191344,30.2872242596007)) ;
#76258=CARTESIAN_POINT('Ctrl Pts',(70.3215245131287,218.761919046833,30.2872242596007)) ;
#76259=CARTESIAN_POINT('Ctrl Pts',(70.3491829883129,219.192552014874,30.2872242596007)) ;
#76260=CARTESIAN_POINT('Ctrl Pts',(70.3850625789433,219.622496965577,30.2872242596007)) ;
#76261=CARTESIAN_POINT('Ctrl Pts',(70.2721528021911,218.332286428087,30.3493565173742)) ;
#76262=CARTESIAN_POINT('Ctrl Pts',(70.2914136304585,218.763662624851,30.3493565173742)) ;
#76263=CARTESIAN_POINT('Ctrl Pts',(70.3190962939392,219.194670899254,30.3493565173742)) ;
#76264=CARTESIAN_POINT('Ctrl Pts',(70.3550083629108,219.625005037752,30.3493565173742)) ;
#76265=CARTESIAN_POINT('Ctrl Pts',(70.2093020433682,218.335092697142,30.3713203435596)) ;
#76266=CARTESIAN_POINT('Ctrl Pts',(70.228599383625,218.767286636677,30.3713203435596)) ;
#76267=CARTESIAN_POINT('Ctrl Pts',(70.2563341749771,219.199103982098,30.3713203435596)) ;
#76268=CARTESIAN_POINT('Ctrl Pts',(70.2923129177541,219.630237072465,30.3713203435596)) ;
#76269=CARTESIAN_POINT('Ctrl Pts',(70.1824009080094,218.33629382542,30.3713203435596)) ;
#76270=CARTESIAN_POINT('Ctrl Pts',(70.2017138522361,218.768837240123,30.3713203435596)) ;
#76271=CARTESIAN_POINT('Ctrl Pts',(70.2294710222708,219.201001932499,30.3713203435596)) ;
#76272=CARTESIAN_POINT('Ctrl Pts',(70.2654782591418,219.632476467448,30.3713203435596)) ;
#76273=CARTESIAN_POINT('',(70.3022814706893,218.330941191344,30.2513203435596)) ;
#76274=CARTESIAN_POINT('Origin',(70.1824009080094,218.33629382542,30.2513203435596)) ;
#76275=CARTESIAN_POINT('Origin',(103.767178705384,216.834469413406,30.2513203435596)) ;
#76276=CARTESIAN_POINT('Ctrl Pts',(70.2813572214291,216.003852832276,30.2513203435596)) ;
#76277=CARTESIAN_POINT('Ctrl Pts',(70.2602736675229,216.779393400763,30.2513203435596)) ;
#76278=CARTESIAN_POINT('Ctrl Pts',(70.2676697182798,217.555757180025,30.2513203435596)) ;
#76279=CARTESIAN_POINT('Ctrl Pts',(70.3022814706893,218.330941191344,30.2513203435596)) ;
#76280=CARTESIAN_POINT('Ctrl Pts',(70.2813572214291,216.003852832276,30.2872242596007)) ;
#76281=CARTESIAN_POINT('Ctrl Pts',(70.2602739227663,216.779384011854,30.2872242596007)) ;
#76282=CARTESIAN_POINT('Ctrl Pts',(70.2676701188078,217.555766150471,30.2872242596007)) ;
#76283=CARTESIAN_POINT('Ctrl Pts',(70.3022814706893,218.330941191344,30.2872242596007)) ;
#76284=CARTESIAN_POINT('Ctrl Pts',(70.2512096898405,216.003033252833,30.3493565363917)) ;
#76285=CARTESIAN_POINT('Ctrl Pts',(70.2301060047771,216.779314328785,30.3493565363917)) ;
#76286=CARTESIAN_POINT('Ctrl Pts',(70.2375094757991,217.556394913003,30.3493565363917)) ;
#76287=CARTESIAN_POINT('Ctrl Pts',(70.2721528180251,218.33228642738,30.3493565363917)) ;
#76288=CARTESIAN_POINT('Ctrl Pts',(70.1883195322401,216.001323544686,30.3713203435596)) ;
#76289=CARTESIAN_POINT('Ctrl Pts',(70.1671739965509,216.779144060255,30.3713203435596)) ;
#76290=CARTESIAN_POINT('Ctrl Pts',(70.1745930291305,217.557730355953,30.3713203435596)) ;
#76291=CARTESIAN_POINT('Ctrl Pts',(70.2093020433682,218.335092697142,30.3713203435596)) ;
#76292=CARTESIAN_POINT('Ctrl Pts',(70.1614015403524,216.000591762293,30.3713203435596)) ;
#76293=CARTESIAN_POINT('Ctrl Pts',(70.1402381191435,216.779070181469,30.3713203435596)) ;
#76294=CARTESIAN_POINT('Ctrl Pts',(70.14766382781,217.558302903379,30.3713203435596)) ;
#76295=CARTESIAN_POINT('Ctrl Pts',(70.1824009080094,218.33629382542,30.3713203435596)) ;
#76296=CARTESIAN_POINT('',(70.2813572214291,216.003852832276,30.2513203435596)) ;
#76297=CARTESIAN_POINT('Origin',(70.1614015403524,216.000591762293,30.2513203435596)) ;
#76298=CARTESIAN_POINT('Origin',(99.1329946690443,222.962162901317,30.2513203435596)) ;
#76299=CARTESIAN_POINT('Ctrl Pts',(70.4779346423502,213.258471670562,30.2513203435596)) ;
#76300=CARTESIAN_POINT('Ctrl Pts',(70.3711537499326,214.169914953712,30.2513203435596)) ;
#76301=CARTESIAN_POINT('Ctrl Pts',(70.3063010559943,215.086315128482,30.2513203435596)) ;
#76302=CARTESIAN_POINT('Ctrl Pts',(70.2813572214291,216.003852832275,30.2513203435596)) ;
#76303=CARTESIAN_POINT('Ctrl Pts',(70.4779346423502,213.258471670562,30.2872242596007)) ;
#76304=CARTESIAN_POINT('Ctrl Pts',(70.3711551172064,214.169903283155,30.2872242596007)) ;
#76305=CARTESIAN_POINT('Ctrl Pts',(70.3063007540173,215.086326236448,30.2872242596007)) ;
#76306=CARTESIAN_POINT('Ctrl Pts',(70.2813572214291,216.003852832275,30.2872242596007)) ;
#76307=CARTESIAN_POINT('Ctrl Pts',(70.4479808643574,213.254962410903,30.3493565692531)) ;
#76308=CARTESIAN_POINT('Ctrl Pts',(70.3410921344475,214.167326156092,30.3493565692531)) ;
#76309=CARTESIAN_POINT('Ctrl Pts',(70.2761773688426,215.084619459547,30.3493565692531)) ;
#76310=CARTESIAN_POINT('Ctrl Pts',(70.2512097172181,216.003033253576,30.3493565692531)) ;
#76311=CARTESIAN_POINT('Ctrl Pts',(70.3854948082789,213.247641805271,30.3713203435596)) ;
#76312=CARTESIAN_POINT('Ctrl Pts',(70.2783818952035,214.161919097311,30.3713203435596)) ;
#76313=CARTESIAN_POINT('Ctrl Pts',(70.2133366971056,215.081088448267,30.3713203435596)) ;
#76314=CARTESIAN_POINT('Ctrl Pts',(70.1883195322401,216.001323544685,30.3713203435596)) ;
#76315=CARTESIAN_POINT('Ctrl Pts',(70.3587497899394,213.244508470505,30.3713203435596)) ;
#76316=CARTESIAN_POINT('Ctrl Pts',(70.2515410686806,214.159603546732,30.3713203435596)) ;
#76317=CARTESIAN_POINT('Ctrl Pts',(70.1864398654763,215.079578303801,30.3713203435596)) ;
#76318=CARTESIAN_POINT('Ctrl Pts',(70.1614015403525,216.000591762292,30.3713203435596)) ;
#76319=CARTESIAN_POINT('',(70.4779346423502,213.258471670562,30.2513203435596)) ;
#76320=CARTESIAN_POINT('Origin',(70.3587497899394,213.244508470505,30.2513203435596)) ;
#76321=CARTESIAN_POINT('Origin',(97.5077297790289,222.403214896199,30.2513203435596)) ;
#76322=CARTESIAN_POINT('Ctrl Pts',(74.1761041106882,202.05583548982,30.2513203435596)) ;
#76323=CARTESIAN_POINT('Ctrl Pts',(73.3476211486845,203.537657612761,30.2513203435596)) ;
#76324=CARTESIAN_POINT('Ctrl Pts',(71.6591598866693,207.13437740547,30.2513203435596)) ;
#76325=CARTESIAN_POINT('Ctrl Pts',(70.7411453681046,211.011799605831,30.2513203435596)) ;
#76326=CARTESIAN_POINT('Ctrl Pts',(70.4779346423502,213.258471670562,30.2513203435596)) ;
#76327=CARTESIAN_POINT('Ctrl Pts',(74.1761041106882,202.05583548982,30.2872242596007)) ;
#76328=CARTESIAN_POINT('Ctrl Pts',(73.3476299244953,203.537641916373,30.2872242596007)) ;
#76329=CARTESIAN_POINT('Ctrl Pts',(71.6591726184549,207.134367457936,30.2872242596007)) ;
#76330=CARTESIAN_POINT('Ctrl Pts',(70.7411419978282,211.011828373298,30.2872242596007)) ;
#76331=CARTESIAN_POINT('Ctrl Pts',(70.4779346423502,213.258471670562,30.2872242596007)) ;
#76332=CARTESIAN_POINT('Ctrl Pts',(74.1497804176814,202.041117980333,30.3493566054646)) ;
#76333=CARTESIAN_POINT('Ctrl Pts',(73.3206053035724,203.524178084438,30.3493566054646)) ;
#76334=CARTESIAN_POINT('Ctrl Pts',(71.630469640981,207.124386091449,30.3493566054646)) ;
#76335=CARTESIAN_POINT('Ctrl Pts',(70.7114574352898,211.006021446736,30.3493566054646)) ;
#76336=CARTESIAN_POINT('Ctrl Pts',(70.4479808943322,213.254962414415,30.3493566054646)) ;
#76337=CARTESIAN_POINT('Ctrl Pts',(74.0948669375559,202.010415993931,30.3713203435596)) ;
#76338=CARTESIAN_POINT('Ctrl Pts',(73.2642529097014,203.496049734815,30.3713203435596)) ;
#76339=CARTESIAN_POINT('Ctrl Pts',(71.5706265465599,207.103537714816,30.3713203435596)) ;
#76340=CARTESIAN_POINT('Ctrl Pts',(70.6495239519761,210.993984019407,30.3713203435596)) ;
#76341=CARTESIAN_POINT('Ctrl Pts',(70.3854948082789,213.247641805271,30.3713203435596)) ;
#76342=CARTESIAN_POINT('Ctrl Pts',(74.0713631125318,201.997275065426,30.3713203435596)) ;
#76343=CARTESIAN_POINT('Ctrl Pts',(73.2401341423739,203.484008690256,30.3713203435596)) ;
#76344=CARTESIAN_POINT('Ctrl Pts',(71.5450141265831,207.094613224745,30.3713203435596)) ;
#76345=CARTESIAN_POINT('Ctrl Pts',(70.6230150970638,210.988834878587,30.3713203435596)) ;
#76346=CARTESIAN_POINT('Ctrl Pts',(70.3587497899395,213.244508470505,30.3713203435596)) ;
#76347=CARTESIAN_POINT('',(74.1761041106883,202.05583548982,30.2513203435596)) ;
#76348=CARTESIAN_POINT('Origin',(74.0713631125318,201.997275065426,30.2513203435596)) ;
#76349=CARTESIAN_POINT('Ctrl Pts',(74.1761041106882,202.05583548982,30.2513203435596)) ;
#76350=CARTESIAN_POINT('Ctrl Pts',(73.9471261103511,202.465384849466,30.2513203435596)) ;
#76351=CARTESIAN_POINT('Ctrl Pts',(73.4020528825475,203.478780571653,30.2513203435596)) ;
#76352=CARTESIAN_POINT('Ctrl Pts',(72.6149447082149,205.101979283954,30.2513203435596)) ;
#76353=CARTESIAN_POINT('Ctrl Pts',(71.7263234125876,207.330523545477,30.2513203435596)) ;
#76354=CARTESIAN_POINT('Ctrl Pts',(71.0883402872662,209.579226496892,30.2513203435596)) ;
#76355=CARTESIAN_POINT('Ctrl Pts',(70.7249576044374,211.422049476544,30.2513203435596)) ;
#76356=CARTESIAN_POINT('Ctrl Pts',(70.5491399848247,212.650688483389,30.2513203435596)) ;
#76357=CARTESIAN_POINT('Ctrl Pts',(70.4779346423502,213.258471670562,30.2513203435596)) ;
#76358=CARTESIAN_POINT('Ctrl Pts',(83.5725617978318,190.143531583735,30.2513203435596)) ;
#76359=CARTESIAN_POINT('Ctrl Pts',(82.0318758172802,191.680398780727,30.2513203435596)) ;
#76360=CARTESIAN_POINT('Ctrl Pts',(78.5794475585013,195.403251084408,30.2513203435596)) ;
#76361=CARTESIAN_POINT('Ctrl Pts',(75.589441862932,199.527943855939,30.2513203435596)) ;
#76362=CARTESIAN_POINT('Ctrl Pts',(74.1761041106884,202.05583548982,30.2513203435596)) ;
#76363=CARTESIAN_POINT('Ctrl Pts',(83.5725617978318,190.143531583735,30.2872242596007)) ;
#76364=CARTESIAN_POINT('Ctrl Pts',(82.0318829700591,191.680391645677,30.2872242596007)) ;
#76365=CARTESIAN_POINT('Ctrl Pts',(78.5794502186911,195.403252953423,30.2872242596007)) ;
#76366=CARTESIAN_POINT('Ctrl Pts',(75.5894268919727,199.527970632951,30.2872242596007)) ;
#76367=CARTESIAN_POINT('Ctrl Pts',(74.1761041106884,202.05583548982,30.2872242596007)) ;
#76368=CARTESIAN_POINT('Ctrl Pts',(83.5512629812335,190.12217984417,30.3493567154327)) ;
#76369=CARTESIAN_POINT('Ctrl Pts',(82.0100128578202,191.659609785726,30.3493567154327)) ;
#76370=CARTESIAN_POINT('Ctrl Pts',(78.5561937473121,195.383949481323,30.3493567154327)) ;
#76371=CARTESIAN_POINT('Ctrl Pts',(75.5642990161483,199.511114476272,30.3493567154327)) ;
#76372=CARTESIAN_POINT('Ctrl Pts',(74.1497804976783,202.041118025058,30.3493567154327)) ;
#76373=CARTESIAN_POINT('Ctrl Pts',(83.506831624286,190.077638084883,30.3713203435596)) ;
#76374=CARTESIAN_POINT('Ctrl Pts',(81.9644087053098,191.61623791508,30.3713203435596)) ;
#76375=CARTESIAN_POINT('Ctrl Pts',(78.5076855957178,195.3436855626,30.3713203435596)) ;
#76376=CARTESIAN_POINT('Ctrl Pts',(75.5118401487742,199.476021989111,30.3713203435596)) ;
#76377=CARTESIAN_POINT('Ctrl Pts',(74.0948669375562,202.010415993931,30.3713203435596)) ;
#76378=CARTESIAN_POINT('Ctrl Pts',(83.4878143389934,190.058573545737,30.3713203435596)) ;
#76379=CARTESIAN_POINT('Ctrl Pts',(81.9448902074828,191.59767334615,30.3713203435596)) ;
#76380=CARTESIAN_POINT('Ctrl Pts',(78.4869236645555,195.326452202177,30.3713203435596)) ;
#76381=CARTESIAN_POINT('Ctrl Pts',(75.4893853751038,199.461004730524,30.3713203435596)) ;
#76382=CARTESIAN_POINT('Ctrl Pts',(74.071363112532,201.997275065426,30.3713203435596)) ;
#76383=CARTESIAN_POINT('',(83.5725617978318,190.143531583735,30.2513203435596)) ;
#76384=CARTESIAN_POINT('Origin',(83.4878143389934,190.058573545737,30.2513203435596)) ;
#76385=CARTESIAN_POINT('Ctrl Pts',(83.5725617978318,190.143531583735,30.2513203435596)) ;
#76386=CARTESIAN_POINT('Ctrl Pts',(83.16020700552,190.554864302944,30.2513203435596)) ;
#76387=CARTESIAN_POINT('Ctrl Pts',(82.1803361041118,191.549821741792,30.2513203435596)) ;
#76388=CARTESIAN_POINT('Ctrl Pts',(80.6886895533707,193.132887074724,30.2513203435596)) ;
#76389=CARTESIAN_POINT('Ctrl Pts',(78.784019206408,195.312002858836,30.2513203435596)) ;
#76390=CARTESIAN_POINT('Ctrl Pts',(76.933494947875,197.696777376424,30.2513203435596)) ;
#76391=CARTESIAN_POINT('Ctrl Pts',(75.5850166034805,199.677432982293,30.2513203435596)) ;
#76392=CARTESIAN_POINT('Ctrl Pts',(74.7358054436199,201.068974645156,30.2513203435596)) ;
#76393=CARTESIAN_POINT('Ctrl Pts',(74.2838092722993,201.863194363147,30.2513203435596)) ;
#76394=CARTESIAN_POINT('Ctrl Pts',(74.1761041106884,202.05583548982,30.2513203435596)) ;
#76395=CARTESIAN_POINT('Ctrl Pts',(83.4878143389935,190.058573545737,30.3713203435596)) ;
#76396=CARTESIAN_POINT('Ctrl Pts',(83.5482147548369,189.998322839904,30.3713203435596)) ;
#76397=CARTESIAN_POINT('Ctrl Pts',(83.6266011938506,189.835494820776,30.3713203435596)) ;
#76398=CARTESIAN_POINT('Ctrl Pts',(83.576428513561,189.615885650627,30.3713203435596)) ;
#76399=CARTESIAN_POINT('Ctrl Pts',(83.4319195690048,189.454561122737,30.3713203435596)) ;
#76400=CARTESIAN_POINT('Ctrl Pts',(83.3047606779792,189.409539758744,30.3713203435596)) ;
#76401=CARTESIAN_POINT('Ctrl Pts',(83.2194473860052,189.409539758744,30.3713203435596)) ;
#76402=CARTESIAN_POINT('Ctrl Pts',(83.5131707193837,190.083992931264,30.3713203435596)) ;
#76403=CARTESIAN_POINT('Ctrl Pts',(83.5793027341282,190.018024833018,30.3713203435596)) ;
#76404=CARTESIAN_POINT('Ctrl Pts',(83.6651610120024,189.839826806225,30.3713203435596)) ;
#76405=CARTESIAN_POINT('Ctrl Pts',(83.6102436634627,189.599417715804,30.3713203435596)) ;
#76406=CARTESIAN_POINT('Ctrl Pts',(83.4520401256346,189.422828986583,30.3713203435596)) ;
#76407=CARTESIAN_POINT('Ctrl Pts',(83.3128563436082,189.373635842703,30.3713203435596)) ;
#76408=CARTESIAN_POINT('Ctrl Pts',(83.2194473860052,189.373635842703,30.3713203435596)) ;
#76409=CARTESIAN_POINT('Ctrl Pts',(83.5570504774321,190.127981721049,30.3411618545504)) ;
#76410=CARTESIAN_POINT('Ctrl Pts',(83.6330276918247,190.052192825717,30.3411618545504)) ;
#76411=CARTESIAN_POINT('Ctrl Pts',(83.7316213436252,189.847353201833,30.3411618545504)) ;
#76412=CARTESIAN_POINT('Ctrl Pts',(83.6685055832356,189.571099036852,30.3411618545504)) ;
#76413=CARTESIAN_POINT('Ctrl Pts',(83.4867244971632,189.368159496056,30.3411618545504)) ;
#76414=CARTESIAN_POINT('Ctrl Pts',(83.3267623139628,189.311503348844,30.3411618545504)) ;
#76415=CARTESIAN_POINT('Ctrl Pts',(83.2194473860052,189.311503348844,30.3411618545504)) ;
#76416=CARTESIAN_POINT('Ctrl Pts',(83.5725617978319,190.143531583735,30.2782482805904)) ;
#76417=CARTESIAN_POINT('Ctrl Pts',(83.6520515313441,190.064238875503,30.2782482805904)) ;
#76418=CARTESIAN_POINT('Ctrl Pts',(83.7552326945549,189.850000656062,30.2782482805904)) ;
#76419=CARTESIAN_POINT('Ctrl Pts',(83.6892134061226,189.561009642818,30.2782482805904)) ;
#76420=CARTESIAN_POINT('Ctrl Pts',(83.4990444715275,189.348726975021,30.2782482805904)) ;
#76421=CARTESIAN_POINT('Ctrl Pts',(83.3317236137325,189.289539758744,30.2782482805904)) ;
#76422=CARTESIAN_POINT('Ctrl Pts',(83.2194473860052,189.289539758744,30.2782482805904)) ;
#76423=CARTESIAN_POINT('Ctrl Pts',(83.5725617978319,190.143531583735,30.2513203435596)) ;
#76424=CARTESIAN_POINT('Ctrl Pts',(83.6520360292049,190.064254339218,30.2513203435596)) ;
#76425=CARTESIAN_POINT('Ctrl Pts',(83.7551760805387,189.850006945628,30.2513203435596)) ;
#76426=CARTESIAN_POINT('Ctrl Pts',(83.6891593959471,189.561047511221,30.2513203435596)) ;
#76427=CARTESIAN_POINT('Ctrl Pts',(83.4990160478468,189.348778395577,30.2513203435596)) ;
#76428=CARTESIAN_POINT('Ctrl Pts',(83.3317017175499,189.289539758744,30.2513203435596)) ;
#76429=CARTESIAN_POINT('Ctrl Pts',(83.2194473860052,189.289539758744,30.2513203435596)) ;
#76430=CARTESIAN_POINT('',(83.2194473860052,189.289539758744,30.2513203435596)) ;
#76431=CARTESIAN_POINT('Origin',(83.2194473860052,189.409539758744,30.2513203435596)) ;
#76432=CARTESIAN_POINT('Ctrl Pts',(83.2194473860051,189.289539758744,30.2513203435596)) ;
#76433=CARTESIAN_POINT('Ctrl Pts',(83.2755767988648,189.289539758744,30.2513203435596)) ;
#76434=CARTESIAN_POINT('Ctrl Pts',(83.4441273250624,189.317541444415,30.2513203435596)) ;
#76435=CARTESIAN_POINT('Ctrl Pts',(83.6762811453293,189.502581007553,30.2513203435596)) ;
#76436=CARTESIAN_POINT('Ctrl Pts',(83.7551748851088,189.850164868248,30.2513203435596)) ;
#76437=CARTESIAN_POINT('Ctrl Pts',(83.6520392110072,190.064251165302,30.2513203435596)) ;
#76438=CARTESIAN_POINT('Ctrl Pts',(83.5725617978318,190.143531583735,30.2513203435596)) ;
#76439=CARTESIAN_POINT('Origin',(73.5558661461117,189.409539758744,30.2513203435596)) ;
#76440=CARTESIAN_POINT('',(77.8285014478222,189.289539758744,30.2513203435596)) ;
#76441=CARTESIAN_POINT('Origin',(77.8285014478222,189.409539758744,30.2513203435596)) ;
#76442=CARTESIAN_POINT('',(73.5558661461117,189.289539758744,30.2513203435596)) ;
#76443=CARTESIAN_POINT('Ctrl Pts',(77.8285014478222,189.409539758744,30.3713203435596)) ;
#76444=CARTESIAN_POINT('Ctrl Pts',(77.6025348183859,189.409539758744,30.3713203435596)) ;
#76445=CARTESIAN_POINT('Ctrl Pts',(77.3771291752411,189.482701147464,30.3713203435596)) ;
#76446=CARTESIAN_POINT('Ctrl Pts',(77.1942359127804,189.615407485539,30.3713203435596)) ;
#76447=CARTESIAN_POINT('Ctrl Pts',(77.8285014478222,189.373635842703,30.3713203435596)) ;
#76448=CARTESIAN_POINT('Ctrl Pts',(77.5949901525181,189.373635842703,30.3713203435596)) ;
#76449=CARTESIAN_POINT('Ctrl Pts',(77.3621499339521,189.449210320354,30.3713203435596)) ;
#76450=CARTESIAN_POINT('Ctrl Pts',(77.1731501567454,189.5863475117,30.3713203435596)) ;
#76451=CARTESIAN_POINT('Ctrl Pts',(77.8285014478222,189.311503249434,30.3411619374018)) ;
#76452=CARTESIAN_POINT('Ctrl Pts',(77.5820306375502,189.311503249434,30.3411619374018)) ;
#76453=CARTESIAN_POINT('Ctrl Pts',(77.3361497189201,189.391310432679,30.3411619374018)) ;
#76454=CARTESIAN_POINT('Ctrl Pts',(77.1366607470111,189.536058525595,30.3411619374018)) ;
#76455=CARTESIAN_POINT('Ctrl Pts',(77.8285014478222,189.289539758744,30.2782482805904)) ;
#76456=CARTESIAN_POINT('Ctrl Pts',(77.5774070092103,189.289539758744,30.2782482805904)) ;
#76457=CARTESIAN_POINT('Ctrl Pts',(77.3269932166768,189.370818206616,30.2782482805904)) ;
#76458=CARTESIAN_POINT('Ctrl Pts',(77.1237619644425,189.518281677405,30.2782482805904)) ;
#76459=CARTESIAN_POINT('Ctrl Pts',(77.8285014478222,189.289539758744,30.2513203435596)) ;
#76460=CARTESIAN_POINT('Ctrl Pts',(77.577427415115,189.289539758744,30.2513203435596)) ;
#76461=CARTESIAN_POINT('Ctrl Pts',(77.3269767005102,189.370830190655,30.2513203435596)) ;
#76462=CARTESIAN_POINT('Ctrl Pts',(77.1237619644425,189.518281677405,30.2513203435596)) ;
#76463=CARTESIAN_POINT('',(77.1237619644425,189.518281677405,30.2513203435596)) ;
#76464=CARTESIAN_POINT('Origin',(77.1942359127804,189.615407485539,30.2513203435596)) ;
#76465=CARTESIAN_POINT('Origin',(77.736831196317,190.207109471954,30.2513203435596)) ;
#76466=CARTESIAN_POINT('Ctrl Pts',(66.1952689412979,200.55583548982,30.2513203435596)) ;
#76467=CARTESIAN_POINT('Ctrl Pts',(67.4193871398855,198.688317658303,30.2513203435596)) ;
#76468=CARTESIAN_POINT('Ctrl Pts',(70.723607560073,194.63303708426,30.2513203435596)) ;
#76469=CARTESIAN_POINT('Ctrl Pts',(74.7177688589066,191.264056946398,30.2513203435596)) ;
#76470=CARTESIAN_POINT('Ctrl Pts',(77.1237619644425,189.518281677405,30.2513203435596)) ;
#76471=CARTESIAN_POINT('Ctrl Pts',(66.1952689412979,200.55583548982,30.2872242596007)) ;
#76472=CARTESIAN_POINT('Ctrl Pts',(67.4194012221606,198.688296174348,30.2872242596007)) ;
#76473=CARTESIAN_POINT('Ctrl Pts',(70.7236224085444,194.63301168528,30.2872242596007)) ;
#76474=CARTESIAN_POINT('Ctrl Pts',(74.7177531457742,191.26406834776,30.2872242596007)) ;
#76475=CARTESIAN_POINT('Ctrl Pts',(77.1237619644425,189.518281677405,30.2872242596007)) ;
#76476=CARTESIAN_POINT('Ctrl Pts',(66.2204917300716,200.572368491131,30.3493568579639)) ;
#76477=CARTESIAN_POINT('Ctrl Pts',(67.4434992533509,198.706545108684,30.3493568579639)) ;
#76478=CARTESIAN_POINT('Ctrl Pts',(70.7448735388302,194.654676064875,30.3493568579639)) ;
#76479=CARTESIAN_POINT('Ctrl Pts',(74.7367196744804,191.287567375558,30.3493568579639)) ;
#76480=CARTESIAN_POINT('Ctrl Pts',(77.1414734782616,189.542691337053,30.3493568579639)) ;
#76481=CARTESIAN_POINT('Ctrl Pts',(66.2731091727487,200.60685810513,30.3713203435596)) ;
#76482=CARTESIAN_POINT('Ctrl Pts',(67.4938077151616,198.744557309755,30.3713203435596)) ;
#76483=CARTESIAN_POINT('Ctrl Pts',(70.7892450940213,194.699802857899,30.3713203435596)) ;
#76484=CARTESIAN_POINT('Ctrl Pts',(74.7762441741238,191.336619135049,30.3713203435596)) ;
#76485=CARTESIAN_POINT('Ctrl Pts',(77.1784215957542,189.59361250516,30.3713203435596)) ;
#76486=CARTESIAN_POINT('Ctrl Pts',(66.2956301826426,200.621620147878,30.3713203435596)) ;
#76487=CARTESIAN_POINT('Ctrl Pts',(67.5153419459542,198.760824785205,30.3713203435596)) ;
#76488=CARTESIAN_POINT('Ctrl Pts',(70.8082383262559,194.719115063076,30.3713203435596)) ;
#76489=CARTESIAN_POINT('Ctrl Pts',(74.7931595483741,191.357615194406,30.3713203435596)) ;
#76490=CARTESIAN_POINT('Ctrl Pts',(77.1942359127805,189.615407485539,30.3713203435596)) ;
#76491=CARTESIAN_POINT('',(66.1952689412922,200.555835489829,30.2513203435596)) ;
#76492=CARTESIAN_POINT('Origin',(66.2956301826426,200.621620147878,30.2513203435596)) ;
#76493=CARTESIAN_POINT('Ctrl Pts',(66.1952689412979,200.55583548982,30.2513203435596)) ;
#76494=CARTESIAN_POINT('Ctrl Pts',(66.518831227978,200.062208043811,30.2513203435596)) ;
#76495=CARTESIAN_POINT('Ctrl Pts',(67.2058910887118,199.062896363505,30.2513203435596)) ;
#76496=CARTESIAN_POINT('Ctrl Pts',(68.3175691899266,197.591996864875,30.2513203435596)) ;
#76497=CARTESIAN_POINT('Ctrl Pts',(69.9484449125888,195.702271045863,30.2513203435596)) ;
#76498=CARTESIAN_POINT('Ctrl Pts',(72.1605421210852,193.509486853481,30.2513203435596)) ;
#76499=CARTESIAN_POINT('Ctrl Pts',(74.0936919389024,191.835218710936,30.2513203435596)) ;
#76500=CARTESIAN_POINT('Ctrl Pts',(75.6101591471701,190.636965311174,30.2513203435596)) ;
#76501=CARTESIAN_POINT('Ctrl Pts',(76.6350044216196,189.872921442927,30.2513203435596)) ;
#76502=CARTESIAN_POINT('Ctrl Pts',(77.1237619644427,189.518281677405,30.2513203435596)) ;
#76503=CARTESIAN_POINT('Ctrl Pts',(65.2679705316394,202.05583548982,30.2513203435596)) ;
#76504=CARTESIAN_POINT('Ctrl Pts',(65.5637332147712,201.547759052751,30.2513203435596)) ;
#76505=CARTESIAN_POINT('Ctrl Pts',(65.8729833388595,201.047515223108,30.2513203435596)) ;
#76506=CARTESIAN_POINT('Ctrl Pts',(66.1952689412975,200.555835489821,30.2513203435596)) ;
#76507=CARTESIAN_POINT('Ctrl Pts',(65.2679705316394,202.05583548982,30.2872242596007)) ;
#76508=CARTESIAN_POINT('Ctrl Pts',(65.5637366175854,201.547753207221,30.2872242596007)) ;
#76509=CARTESIAN_POINT('Ctrl Pts',(65.8729796312809,201.0475208794,30.2872242596007)) ;
#76510=CARTESIAN_POINT('Ctrl Pts',(66.1952689412975,200.555835489821,30.2872242596007)) ;
#76511=CARTESIAN_POINT('Ctrl Pts',(65.2940344552751,202.071007884021,30.3493568489088)) ;
#76512=CARTESIAN_POINT('Ctrl Pts',(65.589528756939,201.563392486522,30.3493568489088)) ;
#76513=CARTESIAN_POINT('Ctrl Pts',(65.8984985523252,201.063602114333,30.3493568489088)) ;
#76514=CARTESIAN_POINT('Ctrl Pts',(66.2204917363829,200.572368495269,30.3493568489088)) ;
#76515=CARTESIAN_POINT('Ctrl Pts',(65.3484065753628,202.102659113937,30.3713203435596)) ;
#76516=CARTESIAN_POINT('Ctrl Pts',(65.6433429392841,201.596002170755,30.3713203435596)) ;
#76517=CARTESIAN_POINT('Ctrl Pts',(65.9517238967263,201.097164298152,30.3713203435596)) ;
#76518=CARTESIAN_POINT('Ctrl Pts',(66.2731091727483,200.60685810513,30.3713203435596)) ;
#76519=CARTESIAN_POINT('Ctrl Pts',(65.371678614805,202.116206289766,30.3713203435596)) ;
#76520=CARTESIAN_POINT('Ctrl Pts',(65.6663765353021,201.609958957032,30.3713203435596)) ;
#76521=CARTESIAN_POINT('Ctrl Pts',(65.9745047056309,201.11152999087,30.3713203435596)) ;
#76522=CARTESIAN_POINT('Ctrl Pts',(66.2956301826422,200.621620147878,30.3713203435596)) ;
#76523=CARTESIAN_POINT('',(65.2679705316444,202.055835489811,30.2513203435596)) ;
#76524=CARTESIAN_POINT('Origin',(65.371678614805,202.116206289766,30.2513203435596)) ;
#76525=CARTESIAN_POINT('Origin',(94.0039513890618,218.783760942349,30.2513203435596)) ;
#76526=CARTESIAN_POINT('Ctrl Pts',(61.1448474062769,212.657605881106,30.2513203435596)) ;
#76527=CARTESIAN_POINT('Ctrl Pts',(62.0239099776425,208.957224782185,30.2513203435596)) ;
#76528=CARTESIAN_POINT('Ctrl Pts',(63.3524709375853,205.346379782453,30.2513203435596)) ;
#76529=CARTESIAN_POINT('Ctrl Pts',(65.2679705316376,202.055835489823,30.2513203435596)) ;
#76530=CARTESIAN_POINT('Ctrl Pts',(61.1448474062769,212.657605881106,30.2872242596007)) ;
#76531=CARTESIAN_POINT('Ctrl Pts',(62.0239170695688,208.957194928986,30.2872242596007)) ;
#76532=CARTESIAN_POINT('Ctrl Pts',(63.3524488993448,205.346417640882,30.2872242596007)) ;
#76533=CARTESIAN_POINT('Ctrl Pts',(65.2679705316376,202.055835489823,30.2872242596007)) ;
#76534=CARTESIAN_POINT('Ctrl Pts',(61.1741893104987,212.66457634417,30.3493567486976)) ;
#76535=CARTESIAN_POINT('Ctrl Pts',(62.0526925384775,208.966549780369,30.3493567486976)) ;
#76536=CARTESIAN_POINT('Ctrl Pts',(63.3802730992418,205.358566307474,30.3493567486976)) ;
#76537=CARTESIAN_POINT('Ctrl Pts',(65.2940345274534,202.071007926042,30.3493567486976)) ;
#76538=CARTESIAN_POINT('Ctrl Pts',(61.2353993963707,212.67911741279,30.3713203435596)) ;
#76539=CARTESIAN_POINT('Ctrl Pts',(62.1127398064059,208.985985687741,30.3713203435596)) ;
#76540=CARTESIAN_POINT('Ctrl Pts',(63.4382586169361,205.384010090046,30.3713203435596)) ;
#76541=CARTESIAN_POINT('Ctrl Pts',(65.3484065753611,202.10265911394,30.3713203435596)) ;
#76542=CARTESIAN_POINT('Ctrl Pts',(61.2615982170421,212.685341204894,30.3713203435596)) ;
#76543=CARTESIAN_POINT('Ctrl Pts',(62.1384416786349,208.994301365774,30.3713203435596)) ;
#76544=CARTESIAN_POINT('Ctrl Pts',(63.4630749292305,205.394904434083,30.3713203435596)) ;
#76545=CARTESIAN_POINT('Ctrl Pts',(65.3716786148033,202.116206289769,30.3713203435596)) ;
#76546=CARTESIAN_POINT('',(61.1448474062699,212.657605881124,30.2513203435596)) ;
#76547=CARTESIAN_POINT('Origin',(61.2615982170421,212.685341204894,30.2513203435596)) ;
#76548=CARTESIAN_POINT('Origin',(136.041288291393,279.717177048122,30.2513203435596)) ;
#76549=CARTESIAN_POINT('Ctrl Pts',(60.8054892120567,214.197609441503,30.2513203435596)) ;
#76550=CARTESIAN_POINT('Ctrl Pts',(60.9103243659135,213.682523068924,30.2513203435596)) ;
#76551=CARTESIAN_POINT('Ctrl Pts',(61.0233429894376,213.16907419082,30.2513203435596)) ;
#76552=CARTESIAN_POINT('Ctrl Pts',(61.1448474062677,212.657605881144,30.2513203435596)) ;
#76553=CARTESIAN_POINT('Ctrl Pts',(60.8054892120567,214.197609441503,30.2872242596007)) ;
#76554=CARTESIAN_POINT('Ctrl Pts',(60.9103251761397,213.682519088041,30.2872242596007)) ;
#76555=CARTESIAN_POINT('Ctrl Pts',(61.0233420091884,213.169078317142,30.2872242596007)) ;
#76556=CARTESIAN_POINT('Ctrl Pts',(61.1448474062677,212.657605881144,30.2872242596007)) ;
#76557=CARTESIAN_POINT('Ctrl Pts',(60.835041834708,214.203624265245,30.3493567305651)) ;
#76558=CARTESIAN_POINT('Ctrl Pts',(60.9398130856633,213.688851866676,30.3493567305651)) ;
#76559=CARTESIAN_POINT('Ctrl Pts',(61.0527622210523,213.175719212493,30.3493567305651)) ;
#76560=CARTESIAN_POINT('Ctrl Pts',(61.1741893251925,212.664576347702,30.3493567305651)) ;
#76561=CARTESIAN_POINT('Ctrl Pts',(60.8966914541607,214.216171767342,30.3713203435596)) ;
#76562=CARTESIAN_POINT('Ctrl Pts',(61.0013298574909,213.702052088771,30.3713203435596)) ;
#76563=CARTESIAN_POINT('Ctrl Pts',(61.114133017431,213.189583710846,30.3713203435596)) ;
#76564=CARTESIAN_POINT('Ctrl Pts',(61.2353993963615,212.679117412829,30.3713203435596)) ;
#76565=CARTESIAN_POINT('Ctrl Pts',(60.9230784080337,214.221542284825,30.3713203435596)) ;
#76566=CARTESIAN_POINT('Ctrl Pts',(61.0276600368527,213.707701556357,30.3713203435596)) ;
#76567=CARTESIAN_POINT('Ctrl Pts',(61.1404005265357,213.195518361553,30.3713203435596)) ;
#76568=CARTESIAN_POINT('Ctrl Pts',(61.261598217033,212.685341204933,30.3713203435596)) ;
#76569=CARTESIAN_POINT('',(60.8054892120567,214.197609441503,30.2513203435596)) ;
#76570=CARTESIAN_POINT('Origin',(60.9230784080337,214.221542284825,30.2513203435596)) ;
#76571=CARTESIAN_POINT('Origin',(195.552488558874,312.073624274513,30.2513203435596)) ;
#76572=CARTESIAN_POINT('Ctrl Pts',(60.7651166309946,214.398081303037,30.2513203435596)) ;
#76573=CARTESIAN_POINT('Ctrl Pts',(60.7784368168398,214.3312301992,30.2513203435596)) ;
#76574=CARTESIAN_POINT('Ctrl Pts',(60.7918941539075,214.264406016215,30.2513203435596)) ;
#76575=CARTESIAN_POINT('Ctrl Pts',(60.8054892120567,214.197609441503,30.2513203435596)) ;
#76576=CARTESIAN_POINT('Ctrl Pts',(60.7651166309946,214.398081303037,30.2872242596007)) ;
#76577=CARTESIAN_POINT('Ctrl Pts',(60.7784369192806,214.331229685072,30.2872242596007)) ;
#76578=CARTESIAN_POINT('Ctrl Pts',(60.7918940488371,214.264406532458,30.2872242596007)) ;
#76579=CARTESIAN_POINT('Ctrl Pts',(60.8054892120567,214.197609441503,30.2872242596007)) ;
#76580=CARTESIAN_POINT('Ctrl Pts',(60.7946937326725,214.403974586296,30.3493567281575)) ;
#76581=CARTESIAN_POINT('Ctrl Pts',(60.8080058389667,214.337164031961,30.3493567281575)) ;
#76582=CARTESIAN_POINT('Ctrl Pts',(60.821455065475,214.270380124101,30.3493567281575)) ;
#76583=CARTESIAN_POINT('Ctrl Pts',(60.8350418366743,214.203624265645,30.3493567281575)) ;
#76584=CARTESIAN_POINT('Ctrl Pts',(60.856394411661,214.416268542024,30.3713203435596)) ;
#76585=CARTESIAN_POINT('Ctrl Pts',(60.8696897213913,214.349542285975,30.3713203435596)) ;
#76586=CARTESIAN_POINT('Ctrl Pts',(60.8831219106862,214.282842980849,30.3713203435596)) ;
#76587=CARTESIAN_POINT('Ctrl Pts',(60.8966914541607,214.216171767342,30.3713203435596)) ;
#76588=CARTESIAN_POINT('Ctrl Pts',(60.882803220617,214.421530538057,30.3713203435596)) ;
#76589=CARTESIAN_POINT('Ctrl Pts',(60.8960913520729,214.3548403082,30.3713203435596)) ;
#76590=CARTESIAN_POINT('Ctrl Pts',(60.9095162270971,214.288177323988,30.3713203435596)) ;
#76591=CARTESIAN_POINT('Ctrl Pts',(60.9230784080337,214.221542284825,30.3713203435596)) ;
#76592=CARTESIAN_POINT('',(60.7651166309946,214.398081303037,30.2513203435596)) ;
#76593=CARTESIAN_POINT('Origin',(60.882803220617,214.421530538057,30.2513203435596)) ;
#76594=CARTESIAN_POINT('Origin',(151.214887771711,273.326691475263,30.2513203435596)) ;
#76595=CARTESIAN_POINT('Ctrl Pts',(60.882803220617,214.421530538057,30.3713203435596)) ;
#76596=CARTESIAN_POINT('Ctrl Pts',(60.7690431212421,214.992467633397,30.3713203435596)) ;
#76597=CARTESIAN_POINT('Ctrl Pts',(60.7116108526749,215.57461370503,30.3713203435596)) ;
#76598=CARTESIAN_POINT('Ctrl Pts',(60.7116108526749,216.156773929576,30.3713203435596)) ;
#76599=CARTESIAN_POINT('Ctrl Pts',(60.8475914753424,214.414514543346,30.3713203435596)) ;
#76600=CARTESIAN_POINT('Ctrl Pts',(60.7333694243887,214.987770072776,30.3713203435596)) ;
#76601=CARTESIAN_POINT('Ctrl Pts',(60.6757069366339,215.572249696592,30.3713203435596)) ;
#76602=CARTESIAN_POINT('Ctrl Pts',(60.6757069366339,216.156773929576,30.3713203435596)) ;
#76603=CARTESIAN_POINT('Ctrl Pts',(60.7866568455963,214.402373224115,30.3411618139191)) ;
#76604=CARTESIAN_POINT('Ctrl Pts',(60.6716412978193,214.979611140814,30.3411618139191)) ;
#76605=CARTESIAN_POINT('Ctrl Pts',(60.613574491527,215.568189026011,30.3411618139191)) ;
#76606=CARTESIAN_POINT('Ctrl Pts',(60.613574491527,216.156773929576,30.3411618139191)) ;
#76607=CARTESIAN_POINT('Ctrl Pts',(60.7651166309946,214.398081303037,30.2782482805904)) ;
#76608=CARTESIAN_POINT('Ctrl Pts',(60.6498179835484,214.976740035151,30.2782482805904)) ;
#76609=CARTESIAN_POINT('Ctrl Pts',(60.5916108526749,215.566740281083,30.2782482805904)) ;
#76610=CARTESIAN_POINT('Ctrl Pts',(60.5916108526749,216.156773929576,30.2782482805904)) ;
#76611=CARTESIAN_POINT('Ctrl Pts',(60.7651166309946,214.398081303037,30.2513203435596)) ;
#76612=CARTESIAN_POINT('Ctrl Pts',(60.6498192329795,214.976733764529,30.2513203435596)) ;
#76613=CARTESIAN_POINT('Ctrl Pts',(60.5916108526749,215.566746674968,30.2513203435596)) ;
#76614=CARTESIAN_POINT('Ctrl Pts',(60.5916108526749,216.156773929576,30.2513203435596)) ;
#76615=CARTESIAN_POINT('',(60.5916108526749,216.156773929576,30.2513203435596)) ;
#76616=CARTESIAN_POINT('Origin',(60.7116108526749,216.156773929576,30.2513203435596)) ;
#76617=CARTESIAN_POINT('Origin',(69.5988372871804,216.157486861515,30.2513203435596)) ;
#76618=CARTESIAN_POINT('Origin',(60.7116108526749,218.583329440748,30.2513203435596)) ;
#76619=CARTESIAN_POINT('',(60.5916108526749,219.547374675056,30.2513203435596)) ;
#76620=CARTESIAN_POINT('',(60.5916108526749,218.583329440748,30.2513203435596)) ;
#76621=CARTESIAN_POINT('Origin',(60.7116108526749,219.512965228765,30.2513203435596)) ;
#76622=CARTESIAN_POINT('Origin',(61.5409585020332,220.840198908612,30.2513203435596)) ;
#76623=CARTESIAN_POINT('',(60.6037668263229,219.566828299419,30.2513203435596)) ;
#76624=CARTESIAN_POINT('',(61.4391927304944,220.90378922032,30.2513203435596)) ;
#76625=CARTESIAN_POINT('Ctrl Pts',(60.7297059832955,219.541923491104,30.3713203435596)) ;
#76626=CARTESIAN_POINT('Ctrl Pts',(60.7291626690358,219.542029099686,30.3713203435596)) ;
#76627=CARTESIAN_POINT('Ctrl Pts',(60.7286193620522,219.542134730958,30.3713170060568)) ;
#76628=CARTESIAN_POINT('Ctrl Pts',(60.7280760963346,219.54224037829,30.3713103308243)) ;
#76629=CARTESIAN_POINT('Ctrl Pts',(60.7189335421281,219.544018304694,30.3711979941303)) ;
#76630=CARTESIAN_POINT('Ctrl Pts',(60.7098171452966,219.545798043439,30.3701405530434)) ;
#76631=CARTESIAN_POINT('Ctrl Pts',(60.7008889231376,219.54754742674,30.368145968699)) ;
#76632=CARTESIAN_POINT('Ctrl Pts',(60.6920179977229,219.549285583397,30.3661641845724)) ;
#76633=CARTESIAN_POINT('Ctrl Pts',(60.683361871084,219.550988074979,30.3632636735234)) ;
#76634=CARTESIAN_POINT('Ctrl Pts',(60.6750811551749,219.552622038395,30.3594713481367)) ;
#76635=CARTESIAN_POINT('Ctrl Pts',(60.6641759608159,219.554773867877,30.3544770884776)) ;
#76636=CARTESIAN_POINT('Ctrl Pts',(60.6540116015145,219.556788120498,30.3479775495335)) ;
#76637=CARTESIAN_POINT('Ctrl Pts',(60.644940406564,219.558593136451,30.3401148642541)) ;
#76638=CARTESIAN_POINT('Ctrl Pts',(60.6419212766097,219.559193892775,30.3374979577961)) ;
#76639=CARTESIAN_POINT('Ctrl Pts',(60.6390235198649,219.559771296374,30.3347301949426)) ;
#76640=CARTESIAN_POINT('Ctrl Pts',(60.6362611894693,219.560322040799,30.3318176370222)) ;
#76641=CARTESIAN_POINT('Ctrl Pts',(60.6280519358831,219.561958775005,30.3231619285703)) ;
#76642=CARTESIAN_POINT('Ctrl Pts',(60.6211548413867,219.563338504298,30.313349088554)) ;
#76643=CARTESIAN_POINT('Ctrl Pts',(60.6158491185412,219.564402430005,30.3026493500833)) ;
#76644=CARTESIAN_POINT('Ctrl Pts',(60.6144636513314,219.564680249677,30.2998553600397)) ;
#76645=CARTESIAN_POINT('Ctrl Pts',(60.6131868361209,219.564936447647,30.2970010850957)) ;
#76646=CARTESIAN_POINT('Ctrl Pts',(60.6120239762211,219.565169769653,30.294091919136)) ;
#76647=CARTESIAN_POINT('Ctrl Pts',(60.6065879367601,219.566260483705,30.2804923952736)) ;
#76648=CARTESIAN_POINT('Ctrl Pts',(60.6037668263229,219.566828299419,30.2660017542171)) ;
#76649=CARTESIAN_POINT('Ctrl Pts',(60.6037668263229,219.566828299419,30.2513203435596)) ;
#76650=CARTESIAN_POINT('Origin',(64.1568347953872,220.146231446812,30.2513203435596)) ;
#76651=CARTESIAN_POINT('Origin',(64.1568347953872,220.146231446812,30.2513203435596)) ;
#76652=CARTESIAN_POINT('Ctrl Pts',(66.1952689412979,200.55583548982,17.8713203435596)) ;
#76653=CARTESIAN_POINT('Ctrl Pts',(66.1952689412979,200.55583548982,32.8713203435596)) ;
#76654=CARTESIAN_POINT('Ctrl Pts',(66.518831227978,200.062208043811,17.8713203435596)) ;
#76655=CARTESIAN_POINT('Ctrl Pts',(66.518831227978,200.062208043811,32.8713203435596)) ;
#76656=CARTESIAN_POINT('Ctrl Pts',(67.2058910887118,199.062896363505,17.8713203435596)) ;
#76657=CARTESIAN_POINT('Ctrl Pts',(67.2058910887118,199.062896363505,32.8713203435596)) ;
#76658=CARTESIAN_POINT('Ctrl Pts',(68.3175691899266,197.591996864875,17.8713203435596)) ;
#76659=CARTESIAN_POINT('Ctrl Pts',(68.3175691899266,197.591996864875,32.8713203435596)) ;
#76660=CARTESIAN_POINT('Ctrl Pts',(69.9484449125888,195.702271045863,17.8713203435596)) ;
#76661=CARTESIAN_POINT('Ctrl Pts',(69.9484449125888,195.702271045863,32.8713203435596)) ;
#76662=CARTESIAN_POINT('Ctrl Pts',(72.2129379945247,193.457548429354,17.8713203435596)) ;
#76663=CARTESIAN_POINT('Ctrl Pts',(72.2129379945247,193.457548429354,32.8713203435596)) ;
#76664=CARTESIAN_POINT('Ctrl Pts',(74.2078323511403,191.736557054229,17.8713203435596)) ;
#76665=CARTESIAN_POINT('Ctrl Pts',(74.2078323511403,191.736557054229,32.8713203435596)) ;
#76666=CARTESIAN_POINT('Ctrl Pts',(75.7911794288343,190.494445187268,17.8713203435596)) ;
#76667=CARTESIAN_POINT('Ctrl Pts',(75.7911794288343,190.494445187268,32.8713203435596)) ;
#76668=CARTESIAN_POINT('Ctrl Pts',(76.884855729364,189.687631312612,17.8713203435596)) ;
#76669=CARTESIAN_POINT('Ctrl Pts',(76.884855729364,189.687631312612,32.8713203435596)) ;
#76670=CARTESIAN_POINT('Ctrl Pts',(77.4412221473412,189.289539758744,17.8713203435596)) ;
#76671=CARTESIAN_POINT('Ctrl Pts',(77.4412221473412,189.289539758744,32.8713203435596)) ;
#76672=CARTESIAN_POINT('',(66.1952689412922,200.555835489829,17.9913203435596)) ;
#76673=CARTESIAN_POINT('',(66.1952689412979,200.55583548982,29.8713203435596)) ;
#76674=CARTESIAN_POINT('',(77.1237619644425,189.518281677405,17.9913203435596)) ;
#76675=CARTESIAN_POINT('Ctrl Pts',(77.1237619644425,189.518281677405,17.9913203435596)) ;
#76676=CARTESIAN_POINT('Ctrl Pts',(75.3192709150292,190.827610386593,17.9913203435596)) ;
#76677=CARTESIAN_POINT('Ctrl Pts',(71.2757417352347,194.115942691271,17.9913203435596)) ;
#76678=CARTESIAN_POINT('Ctrl Pts',(67.8274231206578,198.065816930128,17.9913203435596)) ;
#76679=CARTESIAN_POINT('Ctrl Pts',(66.1952689412979,200.55583548982,17.9913203435596)) ;
#76680=CARTESIAN_POINT('',(77.1237619644425,189.518281677405,30.2513203435596)) ;
#76681=CARTESIAN_POINT('Origin',(93.970367839097,218.762990507114,17.8713203435596)) ;
#76682=CARTESIAN_POINT('',(65.2679705316442,202.055835489812,17.9913203435596)) ;
#76683=CARTESIAN_POINT('',(65.2679705316394,202.05583548982,23.8713203435596)) ;
#76684=CARTESIAN_POINT('Origin',(94.003951389208,218.783760942439,17.9913203435596)) ;
#76685=CARTESIAN_POINT('Ctrl Pts',(61.1448474062769,212.657605881106,17.8713203435596)) ;
#76686=CARTESIAN_POINT('Ctrl Pts',(61.1448474062769,212.657605881106,32.8713203435596)) ;
#76687=CARTESIAN_POINT('Ctrl Pts',(61.1691058108466,212.55549103208,17.8713203435596)) ;
#76688=CARTESIAN_POINT('Ctrl Pts',(61.1691058108466,212.55549103208,32.8713203435596)) ;
#76689=CARTESIAN_POINT('Ctrl Pts',(61.3438459206938,211.828860167372,17.8713203435596)) ;
#76690=CARTESIAN_POINT('Ctrl Pts',(61.3438459206938,211.828860167372,32.8713203435596)) ;
#76691=CARTESIAN_POINT('Ctrl Pts',(61.6936838095791,210.491445465305,17.8713203435596)) ;
#76692=CARTESIAN_POINT('Ctrl Pts',(61.6936838095791,210.491445465305,32.8713203435596)) ;
#76693=CARTESIAN_POINT('Ctrl Pts',(62.2740054220382,208.574144203583,17.8713203435596)) ;
#76694=CARTESIAN_POINT('Ctrl Pts',(62.2740054220382,208.574144203583,32.8713203435596)) ;
#76695=CARTESIAN_POINT('Ctrl Pts',(63.0635008176242,206.4341931397,17.8713203435596)) ;
#76696=CARTESIAN_POINT('Ctrl Pts',(63.0635008176242,206.4341931397,32.8713203435596)) ;
#76697=CARTESIAN_POINT('Ctrl Pts',(63.9562176049502,204.467472055247,17.8713203435596)) ;
#76698=CARTESIAN_POINT('Ctrl Pts',(63.9562176049502,204.467472055247,32.8713203435596)) ;
#76699=CARTESIAN_POINT('Ctrl Pts',(64.6673132018586,203.107895696197,17.8713203435596)) ;
#76700=CARTESIAN_POINT('Ctrl Pts',(64.6673132018586,203.107895696197,32.8713203435596)) ;
#76701=CARTESIAN_POINT('Ctrl Pts',(65.1188571217626,202.311990219034,17.8713203435596)) ;
#76702=CARTESIAN_POINT('Ctrl Pts',(65.1188571217626,202.311990219034,32.8713203435596)) ;
#76703=CARTESIAN_POINT('Ctrl Pts',(65.2679705316376,202.055835489823,17.8713203435596)) ;
#76704=CARTESIAN_POINT('Ctrl Pts',(65.2679705316376,202.055835489823,32.8713203435596)) ;
#76705=CARTESIAN_POINT('',(61.1448474062677,212.657605881144,17.9913203435596)) ;
#76706=CARTESIAN_POINT('',(61.1448474062677,212.657605881144,23.8713203435596)) ;
#76707=CARTESIAN_POINT('Origin',(136.041288291337,279.717177048067,17.9913203435596)) ;
#76708=CARTESIAN_POINT('Ctrl Pts',(60.8054892120567,214.197609441503,17.8713203435596)) ;
#76709=CARTESIAN_POINT('Ctrl Pts',(60.8054892120567,214.197609441503,32.8713203435596)) ;
#76710=CARTESIAN_POINT('Ctrl Pts',(60.8687049964709,213.887011441827,17.8713203435596)) ;
#76711=CARTESIAN_POINT('Ctrl Pts',(60.8687049964709,213.887011441827,32.8713203435596)) ;
#76712=CARTESIAN_POINT('Ctrl Pts',(60.9342401816044,213.577707329413,17.8713203435596)) ;
#76713=CARTESIAN_POINT('Ctrl Pts',(60.9342401816044,213.577707329413,32.8713203435596)) ;
#76714=CARTESIAN_POINT('Ctrl Pts',(61.0021011324506,213.269700654998,17.8713203435596)) ;
#76715=CARTESIAN_POINT('Ctrl Pts',(61.0021011324506,213.269700654998,32.8713203435596)) ;
#76716=CARTESIAN_POINT('Ctrl Pts',(61.0722985912904,212.962997411209,17.8713203435596)) ;
#76717=CARTESIAN_POINT('Ctrl Pts',(61.0722985912904,212.962997411209,32.8713203435596)) ;
#76718=CARTESIAN_POINT('Ctrl Pts',(61.1448474062677,212.657605881144,17.8713203435596)) ;
#76719=CARTESIAN_POINT('Ctrl Pts',(61.1448474062677,212.657605881144,32.8713203435596)) ;
#76720=CARTESIAN_POINT('',(60.8054892120567,214.197609441503,23.8713203435596)) ;
#76721=CARTESIAN_POINT('',(60.8054892120567,214.197609441503,23.8713203435596)) ;
#76722=CARTESIAN_POINT('',(60.8382191089243,214.038138460174,23.8713203435596)) ;
#76723=CARTESIAN_POINT('Origin',(73.0542750642243,222.307841389544,23.8713203435596)) ;
#76724=CARTESIAN_POINT('',(60.8382191089243,214.038138460174,23.7513203435596)) ;
#76725=CARTESIAN_POINT('',(60.8382191089243,214.038138460174,17.9913203435596)) ;
#76726=CARTESIAN_POINT('',(60.8382191089244,214.038138460174,17.9913203435596)) ;
#76727=CARTESIAN_POINT('Origin',(202.163078386837,317.851891258764,17.9913203435596)) ;
#76728=CARTESIAN_POINT('Ctrl Pts',(60.5916108526749,215.31305736582,23.4393203435596)) ;
#76729=CARTESIAN_POINT('Ctrl Pts',(60.5916108526749,215.31305736582,31.7577203435596)) ;
#76730=CARTESIAN_POINT('Ctrl Pts',(60.7075588580463,214.669276583145,23.4393203435596)) ;
#76731=CARTESIAN_POINT('Ctrl Pts',(60.7075588580463,214.669276583145,31.7577203435596)) ;
#76732=CARTESIAN_POINT('Ctrl Pts',(60.9588614284726,213.392541047196,23.4393203435596)) ;
#76733=CARTESIAN_POINT('Ctrl Pts',(60.9588614284726,213.392541047196,31.7577203435596)) ;
#76734=CARTESIAN_POINT('Ctrl Pts',(61.3940337100567,211.509915132417,23.4393203435596)) ;
#76735=CARTESIAN_POINT('Ctrl Pts',(61.3940337100567,211.509915132417,31.7577203435596)) ;
#76736=CARTESIAN_POINT('Ctrl Pts',(62.0926267016154,209.065776691758,23.4393203435596)) ;
#76737=CARTESIAN_POINT('Ctrl Pts',(62.0926267016154,209.065776691758,31.7577203435596)) ;
#76738=CARTESIAN_POINT('Ctrl Pts',(63.176438760595,206.128071441506,23.4393203435596)) ;
#76739=CARTESIAN_POINT('Ctrl Pts',(63.176438760595,206.128071441506,31.7577203435596)) ;
#76740=CARTESIAN_POINT('Ctrl Pts',(64.4892878686988,203.318135454206,23.4393203435596)) ;
#76741=CARTESIAN_POINT('Ctrl Pts',(64.4892878686988,203.318135454206,31.7577203435596)) ;
#76742=CARTESIAN_POINT('Ctrl Pts',(66.0493169032885,200.646089808857,23.4393203435596)) ;
#76743=CARTESIAN_POINT('Ctrl Pts',(66.0493169032885,200.646089808857,31.7577203435596)) ;
#76744=CARTESIAN_POINT('Ctrl Pts',(67.8654194647057,198.116895837109,23.4393203435596)) ;
#76745=CARTESIAN_POINT('Ctrl Pts',(67.8654194647057,198.116895837109,31.7577203435596)) ;
#76746=CARTESIAN_POINT('Ctrl Pts',(69.9262808608795,195.724241591299,23.4393203435596)) ;
#76747=CARTESIAN_POINT('Ctrl Pts',(69.9262808608795,195.724241591299,31.7577203435596)) ;
#76748=CARTESIAN_POINT('Ctrl Pts',(72.2129379945247,193.457548429354,23.4393203435596)) ;
#76749=CARTESIAN_POINT('Ctrl Pts',(72.2129379945247,193.457548429354,31.7577203435596)) ;
#76750=CARTESIAN_POINT('Ctrl Pts',(74.2078323511403,191.736557054229,23.4393203435596)) ;
#76751=CARTESIAN_POINT('Ctrl Pts',(74.2078323511403,191.736557054229,31.7577203435596)) ;
#76752=CARTESIAN_POINT('Ctrl Pts',(75.7911794288343,190.494445187268,23.4393203435596)) ;
#76753=CARTESIAN_POINT('Ctrl Pts',(75.7911794288343,190.494445187268,31.7577203435596)) ;
#76754=CARTESIAN_POINT('Ctrl Pts',(76.884855729364,189.687631312612,23.4393203435596)) ;
#76755=CARTESIAN_POINT('Ctrl Pts',(76.884855729364,189.687631312612,31.7577203435596)) ;
#76756=CARTESIAN_POINT('Ctrl Pts',(77.4412221473412,189.289539758744,23.4393203435596)) ;
#76757=CARTESIAN_POINT('Ctrl Pts',(77.4412221473412,189.289539758744,31.7577203435596)) ;
#76758=CARTESIAN_POINT('',(60.7651166309946,214.398081303037,23.8713203435596)) ;
#76759=CARTESIAN_POINT('',(60.7651166309946,214.398081303037,23.8713203435596)) ;
#76760=CARTESIAN_POINT('Origin',(72.876859665819,222.190806294465,23.8713203435596)) ;
#76761=CARTESIAN_POINT('Ctrl Pts',(60.7651166309946,214.398081303037,23.8713203435596)) ;
#76762=CARTESIAN_POINT('Ctrl Pts',(60.7651166309946,214.398081303037,31.5273203435596)) ;
#76763=CARTESIAN_POINT('Ctrl Pts',(60.6498192105232,214.976733877232,23.8713203435596)) ;
#76764=CARTESIAN_POINT('Ctrl Pts',(60.6498192105232,214.976733877232,31.5273203435596)) ;
#76765=CARTESIAN_POINT('Ctrl Pts',(60.5916108526749,215.56674656005,23.8713203435596)) ;
#76766=CARTESIAN_POINT('Ctrl Pts',(60.5916108526749,215.56674656005,31.5273203435596)) ;
#76767=CARTESIAN_POINT('Ctrl Pts',(60.5916108526749,216.156773929576,23.8713203435596)) ;
#76768=CARTESIAN_POINT('Ctrl Pts',(60.5916108526749,216.156773929576,31.5273203435596)) ;
#76769=CARTESIAN_POINT('',(60.5916108526749,216.156773929576,23.8713203435596)) ;
#76770=CARTESIAN_POINT('',(60.5916108526749,216.156773929576,30.2513203435596)) ;
#76771=CARTESIAN_POINT('Ctrl Pts',(60.5916108526749,216.156773929576,23.8713203435596)) ;
#76772=CARTESIAN_POINT('Ctrl Pts',(60.5916108526749,215.861760359297,23.8713203435596)) ;
#76773=CARTESIAN_POINT('Ctrl Pts',(60.606162930897,215.566750345658,23.8713203435596)) ;
#76774=CARTESIAN_POINT('Ctrl Pts',(60.664091487419,214.979573790456,23.8713203435596)) ;
#76775=CARTESIAN_POINT('Ctrl Pts',(60.7074679431304,214.687407477857,23.8713203435596)) ;
#76776=CARTESIAN_POINT('Ctrl Pts',(60.7651166309946,214.398081303037,23.8713203435596)) ;
#76777=CARTESIAN_POINT('Origin',(60.5916108526749,219.547374675056,23.8713203435596)) ;
#76778=CARTESIAN_POINT('',(60.5916108526749,219.547374675056,23.8713203435596)) ;
#76779=CARTESIAN_POINT('',(60.5916108526749,219.547374675056,23.8713203435596)) ;
#76780=CARTESIAN_POINT('',(60.5916108526749,220.645409008718,23.8713203435596)) ;
#76781=CARTESIAN_POINT('Origin',(60.6037668263229,219.566828299419,23.8713203435596)) ;
#76782=CARTESIAN_POINT('',(60.6037668263229,219.566828299419,23.8713203435596)) ;
#76783=CARTESIAN_POINT('',(60.6037668263229,219.566828299419,23.8713203435596)) ;
#76784=CARTESIAN_POINT('',(63.8582048387328,224.775017823302,23.8713203435596)) ;
#76785=CARTESIAN_POINT('Origin',(64.1568347953872,220.146231446812,23.8713203435596)) ;
#76786=CARTESIAN_POINT('',(60.5916108526749,219.647053884905,23.8713203435596)) ;
#76787=CARTESIAN_POINT('',(60.5916108526749,219.647053884905,23.8713203435596)) ;
#76788=CARTESIAN_POINT('Origin',(64.1568347953872,220.146231446812,23.8713203435596)) ;
#76789=CARTESIAN_POINT('Origin',(60.5916108526749,220.645409008718,23.8713203435596)) ;
#76790=CARTESIAN_POINT('',(60.5916108526749,220.645409008718,23.8713203435596)) ;
#76791=CARTESIAN_POINT('',(60.5916108526749,220.645409008718,23.8713203435596)) ;
#76792=CARTESIAN_POINT('',(60.5916108526749,220.645409008718,23.8713203435596)) ;
#76793=CARTESIAN_POINT('Origin',(64.1568347953872,220.146231446812,30.2513203435596)) ;
#76794=CARTESIAN_POINT('',(61.7916108526749,217.432246240363,30.2513203435596)) ;
#76795=CARTESIAN_POINT('Ctrl Pts',(61.671610852675,217.7102384348,30.3713203435596)) ;
#76796=CARTESIAN_POINT('Ctrl Pts',(61.6721253819932,217.708978462956,30.3713203435596)) ;
#76797=CARTESIAN_POINT('Ctrl Pts',(61.6726402662739,217.70771859947,30.3713170343059)) ;
#76798=CARTESIAN_POINT('Ctrl Pts',(61.6962023853316,217.650109410363,30.3710137213554)) ;
#76799=CARTESIAN_POINT('Ctrl Pts',(61.7186676884083,217.597219366085,30.3641419360414)) ;
#76800=CARTESIAN_POINT('Ctrl Pts',(61.7513364234646,217.522083093465,30.3424118695719)) ;
#76801=CARTESIAN_POINT('Ctrl Pts',(61.7626310589793,217.496635439055,30.3311044721307)) ;
#76802=CARTESIAN_POINT('Ctrl Pts',(61.7762176463779,217.466271908482,30.3107533540404)) ;
#76803=CARTESIAN_POINT('Ctrl Pts',(61.780952629944,217.455762082477,30.3019796043198)) ;
#76804=CARTESIAN_POINT('Ctrl Pts',(61.7868899451735,217.44263800318,30.2853058545662)) ;
#76805=CARTESIAN_POINT('Ctrl Pts',(61.7888011111258,217.438427571582,30.2782891621224)) ;
#76806=CARTESIAN_POINT('Ctrl Pts',(61.7910596764519,217.433457069678,30.2644053677528)) ;
#76807=CARTESIAN_POINT('Ctrl Pts',(61.7916108526749,217.432246240364,30.257961146373)) ;
#76808=CARTESIAN_POINT('Ctrl Pts',(61.7916108526749,217.432246240364,30.2513203435596)) ;
#76809=CARTESIAN_POINT('',(67.7485452644419,219.902067758924,30.2513203435596)) ;
#76810=CARTESIAN_POINT('Origin',(64.1568347953872,220.146231446812,30.2513203435596)) ;
#76811=CARTESIAN_POINT('Ctrl Pts',(67.635124836556,220.037151707603,30.3713203435596)) ;
#76812=CARTESIAN_POINT('Ctrl Pts',(67.6356227882016,220.036569616232,30.3713203435596)) ;
#76813=CARTESIAN_POINT('Ctrl Pts',(67.636120674921,220.035987456957,30.3713170159727)) ;
#76814=CARTESIAN_POINT('Ctrl Pts',(67.6490217074181,220.020899064839,30.371144461022)) ;
#76815=CARTESIAN_POINT('Ctrl Pts',(67.6614649298788,220.006254419689,30.3689095647645)) ;
#76816=CARTESIAN_POINT('Ctrl Pts',(67.6846753402724,219.978777532849,30.3602924369633)) ;
#76817=CARTESIAN_POINT('Ctrl Pts',(67.6956816716256,219.965671687184,30.3540979027369)) ;
#76818=CARTESIAN_POINT('Ctrl Pts',(67.7154693827078,219.941997430011,30.337552097772)) ;
#76819=CARTESIAN_POINT('Ctrl Pts',(67.7244805588803,219.931158578531,30.327243797285)) ;
#76820=CARTESIAN_POINT('Ctrl Pts',(67.7371840595297,219.915830858124,30.3052692101847)) ;
#76821=CARTESIAN_POINT('Ctrl Pts',(67.7416269457272,219.910452972978,30.2947007603144)) ;
#76822=CARTESIAN_POINT('Ctrl Pts',(67.7471684473396,219.903738959239,30.2728956002824)) ;
#76823=CARTESIAN_POINT('Ctrl Pts',(67.7485452644419,219.902067758924,30.26223415745)) ;
#76824=CARTESIAN_POINT('Ctrl Pts',(67.7485452644419,219.902067758924,30.2513203435596)) ;
#76825=CARTESIAN_POINT('Ctrl Pts',(62.1439228384234,214.067655379578,30.2513203435596)) ;
#76826=CARTESIAN_POINT('Ctrl Pts',(62.1222982033092,214.069755004928,30.2513203435596)) ;
#76827=CARTESIAN_POINT('Ctrl Pts',(62.0731635470014,214.088684352254,30.2513203435596)) ;
#76828=CARTESIAN_POINT('Ctrl Pts',(62.044013686833,214.13412578273,30.2513203435596)) ;
#76829=CARTESIAN_POINT('Ctrl Pts',(62.0380714133749,214.162478201405,30.2513203435596)) ;
#76830=CARTESIAN_POINT('Ctrl Pts',(62.1439228384234,214.067655379578,30.2872242596007)) ;
#76831=CARTESIAN_POINT('Ctrl Pts',(62.1223673122467,214.069748294855,30.2872242596007)) ;
#76832=CARTESIAN_POINT('Ctrl Pts',(62.0732712928142,214.088723191247,30.2872242596007)) ;
#76833=CARTESIAN_POINT('Ctrl Pts',(62.0439946962603,214.134216392607,30.2872242596007)) ;
#76834=CARTESIAN_POINT('Ctrl Pts',(62.0380714133749,214.162478201405,30.2872242596007)) ;
#76835=CARTESIAN_POINT('Ctrl Pts',(62.1410083285202,214.03763801805,30.3493567156287)) ;
#76836=CARTESIAN_POINT('Ctrl Pts',(62.1139330407202,214.040266869835,30.3493567156287)) ;
#76837=CARTESIAN_POINT('Ctrl Pts',(62.0524409085205,214.063943061966,30.3493567156287)) ;
#76838=CARTESIAN_POINT('Ctrl Pts',(62.0159942853878,214.120792946662,30.3493567156287)) ;
#76839=CARTESIAN_POINT('Ctrl Pts',(62.0085542170022,214.156291806707,30.3493567156287)) ;
#76840=CARTESIAN_POINT('Ctrl Pts',(62.1349283836427,213.975018946742,30.3713203435596)) ;
#76841=CARTESIAN_POINT('Ctrl Pts',(62.0965217439458,213.978748006395,30.3713203435596)) ;
#76842=CARTESIAN_POINT('Ctrl Pts',(62.0092726729388,214.012352423146,30.3713203435596)) ;
#76843=CARTESIAN_POINT('Ctrl Pts',(61.9575323693022,214.093030815,30.3713203435596)) ;
#76844=CARTESIAN_POINT('Ctrl Pts',(61.9469785377818,214.143386398936,30.3713203435596)) ;
#76845=CARTESIAN_POINT('Ctrl Pts',(62.1323260763097,213.948217047756,30.3713203435596)) ;
#76846=CARTESIAN_POINT('Ctrl Pts',(62.0890768060814,213.952416298455,30.3713203435596)) ;
#76847=CARTESIAN_POINT('Ctrl Pts',(61.9908074934658,213.990274993108,30.3713203435596)) ;
#76848=CARTESIAN_POINT('Ctrl Pts',(61.932507773129,214.081157854061,30.3713203435596)) ;
#76849=CARTESIAN_POINT('Ctrl Pts',(61.9206232262128,214.13786269141,30.3713203435596)) ;
#76850=CARTESIAN_POINT('',(62.1439228384234,214.067655379578,30.2513203435596)) ;
#76851=CARTESIAN_POINT('Origin',(62.1323260763097,213.948217047756,30.2513203435596)) ;
#76852=CARTESIAN_POINT('',(62.0380714133749,214.162478201405,30.2513203435596)) ;
#76853=CARTESIAN_POINT('Ctrl Pts',(62.1439228384234,214.067655379578,30.2513203435596)) ;
#76854=CARTESIAN_POINT('Ctrl Pts',(62.115089064211,214.070454970089,30.2513203435596)) ;
#76855=CARTESIAN_POINT('Ctrl Pts',(62.0667252302728,214.094448639981,30.2513203435596)) ;
#76856=CARTESIAN_POINT('Ctrl Pts',(62.0425282618161,214.141213203443,30.2513203435596)) ;
#76857=CARTESIAN_POINT('Ctrl Pts',(62.0380714133749,214.162478201405,30.2513203435596)) ;
#76858=CARTESIAN_POINT('Origin',(61.9206232262128,214.13786269141,30.2513203435596)) ;
#76859=CARTESIAN_POINT('Origin',(62.155519600537,214.1870937114,26.4913203435596)) ;
#76860=CARTESIAN_POINT('',(62.0380714133749,214.162478201405,26.4913203435596)) ;
#76861=CARTESIAN_POINT('',(62.1555196005219,214.187093711472,26.3713203435596)) ;
#76862=CARTESIAN_POINT('Origin',(62.155519600537,214.1870937114,26.4913203435596)) ;
#76863=CARTESIAN_POINT('',(62.1439228384234,214.067655379578,26.4913203435596)) ;
#76864=CARTESIAN_POINT('Origin',(62.155519600537,214.1870937114,26.4913203435596)) ;
#76865=CARTESIAN_POINT('Origin',(62.1555196004967,214.187093711404,26.4913203435596)) ;
#76866=CARTESIAN_POINT('Ctrl Pts',(62.1439228384234,214.067655379578,26.4913203435596)) ;
#76867=CARTESIAN_POINT('Ctrl Pts',(62.1439228384234,214.067655379578,31.0033203435597)) ;
#76868=CARTESIAN_POINT('Ctrl Pts',(62.115089064211,214.070454970089,26.4913203435596)) ;
#76869=CARTESIAN_POINT('Ctrl Pts',(62.115089064211,214.070454970089,31.0033203435597)) ;
#76870=CARTESIAN_POINT('Ctrl Pts',(62.0667252302728,214.094448639981,26.4913203435596)) ;
#76871=CARTESIAN_POINT('Ctrl Pts',(62.0667252302728,214.094448639981,31.0033203435597)) ;
#76872=CARTESIAN_POINT('Ctrl Pts',(62.0425282618161,214.141213203443,26.4913203435596)) ;
#76873=CARTESIAN_POINT('Ctrl Pts',(62.0425282618161,214.141213203443,31.0033203435597)) ;
#76874=CARTESIAN_POINT('Ctrl Pts',(62.0380714133749,214.162478201405,26.4913203435596)) ;
#76875=CARTESIAN_POINT('Ctrl Pts',(62.0380714133749,214.162478201405,31.0033203435597)) ;
#76876=CARTESIAN_POINT('',(62.1439228384234,214.067655379578,30.2513203435597)) ;
#76877=CARTESIAN_POINT('',(62.0380714133749,214.162478201405,26.4913203435596)) ;
#76878=CARTESIAN_POINT('Ctrl Pts',(69.2413920554874,213.523097238281,30.2513203435596)) ;
#76879=CARTESIAN_POINT('Ctrl Pts',(69.2429622182083,213.507997501652,30.2513203435596)) ;
#76880=CARTESIAN_POINT('Ctrl Pts',(69.2398976738995,213.472038237813,30.2513203435596)) ;
#76881=CARTESIAN_POINT('Ctrl Pts',(69.2135287770271,213.426976369741,30.2513203435596)) ;
#76882=CARTESIAN_POINT('Ctrl Pts',(69.1666694054386,213.395034372691,30.2513203435596)) ;
#76883=CARTESIAN_POINT('Ctrl Pts',(69.1305856629887,213.38929136102,30.2513203435596)) ;
#76884=CARTESIAN_POINT('Ctrl Pts',(69.1104388653291,213.391247497013,30.2513203435596)) ;
#76885=CARTESIAN_POINT('Ctrl Pts',(69.2413920554874,213.523097238281,30.2872242596007)) ;
#76886=CARTESIAN_POINT('Ctrl Pts',(69.2429572002149,213.508045758039,30.2872242596007)) ;
#76887=CARTESIAN_POINT('Ctrl Pts',(69.2398004488935,213.472098680599,30.2872242596007)) ;
#76888=CARTESIAN_POINT('Ctrl Pts',(69.2134077180135,213.427071983451,30.2872242596007)) ;
#76889=CARTESIAN_POINT('Ctrl Pts',(69.1666433975403,213.395176978348,30.2872242596007)) ;
#76890=CARTESIAN_POINT('Ctrl Pts',(69.1305212769876,213.389297612523,30.2872242596007)) ;
#76891=CARTESIAN_POINT('Ctrl Pts',(69.1104388653291,213.391247497013,30.2872242596007)) ;
#76892=CARTESIAN_POINT('Ctrl Pts',(69.271388915094,213.526216494719,30.3493566164462)) ;
#76893=CARTESIAN_POINT('Ctrl Pts',(69.2733548491936,213.507310755373,30.3493566164462)) ;
#76894=CARTESIAN_POINT('Ctrl Pts',(69.2695413496691,213.462311342459,30.3493566164462)) ;
#76895=CARTESIAN_POINT('Ctrl Pts',(69.2365508649147,213.405916351071,30.3493566164462)) ;
#76896=CARTESIAN_POINT('Ctrl Pts',(69.1778928305879,213.365935817039,30.3493566164462)) ;
#76897=CARTESIAN_POINT('Ctrl Pts',(69.1327492976852,213.358780858359,30.3493566164462)) ;
#76898=CARTESIAN_POINT('Ctrl Pts',(69.1075243474375,213.36123005321,30.3493566164462)) ;
#76899=CARTESIAN_POINT('Ctrl Pts',(69.3339649637103,213.532723533959,30.3713203435596)) ;
#76900=CARTESIAN_POINT('Ctrl Pts',(69.336753666205,213.505905502527,30.3713203435596)) ;
#76901=CARTESIAN_POINT('Ctrl Pts',(69.3313255035809,213.442054464431,30.3713203435596)) ;
#76902=CARTESIAN_POINT('Ctrl Pts',(69.2845082997786,213.362037536173,30.3713203435596)) ;
#76903=CARTESIAN_POINT('Ctrl Pts',(69.2012911226345,213.305314559911,30.3713203435596)) ;
#76904=CARTESIAN_POINT('Ctrl Pts',(69.1372263229216,213.295136850167,30.3713203435596)) ;
#76905=CARTESIAN_POINT('Ctrl Pts',(69.1014444105484,213.298611064177,30.3713203435596)) ;
#76906=CARTESIAN_POINT('Ctrl Pts',(69.360748483532,213.535508647726,30.3713203435596)) ;
#76907=CARTESIAN_POINT('Ctrl Pts',(69.3638888089739,213.505309174469,30.3713203435596)) ;
#76908=CARTESIAN_POINT('Ctrl Pts',(69.3577597203562,213.433390646791,30.3713203435596)) ;
#76909=CARTESIAN_POINT('Ctrl Pts',(69.3050219266113,213.343266910648,30.3713203435596)) ;
#76910=CARTESIAN_POINT('Ctrl Pts',(69.2113031834343,213.279382916547,30.3713203435596)) ;
#76911=CARTESIAN_POINT('Ctrl Pts',(69.1391356985346,213.267896893205,30.3713203435596)) ;
#76912=CARTESIAN_POINT('Ctrl Pts',(69.0988421032155,213.27180916519,30.3713203435596)) ;
#76913=CARTESIAN_POINT('',(69.2413920554874,213.523097238281,30.2513203435596)) ;
#76914=CARTESIAN_POINT('Origin',(69.360748483532,213.535508647726,30.2513203435596)) ;
#76915=CARTESIAN_POINT('',(69.1104388653291,213.391247497013,30.2513203435596)) ;
#76916=CARTESIAN_POINT('Ctrl Pts',(69.2413920554874,213.523097238281,30.2513203435596)) ;
#76917=CARTESIAN_POINT('Ctrl Pts',(69.2434856838755,213.502963505109,30.2513203435596)) ;
#76918=CARTESIAN_POINT('Ctrl Pts',(69.237232259097,213.461730274006,30.2513203435596)) ;
#76919=CARTESIAN_POINT('Ctrl Pts',(69.1926794105975,213.403591641984,30.2513203435596)) ;
#76920=CARTESIAN_POINT('Ctrl Pts',(69.1406601890908,213.388313183572,30.2513203435596)) ;
#76921=CARTESIAN_POINT('Ctrl Pts',(69.1104388653291,213.391247497013,30.2513203435596)) ;
#76922=CARTESIAN_POINT('Origin',(69.0988421032155,213.27180916519,30.2513203435596)) ;
#76923=CARTESIAN_POINT('Origin',(69.1220356274428,213.510685828835,26.4913203435596)) ;
#76924=CARTESIAN_POINT('',(69.1104388653291,213.391247497013,26.4913203435596)) ;
#76925=CARTESIAN_POINT('',(69.1220356292711,213.51068582655,26.3713203435596)) ;
#76926=CARTESIAN_POINT('Origin',(69.1220356274428,213.510685828835,26.4913203435596)) ;
#76927=CARTESIAN_POINT('',(69.2403544421435,213.490669383401,26.4913203435596)) ;
#76928=CARTESIAN_POINT('Origin',(69.1220356274428,213.510685828835,26.4913203435596)) ;
#76929=CARTESIAN_POINT('',(69.2413920554874,213.523097238281,26.4913203435596)) ;
#76930=CARTESIAN_POINT('Origin',(69.1220356274428,213.510685828835,26.4913203435596)) ;
#76931=CARTESIAN_POINT('Origin',(69.1220356281404,213.510685822126,26.4913203435596)) ;
#76932=CARTESIAN_POINT('Ctrl Pts',(69.2413920554874,213.523097238281,26.4913203435596)) ;
#76933=CARTESIAN_POINT('Ctrl Pts',(69.2413920554874,213.523097238281,31.0033203435596)) ;
#76934=CARTESIAN_POINT('Ctrl Pts',(69.2434856838755,213.502963505109,26.4913203435596)) ;
#76935=CARTESIAN_POINT('Ctrl Pts',(69.2434856838755,213.502963505109,31.0033203435596)) ;
#76936=CARTESIAN_POINT('Ctrl Pts',(69.237232259097,213.461730274006,26.4913203435596)) ;
#76937=CARTESIAN_POINT('Ctrl Pts',(69.237232259097,213.461730274006,31.0033203435596)) ;
#76938=CARTESIAN_POINT('Ctrl Pts',(69.1926794105975,213.403591641984,26.4913203435596)) ;
#76939=CARTESIAN_POINT('Ctrl Pts',(69.1926794105975,213.403591641984,31.0033203435596)) ;
#76940=CARTESIAN_POINT('Ctrl Pts',(69.1406601890908,213.388313183572,26.4913203435596)) ;
#76941=CARTESIAN_POINT('Ctrl Pts',(69.1406601890908,213.388313183572,31.0033203435596)) ;
#76942=CARTESIAN_POINT('Ctrl Pts',(69.1104388653291,213.391247497013,26.4913203435596)) ;
#76943=CARTESIAN_POINT('Ctrl Pts',(69.1104388653291,213.391247497013,31.0033203435596)) ;
#76944=CARTESIAN_POINT('',(69.2413920554874,213.523097238281,30.2513203435596)) ;
#76945=CARTESIAN_POINT('',(69.1104388653291,213.391247497013,26.4913203435596)) ;
#76946=CARTESIAN_POINT('Ctrl Pts',(69.1686691234544,219.464553538579,26.4913203435596)) ;
#76947=CARTESIAN_POINT('Ctrl Pts',(69.075747399216,218.242094170941,26.4913203435596)) ;
#76948=CARTESIAN_POINT('Ctrl Pts',(69.0471488167689,217.014745324447,26.4913203435596)) ;
#76949=CARTESIAN_POINT('Ctrl Pts',(69.0872384835382,215.789690777862,26.4913203435596)) ;
#76950=CARTESIAN_POINT('Ctrl Pts',(69.1686691234544,219.464553538579,26.4554164275186)) ;
#76951=CARTESIAN_POINT('Ctrl Pts',(69.0757484199277,218.242107599218,26.4554164275186)) ;
#76952=CARTESIAN_POINT('Ctrl Pts',(69.0471492860395,217.014730984541,26.4554164275186)) ;
#76953=CARTESIAN_POINT('Ctrl Pts',(69.0872384835382,215.789690777862,26.4554164275186)) ;
#76954=CARTESIAN_POINT('Ctrl Pts',(69.1385972482844,219.466839365467,26.3932840972059)) ;
#76955=CARTESIAN_POINT('Ctrl Pts',(69.0455950200553,218.243320903646,26.3932840972059)) ;
#76956=CARTESIAN_POINT('Ctrl Pts',(69.0169693155449,217.014889912194,26.3932840972059)) ;
#76957=CARTESIAN_POINT('Ctrl Pts',(69.0570959938923,215.788704370874,26.3932840972059)) ;
#76958=CARTESIAN_POINT('Ctrl Pts',(69.0758647787493,219.471607793269,26.3713203435596)) ;
#76959=CARTESIAN_POINT('Ctrl Pts',(68.9826951909212,218.245887582489,26.3713203435596)) ;
#76960=CARTESIAN_POINT('Ctrl Pts',(68.9540125949514,217.015183406856,26.3713203435596)) ;
#76961=CARTESIAN_POINT('Ctrl Pts',(68.9942162166009,215.786646642648,26.3713203435596)) ;
#76962=CARTESIAN_POINT('Ctrl Pts',(69.0490142989096,219.473648755078,26.3713203435596)) ;
#76963=CARTESIAN_POINT('Ctrl Pts',(68.9557731873382,218.246987592431,26.3713203435596)) ;
#76964=CARTESIAN_POINT('Ctrl Pts',(68.9270661821599,217.015307498826,26.3713203435596)) ;
#76965=CARTESIAN_POINT('Ctrl Pts',(68.9673026867335,215.785765902728,26.3713203435596)) ;
#76966=CARTESIAN_POINT('',(69.1686691234544,219.464553538579,26.4913203435596)) ;
#76967=CARTESIAN_POINT('',(69.0490142989096,219.473648755078,26.3713203435596)) ;
#76968=CARTESIAN_POINT('Origin',(69.0490142989096,219.473648755078,26.4913203435596)) ;
#76969=CARTESIAN_POINT('',(68.9673026867972,215.785765900781,26.3713203435596)) ;
#76970=CARTESIAN_POINT('Origin',(98.8235066990713,222.791430341492,26.3713203435596)) ;
#76971=CARTESIAN_POINT('',(69.0872384836096,215.78969077568,26.4913203435596)) ;
#76972=CARTESIAN_POINT('Origin',(68.9673026867335,215.785765902728,26.4913203435596)) ;
#76973=CARTESIAN_POINT('Origin',(98.5678225429277,222.744057364665,26.4913203435596)) ;
#76974=CARTESIAN_POINT('Ctrl Pts',(69.087238483681,215.789690773497,26.4913203435596)) ;
#76975=CARTESIAN_POINT('Ctrl Pts',(69.1120141497305,215.032599366639,26.4913203435596)) ;
#76976=CARTESIAN_POINT('Ctrl Pts',(69.1630580206422,214.276409794352,26.4913203435596)) ;
#76977=CARTESIAN_POINT('Ctrl Pts',(69.2413920561824,213.523097231597,26.4913203435596)) ;
#76978=CARTESIAN_POINT('Ctrl Pts',(69.087238483681,215.789690773497,26.4554164275186)) ;
#76979=CARTESIAN_POINT('Ctrl Pts',(69.1120138597183,215.032608228791,26.4554164275186)) ;
#76980=CARTESIAN_POINT('Ctrl Pts',(69.163058978161,214.27640058621,26.4554164275186)) ;
#76981=CARTESIAN_POINT('Ctrl Pts',(69.2413920561824,213.523097231597,26.4554164275186)) ;
#76982=CARTESIAN_POINT('Ctrl Pts',(69.0570960390057,215.788704367977,26.3932840432188)) ;
#76983=CARTESIAN_POINT('Ctrl Pts',(69.0818945784431,215.030913999266,26.3932840432188)) ;
#76984=CARTESIAN_POINT('Ctrl Pts',(69.1329856638633,214.274016790527,26.3932840432188)) ;
#76985=CARTESIAN_POINT('Ctrl Pts',(69.211395219335,213.519977977518,26.3932840432188)) ;
#76986=CARTESIAN_POINT('Ctrl Pts',(68.9942162167441,215.786646638271,26.3713203435596)) ;
#76987=CARTESIAN_POINT('Ctrl Pts',(69.0190623076259,215.027403199043,26.3713203435596)) ;
#76988=CARTESIAN_POINT('Ctrl Pts',(69.0702525942423,214.26901954923,26.3713203435596)) ;
#76989=CARTESIAN_POINT('Ctrl Pts',(69.1488191479615,213.513470935898,26.3713203435596)) ;
#76990=CARTESIAN_POINT('Ctrl Pts',(68.9673026868768,215.785765898347,26.3713203435596)) ;
#76991=CARTESIAN_POINT('Ctrl Pts',(68.9921690996123,215.025901466698,26.3713203435596)) ;
#76992=CARTESIAN_POINT('Ctrl Pts',(69.0434019787636,214.266879672249,26.3713203435596)) ;
#76993=CARTESIAN_POINT('Ctrl Pts',(69.1220356281404,213.510685822126,26.3713203435596)) ;
#76994=CARTESIAN_POINT('Origin',(97.1540654702609,222.393518409093,26.4913203435596)) ;
#76995=CARTESIAN_POINT('Origin',(97.133994720273,222.390783272674,26.3713203435596)) ;
#76996=CARTESIAN_POINT('Origin',(67.2629739196944,213.691189826592,26.4913203435596)) ;
#76997=CARTESIAN_POINT('',(67.2513771575808,213.57175149477,26.4913203435596)) ;
#76998=CARTESIAN_POINT('',(67.2629739196944,213.691189826592,26.3713203435596)) ;
#76999=CARTESIAN_POINT('Origin',(69.2461649893318,213.257504976258,30.2513203435596)) ;
#77000=CARTESIAN_POINT('',(69.2577617514454,213.37694330808,30.2513203435596)) ;
#77001=CARTESIAN_POINT('Ctrl Pts',(69.1987989853619,219.837084335145,30.2513203435596)) ;
#77002=CARTESIAN_POINT('Ctrl Pts',(69.195605783884,219.798820218195,30.2513203435596)) ;
#77003=CARTESIAN_POINT('Ctrl Pts',(69.1924125824061,219.760556101245,30.2513203435596)) ;
#77004=CARTESIAN_POINT('Ctrl Pts',(69.1892193809281,219.722291984294,30.2513203435596)) ;
#77005=CARTESIAN_POINT('Ctrl Pts',(69.1820520081344,219.636405392827,30.2513203435596)) ;
#77006=CARTESIAN_POINT('Ctrl Pts',(69.1752014751529,219.550491833333,30.2513203435596)) ;
#77007=CARTESIAN_POINT('Ctrl Pts',(69.1686691234544,219.464553538581,30.2513203435596)) ;
#77008=CARTESIAN_POINT('Ctrl Pts',(69.1987989853619,219.837084335145,30.2872242596007)) ;
#77009=CARTESIAN_POINT('Ctrl Pts',(69.195605783884,219.798820218195,30.2872242596007)) ;
#77010=CARTESIAN_POINT('Ctrl Pts',(69.1924125824061,219.760556101245,30.2872242596007)) ;
#77011=CARTESIAN_POINT('Ctrl Pts',(69.1892193809281,219.722291984294,30.2872242596007)) ;
#77012=CARTESIAN_POINT('Ctrl Pts',(69.1820520081344,219.636405392827,30.2872242596007)) ;
#77013=CARTESIAN_POINT('Ctrl Pts',(69.1752014751529,219.550491833333,30.2872242596007)) ;
#77014=CARTESIAN_POINT('Ctrl Pts',(69.1686691234544,219.464553538581,30.2872242596007)) ;
#77015=CARTESIAN_POINT('Ctrl Pts',(69.2288531922854,219.834576263729,30.3493565283418)) ;
#77016=CARTESIAN_POINT('Ctrl Pts',(69.2256599908075,219.796312146779,30.3493565283418)) ;
#77017=CARTESIAN_POINT('Ctrl Pts',(69.2224667893296,219.758048029829,30.3493565283418)) ;
#77018=CARTESIAN_POINT('Ctrl Pts',(69.2192735878516,219.719783912879,30.3493565283418)) ;
#77019=CARTESIAN_POINT('Ctrl Pts',(69.2121123842297,219.633971246513,30.3493565283418)) ;
#77020=CARTESIAN_POINT('Ctrl Pts',(69.205267758613,219.548131765938,30.3493565283418)) ;
#77021=CARTESIAN_POINT('Ctrl Pts',(69.1987410497925,219.462267707803,30.3493565283417)) ;
#77022=CARTESIAN_POINT('Ctrl Pts',(69.2915486465511,219.829344228257,30.3713203435596)) ;
#77023=CARTESIAN_POINT('Ctrl Pts',(69.2883554450732,219.791080111306,30.3713203435596)) ;
#77024=CARTESIAN_POINT('Ctrl Pts',(69.2851622435952,219.752815994356,30.3713203435596)) ;
#77025=CARTESIAN_POINT('Ctrl Pts',(69.2819690421173,219.714551877406,30.3713203435596)) ;
#77026=CARTESIAN_POINT('Ctrl Pts',(69.2748207078644,219.628893424645,30.3713203435596)) ;
#77027=CARTESIAN_POINT('Ctrl Pts',(69.2679884054781,219.543208478558,30.3713203435596)) ;
#77028=CARTESIAN_POINT('Ctrl Pts',(69.2614734681595,219.457499283891,30.3713203435596)) ;
#77029=CARTESIAN_POINT('Ctrl Pts',(69.3183833051634,219.827104833273,30.3713203435596)) ;
#77030=CARTESIAN_POINT('Ctrl Pts',(69.3151901036855,219.788840716323,30.3713203435596)) ;
#77031=CARTESIAN_POINT('Ctrl Pts',(69.3119969022076,219.750576599373,30.3713203435596)) ;
#77032=CARTESIAN_POINT('Ctrl Pts',(69.3088037007297,219.712312482423,30.3713203435596)) ;
#77033=CARTESIAN_POINT('Ctrl Pts',(69.3016608747709,219.626720035554,30.3713203435596)) ;
#77034=CARTESIAN_POINT('Ctrl Pts',(69.2948338469246,219.541101232703,30.3713203435596)) ;
#77035=CARTESIAN_POINT('Ctrl Pts',(69.2883239479992,219.455458322081,30.3713203435596)) ;
#77036=CARTESIAN_POINT('',(69.1892193814451,219.72229198423,30.2513203435596)) ;
#77037=CARTESIAN_POINT('',(69.1686691234544,219.46455353858,30.2513203435596)) ;
#77038=CARTESIAN_POINT('Origin',(98.9345171832154,222.024247258091,30.2513203435596)) ;
#77039=CARTESIAN_POINT('Origin',(69.2883239479992,219.455458322081,30.2513203435596)) ;
#77040=CARTESIAN_POINT('Ctrl Pts',(69.3183833051634,219.827104833273,30.3713203435596)) ;
#77041=CARTESIAN_POINT('Ctrl Pts',(69.318101580658,219.826871585683,30.3713203435596)) ;
#77042=CARTESIAN_POINT('Ctrl Pts',(69.3178198111958,219.826638390472,30.3713194568659)) ;
#77043=CARTESIAN_POINT('Ctrl Pts',(69.3028143009312,219.814224398279,30.3712250783813)) ;
#77044=CARTESIAN_POINT('Ctrl Pts',(69.2878306017834,219.802081997314,30.3687143086752)) ;
#77045=CARTESIAN_POINT('Ctrl Pts',(69.2597178898201,219.779423852337,30.3590473904662)) ;
#77046=CARTESIAN_POINT('Ctrl Pts',(69.2461518879997,219.768543441465,30.3519487591578)) ;
#77047=CARTESIAN_POINT('Ctrl Pts',(69.2217945704143,219.748610301608,30.3322980192289)) ;
#77048=CARTESIAN_POINT('Ctrl Pts',(69.2115959028757,219.740182294065,30.3201725243576)) ;
#77049=CARTESIAN_POINT('Ctrl Pts',(69.1994121293716,219.730311833466,30.2983574623926)) ;
#77050=CARTESIAN_POINT('Ctrl Pts',(69.1956759077495,219.727331200005,30.2894514633275)) ;
#77051=CARTESIAN_POINT('Ctrl Pts',(69.1905841803268,219.723326414298,30.2707124141225)) ;
#77052=CARTESIAN_POINT('Ctrl Pts',(69.1892193809281,219.722291984294,30.2610938408263)) ;
#77053=CARTESIAN_POINT('Ctrl Pts',(69.1892193809281,219.722291984294,30.2513203435596)) ;
#77054=CARTESIAN_POINT('Ctrl Pts',(69.1686691234544,219.464553538579,30.2513203435596)) ;
#77055=CARTESIAN_POINT('Ctrl Pts',(69.075767060595,218.242352832058,30.2513203435596)) ;
#77056=CARTESIAN_POINT('Ctrl Pts',(69.0471392129121,217.015038797788,30.2513203435596)) ;
#77057=CARTESIAN_POINT('Ctrl Pts',(69.0872384835382,215.789690777862,30.2513203435596)) ;
#77058=CARTESIAN_POINT('Ctrl Pts',(69.1686691234544,219.464553538579,30.2872242596007)) ;
#77059=CARTESIAN_POINT('Ctrl Pts',(69.0757660400992,218.242339406623,30.2872242596007)) ;
#77060=CARTESIAN_POINT('Ctrl Pts',(69.0471387435291,217.015053141129,30.2872242596007)) ;
#77061=CARTESIAN_POINT('Ctrl Pts',(69.0872384835382,215.789690777862,30.2872242596007)) ;
#77062=CARTESIAN_POINT('Ctrl Pts',(69.1987410451693,219.462267708153,30.3493565339049)) ;
#77063=CARTESIAN_POINT('Ctrl Pts',(69.1059194692668,218.241125871721,30.3493565339049)) ;
#77064=CARTESIAN_POINT('Ctrl Pts',(69.0773187696569,217.014893940627,30.3493565339049)) ;
#77065=CARTESIAN_POINT('Ctrl Pts',(69.1173810198383,215.790677186376,30.3493565339049)) ;
#77066=CARTESIAN_POINT('Ctrl Pts',(69.2614734681594,219.45749928389,30.3713203435596)) ;
#77067=CARTESIAN_POINT('Ctrl Pts',(69.1688192164441,218.238558730547,30.3713203435596)) ;
#77068=CARTESIAN_POINT('Ctrl Pts',(69.1402754620286,217.01459988118,30.3713203435596)) ;
#77069=CARTESIAN_POINT('Ctrl Pts',(69.1802607504755,215.792734913075,30.3713203435596)) ;
#77070=CARTESIAN_POINT('Ctrl Pts',(69.2883239479991,219.45545832208,30.3713203435596)) ;
#77071=CARTESIAN_POINT('Ctrl Pts',(69.1957412048934,218.237458521508,30.3713203435596)) ;
#77072=CARTESIAN_POINT('Ctrl Pts',(69.1672218826975,217.014475548494,30.3713203435596)) ;
#77073=CARTESIAN_POINT('Ctrl Pts',(69.2071742803429,215.793615652996,30.3713203435596)) ;
#77074=CARTESIAN_POINT('',(69.0872384836096,215.78969077568,30.2513203435596)) ;
#77075=CARTESIAN_POINT('Origin',(69.2071742803429,215.793615652996,30.2513203435596)) ;
#77076=CARTESIAN_POINT('Origin',(99.1895632998921,222.852119685147,30.2513203435596)) ;
#77077=CARTESIAN_POINT('Ctrl Pts',(69.087238483681,215.789690773497,30.2513203435596)) ;
#77078=CARTESIAN_POINT('Ctrl Pts',(69.1120101109511,215.032722783106,30.2513203435596)) ;
#77079=CARTESIAN_POINT('Ctrl Pts',(69.1630453951407,214.2765312112,30.2513203435596)) ;
#77080=CARTESIAN_POINT('Ctrl Pts',(69.2413920554874,213.523097238281,30.2513203435596)) ;
#77081=CARTESIAN_POINT('Ctrl Pts',(69.087238483681,215.789690773497,30.2872242596007)) ;
#77082=CARTESIAN_POINT('Ctrl Pts',(69.112010400916,215.032713922399,30.2872242596007)) ;
#77083=CARTESIAN_POINT('Ctrl Pts',(69.1630444374676,214.276540420826,30.2872242596007)) ;
#77084=CARTESIAN_POINT('Ctrl Pts',(69.2413920554874,213.523097238281,30.2872242596007)) ;
#77085=CARTESIAN_POINT('Ctrl Pts',(69.1173809762543,215.790677180585,30.3493565863989)) ;
#77086=CARTESIAN_POINT('Ctrl Pts',(69.1421297338651,215.034408038106,30.3493565863989)) ;
#77087=CARTESIAN_POINT('Ctrl Pts',(69.1931178117582,214.278924102927,30.3493565863989)) ;
#77088=CARTESIAN_POINT('Ctrl Pts',(69.2713889400021,213.526216497309,30.3493565863989)) ;
#77089=CARTESIAN_POINT('Ctrl Pts',(69.1802607506179,215.792734908723,30.3713203435596)) ;
#77090=CARTESIAN_POINT('Ctrl Pts',(69.204961964536,215.037918599891,30.3713203435596)) ;
#77091=CARTESIAN_POINT('Ctrl Pts',(69.2558508590168,214.283921095922,30.3713203435596)) ;
#77092=CARTESIAN_POINT('Ctrl Pts',(69.3339649637103,213.532723533959,30.3713203435596)) ;
#77093=CARTESIAN_POINT('Ctrl Pts',(69.2071742804852,215.793615648647,30.3713203435596)) ;
#77094=CARTESIAN_POINT('Ctrl Pts',(69.2318551758623,215.039420231006,30.3713203435596)) ;
#77095=CARTESIAN_POINT('Ctrl Pts',(69.2827014853096,214.286060868906,30.3713203435596)) ;
#77096=CARTESIAN_POINT('Ctrl Pts',(69.360748483532,213.535508647726,30.3713203435596)) ;
#77097=CARTESIAN_POINT('Origin',(97.219772055596,222.411726694737,30.2513203435596)) ;
#77098=CARTESIAN_POINT('Ctrl Pts',(62.0380714133749,214.162478201405,26.4913203435596)) ;
#77099=CARTESIAN_POINT('Ctrl Pts',(62.0151252295802,214.27196151861,26.4913203435596)) ;
#77100=CARTESIAN_POINT('Ctrl Pts',(61.9925614772325,214.381523697747,26.4913203435596)) ;
#77101=CARTESIAN_POINT('Ctrl Pts',(61.9703773266184,214.491161471123,26.4913203435596)) ;
#77102=CARTESIAN_POINT('Ctrl Pts',(62.0380714133749,214.162478201405,26.4554164275186)) ;
#77103=CARTESIAN_POINT('Ctrl Pts',(62.0151250465041,214.271962392122,26.4554164275186)) ;
#77104=CARTESIAN_POINT('Ctrl Pts',(61.9925616526852,214.381522830631,26.4554164275186)) ;
#77105=CARTESIAN_POINT('Ctrl Pts',(61.9703773266184,214.491161471123,26.4554164275186)) ;
#77106=CARTESIAN_POINT('Ctrl Pts',(62.0675885660411,214.168664586943,26.3932839179096)) ;
#77107=CARTESIAN_POINT('Ctrl Pts',(62.0446568215384,214.278079009834,26.3932839179096)) ;
#77108=CARTESIAN_POINT('Ctrl Pts',(62.0221070790419,214.387573156395,26.3932839179096)) ;
#77109=CARTESIAN_POINT('Ctrl Pts',(61.999936766457,214.497142539921,26.3932839179096)) ;
#77110=CARTESIAN_POINT('Ctrl Pts',(62.129164288968,214.181570003874,26.3713203435596)) ;
#77111=CARTESIAN_POINT('Ctrl Pts',(62.1062625622829,214.290841202503,26.3713203435596)) ;
#77112=CARTESIAN_POINT('Ctrl Pts',(62.0837422493721,214.400192437673,26.3713203435596)) ;
#77113=CARTESIAN_POINT('Ctrl Pts',(62.061600704641,214.509619645667,26.3713203435596)) ;
#77114=CARTESIAN_POINT('Ctrl Pts',(62.155519600537,214.1870937114,26.3713203435596)) ;
#77115=CARTESIAN_POINT('Ctrl Pts',(62.1326307024359,214.2963037009,26.3713203435596)) ;
#77116=CARTESIAN_POINT('Ctrl Pts',(62.1101230239711,214.405593582675,26.3713203435596)) ;
#77117=CARTESIAN_POINT('Ctrl Pts',(62.0879937736325,214.51496002973,26.3713203435596)) ;
#77118=CARTESIAN_POINT('',(62.0879937736325,214.51496002973,26.3713203435596)) ;
#77119=CARTESIAN_POINT('Origin',(158.549722376545,280.559557010502,26.3713203435596)) ;
#77120=CARTESIAN_POINT('',(61.9703773266191,214.491161471119,26.4913203435596)) ;
#77121=CARTESIAN_POINT('Origin',(62.0879937736325,214.51496002973,26.4913203435596)) ;
#77122=CARTESIAN_POINT('Origin',(168.040182093702,286.993621933611,26.4913203435596)) ;
#77123=CARTESIAN_POINT('Ctrl Pts',(61.9703773266184,214.491161471123,26.4913203435596)) ;
#77124=CARTESIAN_POINT('Ctrl Pts',(61.8515958146182,215.078199520065,26.4913203435596)) ;
#77125=CARTESIAN_POINT('Ctrl Pts',(61.7916108526749,215.677118713722,26.4913203435596)) ;
#77126=CARTESIAN_POINT('Ctrl Pts',(61.7916108526749,216.276053366666,26.4913203435596)) ;
#77127=CARTESIAN_POINT('Ctrl Pts',(61.9703773266184,214.491161471123,26.4554164275186)) ;
#77128=CARTESIAN_POINT('Ctrl Pts',(61.8515907531908,215.078224534483,26.4554164275186)) ;
#77129=CARTESIAN_POINT('Ctrl Pts',(61.7916108526749,215.677093192374,26.4554164275186)) ;
#77130=CARTESIAN_POINT('Ctrl Pts',(61.7916108526749,216.276053366666,26.4554164275186)) ;
#77131=CARTESIAN_POINT('Ctrl Pts',(61.9999367861991,214.497142543916,26.3932839420772)) ;
#77132=CARTESIAN_POINT('Ctrl Pts',(61.8815544712344,215.082207694509,26.3932839420772)) ;
#77133=CARTESIAN_POINT('Ctrl Pts',(61.8217693486993,215.67913159379,26.3932839420772)) ;
#77134=CARTESIAN_POINT('Ctrl Pts',(61.8217693486993,216.276053366666,26.3932839420772)) ;
#77135=CARTESIAN_POINT('Ctrl Pts',(62.061600704641,214.509619645667,26.3713203435596)) ;
#77136=CARTESIAN_POINT('Ctrl Pts',(61.9440482796633,215.090583341491,26.3713203435596)) ;
#77137=CARTESIAN_POINT('Ctrl Pts',(61.8846829156441,215.68331616648,26.3713203435596)) ;
#77138=CARTESIAN_POINT('Ctrl Pts',(61.8846829156441,216.276053366667,26.3713203435596)) ;
#77139=CARTESIAN_POINT('Ctrl Pts',(62.0879937736325,214.51496002973,26.3713203435596)) ;
#77140=CARTESIAN_POINT('Ctrl Pts',(61.9707960151257,215.094170904685,26.3713203435596)) ;
#77141=CARTESIAN_POINT('Ctrl Pts',(61.9116108526749,215.685104509095,26.3713203435596)) ;
#77142=CARTESIAN_POINT('Ctrl Pts',(61.9116108526749,216.276053366667,26.3713203435596)) ;
#77143=CARTESIAN_POINT('',(61.9116108526749,216.276053366667,26.3713203435596)) ;
#77144=CARTESIAN_POINT('',(61.7916108526749,216.276053366666,26.4913203435596)) ;
#77145=CARTESIAN_POINT('Origin',(61.9116108526749,216.276053366667,26.4913203435596)) ;
#77146=CARTESIAN_POINT('Origin',(70.7990562975695,216.276799067812,26.4913203435596)) ;
#77147=CARTESIAN_POINT('Origin',(70.798957024977,216.27678912513,26.3713203435596)) ;
#77148=CARTESIAN_POINT('Origin',(61.9116108526749,216.02810186684,26.4913203435596)) ;
#77149=CARTESIAN_POINT('',(61.7916108526749,217.432246240363,26.4913203435596)) ;
#77150=CARTESIAN_POINT('',(61.9116108526749,217.332165092393,26.3713203435596)) ;
#77151=CARTESIAN_POINT('Ctrl Pts',(61.7916108526749,217.432246240364,26.4913203435596)) ;
#77152=CARTESIAN_POINT('Ctrl Pts',(61.7916108526749,217.432246240364,26.4763546071157)) ;
#77153=CARTESIAN_POINT('Ctrl Pts',(61.7945994481497,217.429633269658,26.4608211829996)) ;
#77154=CARTESIAN_POINT('Ctrl Pts',(61.8056861138382,217.420035117846,26.4329402504268)) ;
#77155=CARTESIAN_POINT('Ctrl Pts',(61.8137971189369,217.413045531713,26.420599403965)) ;
#77156=CARTESIAN_POINT('Ctrl Pts',(61.8340451542424,217.395799093869,26.3981511688094)) ;
#77157=CARTESIAN_POINT('Ctrl Pts',(61.8484542267829,217.383662220691,26.3878996607103)) ;
#77158=CARTESIAN_POINT('Ctrl Pts',(61.879478171071,217.358033658104,26.3744685762533)) ;
#77159=CARTESIAN_POINT('Ctrl Pts',(61.8961032700049,217.344537933513,26.3713203435596)) ;
#77160=CARTESIAN_POINT('Ctrl Pts',(61.9116108526749,217.332165092393,26.3713203435596)) ;
#77161=CARTESIAN_POINT('',(61.7916108526749,216.02810186684,26.4913203435596)) ;
#77162=CARTESIAN_POINT('',(61.9116108526749,216.02810186684,26.3713203435596)) ;
#77163=CARTESIAN_POINT('Origin',(68.8498979833486,219.885565182264,30.2513203435596)) ;
#77164=CARTESIAN_POINT('',(68.8350389209693,219.766488701525,30.2513203435596)) ;
#77165=CARTESIAN_POINT('Ctrl Pts',(62.0380714133749,214.162478201405,30.2513203435596)) ;
#77166=CARTESIAN_POINT('Ctrl Pts',(62.0151257340927,214.271959111425,30.2513203435596)) ;
#77167=CARTESIAN_POINT('Ctrl Pts',(61.9925619554488,214.381521334322,30.2513203435596)) ;
#77168=CARTESIAN_POINT('Ctrl Pts',(61.9703773266184,214.491161471123,30.2513203435596)) ;
#77169=CARTESIAN_POINT('Ctrl Pts',(62.0380714133749,214.162478201405,30.2872242596007)) ;
#77170=CARTESIAN_POINT('Ctrl Pts',(62.0151259171648,214.271958237932,30.2872242596007)) ;
#77171=CARTESIAN_POINT('Ctrl Pts',(61.9925617799923,214.381522201457,30.2872242596007)) ;
#77172=CARTESIAN_POINT('Ctrl Pts',(61.9703773266184,214.491161471123,30.2872242596007)) ;
#77173=CARTESIAN_POINT('Ctrl Pts',(62.0085542139792,214.156291806073,30.3493567119227)) ;
#77174=CARTESIAN_POINT('Ctrl Pts',(61.9855940957225,214.265841608892,30.3493567119227)) ;
#77175=CARTESIAN_POINT('Ctrl Pts',(61.9630163071413,214.375471864732,30.3493567119227)) ;
#77176=CARTESIAN_POINT('Ctrl Pts',(61.9408178399833,214.485180392856,30.3493567119227)) ;
#77177=CARTESIAN_POINT('Ctrl Pts',(61.9469785377818,214.143386398936,30.3713203435596)) ;
#77178=CARTESIAN_POINT('Ctrl Pts',(61.9239884023675,214.253079422868,30.3713203435596)) ;
#77179=CARTESIAN_POINT('Ctrl Pts',(61.9013811842277,214.362852589857,30.3713203435596)) ;
#77180=CARTESIAN_POINT('Ctrl Pts',(61.8791539485958,214.472703296579,30.3713203435596)) ;
#77181=CARTESIAN_POINT('Ctrl Pts',(61.9206232262128,214.13786269141,30.3713203435596)) ;
#77182=CARTESIAN_POINT('Ctrl Pts',(61.8976202624965,214.247616923126,30.3713203435596)) ;
#77183=CARTESIAN_POINT('Ctrl Pts',(61.8750004098937,214.357451443545,30.3713203435596)) ;
#77184=CARTESIAN_POINT('Ctrl Pts',(61.8527608796043,214.467362912516,30.3713203435596)) ;
#77185=CARTESIAN_POINT('',(61.9703773266191,214.491161471119,30.2513203435596)) ;
#77186=CARTESIAN_POINT('Origin',(149.370337688321,274.199128996313,30.2513203435596)) ;
#77187=CARTESIAN_POINT('Origin',(61.8527608796043,214.467362912516,30.2513203435596)) ;
#77188=CARTESIAN_POINT('Ctrl Pts',(61.6716108526749,216.276053366666,30.3713203435596)) ;
#77189=CARTESIAN_POINT('Ctrl Pts',(61.6716108526749,215.669132918349,30.3713203435596)) ;
#77190=CARTESIAN_POINT('Ctrl Pts',(61.7323956141108,215.062228135443,30.3713203435596)) ;
#77191=CARTESIAN_POINT('Ctrl Pts',(61.8527608796043,214.467362912515,30.3713203435596)) ;
#77192=CARTESIAN_POINT('Ctrl Pts',(61.7075147687159,216.276053366666,30.3713203435596)) ;
#77193=CARTESIAN_POINT('Ctrl Pts',(61.7075147687159,215.671532615249,30.3713203435596)) ;
#77194=CARTESIAN_POINT('Ctrl Pts',(61.7680622838269,215.066996615668,30.3713203435596)) ;
#77195=CARTESIAN_POINT('Ctrl Pts',(61.8879516382597,214.4744834246,30.3713203435596)) ;
#77196=CARTESIAN_POINT('Ctrl Pts',(61.7696471970384,216.276053366666,30.3411617999306)) ;
#77197=CARTESIAN_POINT('Ctrl Pts',(61.7696471970384,215.6756545881,30.3411617999306)) ;
#77198=CARTESIAN_POINT('Ctrl Pts',(61.8297780544614,215.075278702629,30.3411617999306)) ;
#77199=CARTESIAN_POINT('Ctrl Pts',(61.9488499337901,214.486805609907,30.3411617999306)) ;
#77200=CARTESIAN_POINT('Ctrl Pts',(61.7916108526749,216.276053366666,30.2782482805904)) ;
#77201=CARTESIAN_POINT('Ctrl Pts',(61.7916108526749,215.677125204134,30.2782482805904)) ;
#77202=CARTESIAN_POINT('Ctrl Pts',(61.8515971018053,215.078193158571,30.2782482805904)) ;
#77203=CARTESIAN_POINT('Ctrl Pts',(61.9703773266184,214.491161471123,30.2782482805904)) ;
#77204=CARTESIAN_POINT('Ctrl Pts',(61.7916108526749,216.276053366666,30.2513203435596)) ;
#77205=CARTESIAN_POINT('Ctrl Pts',(61.7916108526749,215.677118713722,30.2513203435596)) ;
#77206=CARTESIAN_POINT('Ctrl Pts',(61.8515958146183,215.078199520064,30.2513203435596)) ;
#77207=CARTESIAN_POINT('Ctrl Pts',(61.9703773266184,214.491161471123,30.2513203435596)) ;
#77208=CARTESIAN_POINT('',(61.7916108526749,216.276053366666,30.2513203435596)) ;
#77209=CARTESIAN_POINT('Origin',(70.7990562975712,216.276799067812,30.2513203435596)) ;
#77210=CARTESIAN_POINT('Origin',(61.6716108526749,216.276053366666,30.2513203435596)) ;
#77211=CARTESIAN_POINT('Origin',(61.6716108526749,216.520093569003,30.2513203435596)) ;
#77212=CARTESIAN_POINT('',(61.7916108526749,216.520093569003,30.2513203435596)) ;
#77213=CARTESIAN_POINT('Ctrl Pts',(69.0490142989097,219.47364875508,26.3713203435596)) ;
#77214=CARTESIAN_POINT('Ctrl Pts',(69.0516144229285,219.507855459592,26.3713203435596)) ;
#77215=CARTESIAN_POINT('Ctrl Pts',(69.0542647955834,219.542058391199,26.3713203435596)) ;
#77216=CARTESIAN_POINT('Ctrl Pts',(69.0569653274897,219.576257334544,26.3713203435596)) ;
#77217=CARTESIAN_POINT('Ctrl Pts',(69.084814938696,219.470927472667,26.3713203435596)) ;
#77218=CARTESIAN_POINT('Ctrl Pts',(69.0874123863672,219.505098967692,26.3713203435596)) ;
#77219=CARTESIAN_POINT('Ctrl Pts',(69.0900600681774,219.539267174567,26.3713203435596)) ;
#77220=CARTESIAN_POINT('Ctrl Pts',(69.0927578243876,219.573430967106,26.3713203435596)) ;
#77221=CARTESIAN_POINT('Ctrl Pts',(69.1467685461534,219.46621824782,26.4014789701773)) ;
#77222=CARTESIAN_POINT('Ctrl Pts',(69.1493613966472,219.500329263312,26.4014789701773)) ;
#77223=CARTESIAN_POINT('Ctrl Pts',(69.1520043520586,219.53443647706,26.4014789701773)) ;
#77224=CARTESIAN_POINT('Ctrl Pts',(69.1546973404401,219.568539890862,26.4014789701773)) ;
#77225=CARTESIAN_POINT('Ctrl Pts',(69.1686691234544,219.464553538581,26.4643924065289)) ;
#77226=CARTESIAN_POINT('Ctrl Pts',(69.1712603337912,219.498642976499,26.4643924065289)) ;
#77227=CARTESIAN_POINT('Ctrl Pts',(69.1739016490944,219.53272902503,26.4643924065289)) ;
#77228=CARTESIAN_POINT('Ctrl Pts',(69.1765929364347,219.566810897221,26.4643924065289)) ;
#77229=CARTESIAN_POINT('Ctrl Pts',(69.1686691234544,219.464553538581,26.4913203435596)) ;
#77230=CARTESIAN_POINT('Ctrl Pts',(69.1712603410299,219.49864307173,26.4913203435596)) ;
#77231=CARTESIAN_POINT('Ctrl Pts',(69.173901641587,219.532728929959,26.4913203435596)) ;
#77232=CARTESIAN_POINT('Ctrl Pts',(69.1765929364347,219.566810897221,26.4913203435596)) ;
#77233=CARTESIAN_POINT('',(69.05696532749,219.576257334543,26.3713203435596)) ;
#77234=CARTESIAN_POINT('Ctrl Pts',(69.1686691234543,219.464553538579,26.4913203435596)) ;
#77235=CARTESIAN_POINT('Ctrl Pts',(69.1686691234543,219.464553538579,26.4825755545765)) ;
#77236=CARTESIAN_POINT('Ctrl Pts',(69.1677442553345,219.465478406699,26.4739056649623)) ;
#77237=CARTESIAN_POINT('Ctrl Pts',(69.1637138918045,219.469508770229,26.4544411500671)) ;
#77238=CARTESIAN_POINT('Ctrl Pts',(69.1600464491366,219.473176212897,26.4440224457763)) ;
#77239=CARTESIAN_POINT('Ctrl Pts',(69.1487510229112,219.484471639122,26.4213114813416)) ;
#77240=CARTESIAN_POINT('Ctrl Pts',(69.1403360239462,219.492886638031,26.4103700658404)) ;
#77241=CARTESIAN_POINT('Ctrl Pts',(69.1203185307192,219.512904131258,26.3916682055822)) ;
#77242=CARTESIAN_POINT('Ctrl Pts',(69.1085784082693,219.524644253764,26.3843267857594)) ;
#77243=CARTESIAN_POINT('Ctrl Pts',(69.0837605938726,219.549462068161,26.37407374451)) ;
#77244=CARTESIAN_POINT('Ctrl Pts',(69.0702970781629,219.562925583871,26.3713203435597)) ;
#77245=CARTESIAN_POINT('Ctrl Pts',(69.0569653274903,219.576257334543,26.3713203435596)) ;
#77246=CARTESIAN_POINT('Origin',(88.0257792156962,221.138894496662,26.3713203435596)) ;
#77247=CARTESIAN_POINT('Origin',(65.5243724680055,216.635300802115,26.3713203435596)) ;
#77248=CARTESIAN_POINT('',(68.8712529610467,219.761969700987,26.3713203435596)) ;
#77249=CARTESIAN_POINT('',(70.8292893218811,217.803933340152,26.3713203435596)) ;
#77250=CARTESIAN_POINT('',(67.7485452644419,219.902067758924,26.3713203435596)) ;
#77251=CARTESIAN_POINT('',(66.8542082278115,220.013668385118,26.3713203435596)) ;
#77252=CARTESIAN_POINT('Origin',(64.1568347953872,220.146231446812,26.3713203435596)) ;
#77253=CARTESIAN_POINT('Ctrl Pts',(69.087238483681,215.789690773497,23.8713203435596)) ;
#77254=CARTESIAN_POINT('Ctrl Pts',(69.087238483681,215.789690773497,31.6713203435596)) ;
#77255=CARTESIAN_POINT('Ctrl Pts',(69.1136171491181,214.983615131093,23.8713203435596)) ;
#77256=CARTESIAN_POINT('Ctrl Pts',(69.1136171491181,214.983615131093,31.6713203435596)) ;
#77257=CARTESIAN_POINT('Ctrl Pts',(69.1697039478106,214.179248099427,23.8713203435596)) ;
#77258=CARTESIAN_POINT('Ctrl Pts',(69.1697039478106,214.179248099427,31.6713203435596)) ;
#77259=CARTESIAN_POINT('Ctrl Pts',(69.2569276623894,213.37702429324,23.8713203435596)) ;
#77260=CARTESIAN_POINT('Ctrl Pts',(69.2569276623894,213.37702429324,31.6713203435596)) ;
#77261=CARTESIAN_POINT('',(69.087238483681,215.789690773497,23.8713203435596)) ;
#77262=CARTESIAN_POINT('Ctrl Pts',(69.1686691234544,219.464553538579,23.8713203435596)) ;
#77263=CARTESIAN_POINT('Ctrl Pts',(69.1686691234544,219.464553538579,31.6713203435596)) ;
#77264=CARTESIAN_POINT('Ctrl Pts',(69.0753247917718,218.236534433073,23.8713203435596)) ;
#77265=CARTESIAN_POINT('Ctrl Pts',(69.0753247917718,218.236534433073,31.6713203435596)) ;
#77266=CARTESIAN_POINT('Ctrl Pts',(69.0472671147723,217.011130390261,23.8713203435596)) ;
#77267=CARTESIAN_POINT('Ctrl Pts',(69.0472671147723,217.011130390261,31.6713203435596)) ;
#77268=CARTESIAN_POINT('Ctrl Pts',(69.0872384835382,215.789690777862,23.8713203435596)) ;
#77269=CARTESIAN_POINT('Ctrl Pts',(69.0872384835382,215.789690777862,31.6713203435596)) ;
#77270=CARTESIAN_POINT('',(69.1686691234544,219.464553538579,23.8713203435596)) ;
#77271=CARTESIAN_POINT('Origin',(104.054869375424,216.812621949209,23.8713203435596)) ;
#77272=CARTESIAN_POINT('',(69.189219381737,219.722291984193,23.8713203435596)) ;
#77273=CARTESIAN_POINT('',(69.1892193809281,219.722291984294,23.8713203435596)) ;
#77274=CARTESIAN_POINT('',(69.1686691229769,219.464553539057,23.8713203435596)) ;
#77275=CARTESIAN_POINT('Origin',(180.960510687652,228.725125033291,23.8713203435596)) ;
#77276=CARTESIAN_POINT('',(69.1686691234544,219.464553538579,23.8713203435596)) ;
#77277=CARTESIAN_POINT('Origin',(69.2569276623894,213.37702429324,23.8713203435596)) ;
#77278=CARTESIAN_POINT('Ctrl Pts',(62.8216952668539,212.37422947071,23.3713203435596)) ;
#77279=CARTESIAN_POINT('Ctrl Pts',(62.7643918956731,212.379793292255,23.3713203435596)) ;
#77280=CARTESIAN_POINT('Ctrl Pts',(62.6452781621069,212.331202353327,23.3713203435596)) ;
#77281=CARTESIAN_POINT('Ctrl Pts',(62.6156344352299,212.206021423155,23.3713203435596)) ;
#77282=CARTESIAN_POINT('Ctrl Pts',(62.629967133072,212.150261166418,23.3713203435596)) ;
#77283=CARTESIAN_POINT('Ctrl Pts',(62.8251650099645,212.409965336026,23.3713203435596)) ;
#77284=CARTESIAN_POINT('Ctrl Pts',(62.7563820289917,212.416643760411,23.3713203435596)) ;
#77285=CARTESIAN_POINT('Ctrl Pts',(62.6134890558422,212.358415343631,23.3713203435596)) ;
#77286=CARTESIAN_POINT('Ctrl Pts',(62.5779896202957,212.208253658832,23.3713203435596)) ;
#77287=CARTESIAN_POINT('Ctrl Pts',(62.5951935938603,212.141322925104,23.3713203435596)) ;
#77288=CARTESIAN_POINT('Ctrl Pts',(62.8311694823153,212.471807094442,23.4014787656397)) ;
#77289=CARTESIAN_POINT('Ctrl Pts',(62.7426679110788,212.480400078392,23.4014787656397)) ;
#77290=CARTESIAN_POINT('Ctrl Pts',(62.5586840514308,212.405331040411,23.4014787656397)) ;
#77291=CARTESIAN_POINT('Ctrl Pts',(62.5128811834681,212.211973412379,23.4014787656397)) ;
#77292=CARTESIAN_POINT('Ctrl Pts',(62.5350171634802,212.125855087538,23.4014787656397)) ;
#77293=CARTESIAN_POINT('Ctrl Pts',(62.8332920289675,212.493667802533,23.4643924065289)) ;
#77294=CARTESIAN_POINT('Ctrl Pts',(62.7377553616651,212.502943853085,23.4643924065289)) ;
#77295=CARTESIAN_POINT('Ctrl Pts',(62.539219886079,212.421993293736,23.4643924065289)) ;
#77296=CARTESIAN_POINT('Ctrl Pts',(62.489849543713,212.21335126917,23.4643924065289)) ;
#77297=CARTESIAN_POINT('Ctrl Pts',(62.513745139331,212.120387295379,23.4643924065289)) ;
#77298=CARTESIAN_POINT('Ctrl Pts',(62.8332920289675,212.493667802533,23.4913203435596)) ;
#77299=CARTESIAN_POINT('Ctrl Pts',(62.7377864103328,212.502940838441,23.4913203435596)) ;
#77300=CARTESIAN_POINT('Ctrl Pts',(62.539263521056,212.421955940227,23.4913203435596)) ;
#77301=CARTESIAN_POINT('Ctrl Pts',(62.4898573095942,212.213321056607,23.4913203435596)) ;
#77302=CARTESIAN_POINT('Ctrl Pts',(62.513745139331,212.120387295379,23.4913203435596)) ;
#77303=CARTESIAN_POINT('',(62.629967133072,212.150261166418,23.3713203435596)) ;
#77304=CARTESIAN_POINT('Origin',(62.629967133072,212.150261166418,23.4913203435596)) ;
#77305=CARTESIAN_POINT('',(62.8216952668539,212.37422947071,23.3713203435596)) ;
#77306=CARTESIAN_POINT('Ctrl Pts',(62.629967133072,212.150261166418,23.3713203435596)) ;
#77307=CARTESIAN_POINT('Ctrl Pts',(62.6156344352299,212.206021423155,23.3713203435596)) ;
#77308=CARTESIAN_POINT('Ctrl Pts',(62.6452781621069,212.331202353327,23.3713203435596)) ;
#77309=CARTESIAN_POINT('Ctrl Pts',(62.7643918956731,212.379793292255,23.3713203435596)) ;
#77310=CARTESIAN_POINT('Ctrl Pts',(62.8216952668539,212.37422947071,23.3713203435596)) ;
#77311=CARTESIAN_POINT('Origin',(62.8216952668539,212.37422947071,23.4913203435596)) ;
#77312=CARTESIAN_POINT('Ctrl Pts',(66.5773376779735,202.200615492168,23.4913203435596)) ;
#77313=CARTESIAN_POINT('Ctrl Pts',(64.7210140334605,205.27084597784,23.4913203435596)) ;
#77314=CARTESIAN_POINT('Ctrl Pts',(63.4059506185125,208.649330615767,23.4913203435596)) ;
#77315=CARTESIAN_POINT('Ctrl Pts',(62.513745139331,212.120387295379,23.4913203435596)) ;
#77316=CARTESIAN_POINT('Ctrl Pts',(66.5773376779735,202.200615492168,23.4554164275186)) ;
#77317=CARTESIAN_POINT('Ctrl Pts',(64.7209918030059,205.27088274547,23.4554164275186)) ;
#77318=CARTESIAN_POINT('Ctrl Pts',(63.4059582099283,208.649301081949,23.4554164275186)) ;
#77319=CARTESIAN_POINT('Ctrl Pts',(62.513745139331,212.120387295379,23.4554164275186)) ;
#77320=CARTESIAN_POINT('Ctrl Pts',(66.6031455496054,202.216219454981,23.3932838428366)) ;
#77321=CARTESIAN_POINT('Ctrl Pts',(64.748575230952,205.283550061356,23.3932838428366)) ;
#77322=CARTESIAN_POINT('Ctrl Pts',(63.4345608045287,208.659167865758,23.3932838428366)) ;
#77323=CARTESIAN_POINT('Ctrl Pts',(62.542954063693,212.127895199963,23.3932838428366)) ;
#77324=CARTESIAN_POINT('Ctrl Pts',(66.6569835077658,202.24877097682,23.3713203435596)) ;
#77325=CARTESIAN_POINT('Ctrl Pts',(64.8060581750343,205.310073029429,23.3713203435596)) ;
#77326=CARTESIAN_POINT('Ctrl Pts',(63.4942490034471,208.679672623132,23.3713203435596)) ;
#77327=CARTESIAN_POINT('Ctrl Pts',(62.6038869786632,212.143557485433,23.3713203435596)) ;
#77328=CARTESIAN_POINT('Ctrl Pts',(66.6800269197305,202.262703491229,23.3713203435596)) ;
#77329=CARTESIAN_POINT('Ctrl Pts',(64.8306593287648,205.32142914706,23.3713203435596)) ;
#77330=CARTESIAN_POINT('Ctrl Pts',(63.5197972089754,208.688445810254,23.3713203435596)) ;
#77331=CARTESIAN_POINT('Ctrl Pts',(62.629967133072,212.150261166418,23.3713203435596)) ;
#77332=CARTESIAN_POINT('',(66.6800269197305,202.262703491229,23.3713203435596)) ;
#77333=CARTESIAN_POINT('Origin',(66.6800269197305,202.262703491229,23.4913203435596)) ;
#77334=CARTESIAN_POINT('Origin',(124.488490460381,267.59388982529,23.3713203435596)) ;
#77335=CARTESIAN_POINT('Ctrl Pts',(66.6800269197305,202.262703491229,23.3713203435596)) ;
#77336=CARTESIAN_POINT('Ctrl Pts',(66.7119076863592,202.209974915638,23.3713203435596)) ;
#77337=CARTESIAN_POINT('Ctrl Pts',(66.772443528576,202.17583548982,23.3713203435596)) ;
#77338=CARTESIAN_POINT('Ctrl Pts',(66.8340607823661,202.17583548982,23.3713203435596)) ;
#77339=CARTESIAN_POINT('Ctrl Pts',(66.6493023704442,202.24412680535,23.3713203435596)) ;
#77340=CARTESIAN_POINT('Ctrl Pts',(66.687569825207,202.1808350908,23.3713203435596)) ;
#77341=CARTESIAN_POINT('Ctrl Pts',(66.7600997167655,202.139931573779,23.3713203435596)) ;
#77342=CARTESIAN_POINT('Ctrl Pts',(66.8340607823661,202.139931573779,23.3713203435596)) ;
#77343=CARTESIAN_POINT('Ctrl Pts',(66.5961327241498,202.211979358425,23.4014786793986)) ;
#77344=CARTESIAN_POINT('Ctrl Pts',(66.6453706290186,202.13054328071,23.4014786793986)) ;
#77345=CARTESIAN_POINT('Ctrl Pts',(66.7388966818371,202.077798896138,23.4014786793986)) ;
#77346=CARTESIAN_POINT('Ctrl Pts',(66.8340607823661,202.077798896138,23.4014786793986)) ;
#77347=CARTESIAN_POINT('Ctrl Pts',(66.5773376779735,202.200615492168,23.4643924065289)) ;
#77348=CARTESIAN_POINT('Ctrl Pts',(66.6304895629671,202.112705962943,23.4643924065289)) ;
#77349=CARTESIAN_POINT('Ctrl Pts',(66.7313319733253,202.05583548982,23.4643924065289)) ;
#77350=CARTESIAN_POINT('Ctrl Pts',(66.8340607823661,202.05583548982,23.4643924065289)) ;
#77351=CARTESIAN_POINT('Ctrl Pts',(66.5773376779735,202.200615492168,23.4913203435596)) ;
#77352=CARTESIAN_POINT('Ctrl Pts',(66.6304722890212,202.112734532851,23.4913203435596)) ;
#77353=CARTESIAN_POINT('Ctrl Pts',(66.7313653593827,202.05583548982,23.4913203435596)) ;
#77354=CARTESIAN_POINT('Ctrl Pts',(66.8340607823661,202.05583548982,23.4913203435596)) ;
#77355=CARTESIAN_POINT('',(66.8340607823661,202.17583548982,23.3713203435596)) ;
#77356=CARTESIAN_POINT('Origin',(66.8340607823661,202.17583548982,23.4913203435596)) ;
#77357=CARTESIAN_POINT('Origin',(66.8127335805022,202.318018212697,23.3713203435596)) ;
#77358=CARTESIAN_POINT('Origin',(70.2085194795435,202.17583548982,23.4913203435596)) ;
#77359=CARTESIAN_POINT('',(72.3111547045756,202.17583548982,23.3713203435596)) ;
#77360=CARTESIAN_POINT('Origin',(72.3111547045756,202.17583548982,23.4913203435596)) ;
#77361=CARTESIAN_POINT('',(70.2085194795435,202.17583548982,23.3713203435596)) ;
#77362=CARTESIAN_POINT('Ctrl Pts',(72.3111547045756,202.17583548982,23.3713203435596)) ;
#77363=CARTESIAN_POINT('Ctrl Pts',(72.363829615569,202.17583548982,23.3713203435596)) ;
#77364=CARTESIAN_POINT('Ctrl Pts',(72.4506823622179,202.217096002582,23.3713203435596)) ;
#77365=CARTESIAN_POINT('Ctrl Pts',(72.5005099444522,202.335617710977,23.3713203435596)) ;
#77366=CARTESIAN_POINT('Ctrl Pts',(72.4871463781874,202.40741171428,23.3713203435596)) ;
#77367=CARTESIAN_POINT('Ctrl Pts',(72.4710003713497,202.438596367132,23.3713203435596)) ;
#77368=CARTESIAN_POINT('Ctrl Pts',(72.3111547045756,202.139931573779,23.3713203435596)) ;
#77369=CARTESIAN_POINT('Ctrl Pts',(72.3743820038766,202.139931573779,23.3713203435596)) ;
#77370=CARTESIAN_POINT('Ctrl Pts',(72.4785527184376,202.189324234858,23.3713203435596)) ;
#77371=CARTESIAN_POINT('Ctrl Pts',(72.5383561337277,202.331579334424,23.3713203435596)) ;
#77372=CARTESIAN_POINT('Ctrl Pts',(72.5222647226805,202.417672476653,23.3713203435596)) ;
#77373=CARTESIAN_POINT('Ctrl Pts',(72.5028841791241,202.455104364857,23.3713203435596)) ;
#77374=CARTESIAN_POINT('Ctrl Pts',(72.3111547045756,202.077798995588,23.4014787622833)) ;
#77375=CARTESIAN_POINT('Ctrl Pts',(72.3925079005849,202.077798995588,23.4014787622833)) ;
#77376=CARTESIAN_POINT('Ctrl Pts',(72.5266662486247,202.141555501501,23.4014787622833)) ;
#77377=CARTESIAN_POINT('Ctrl Pts',(72.6036233984803,202.324607505548,23.4014787622833)) ;
#77378=CARTESIAN_POINT('Ctrl Pts',(72.5829963900795,202.435509046935,23.4014787622833)) ;
#77379=CARTESIAN_POINT('Ctrl Pts',(72.5580598646207,202.483671846417,23.4014787622833)) ;
#77380=CARTESIAN_POINT('Ctrl Pts',(72.3111547045756,202.05583548982,23.4643924065289)) ;
#77381=CARTESIAN_POINT('Ctrl Pts',(72.3989747637286,202.05583548982,23.4643924065289)) ;
#77382=CARTESIAN_POINT('Ctrl Pts',(72.5437254422553,202.124541615164,23.4643924065289)) ;
#77383=CARTESIAN_POINT('Ctrl Pts',(72.6267945558901,202.32213567271,23.4643924065289)) ;
#77384=CARTESIAN_POINT('Ctrl Pts',(72.6044829089811,202.44177896715,23.4643924065289)) ;
#77385=CARTESIAN_POINT('Ctrl Pts',(72.5775641491992,202.49377028534,23.4643924065289)) ;
#77386=CARTESIAN_POINT('Ctrl Pts',(72.3111547045756,202.05583548982,23.4913203435596)) ;
#77387=CARTESIAN_POINT('Ctrl Pts',(72.398946222898,202.05583548982,23.4913203435596)) ;
#77388=CARTESIAN_POINT('Ctrl Pts',(72.5437008006462,202.12460301109,23.4913203435596)) ;
#77389=CARTESIAN_POINT('Ctrl Pts',(72.6267467710367,202.322139191748,23.4913203435596)) ;
#77390=CARTESIAN_POINT('Ctrl Pts',(72.6044741605953,202.441795863921,23.4913203435596)) ;
#77391=CARTESIAN_POINT('Ctrl Pts',(72.5775641491992,202.49377028534,23.4913203435596)) ;
#77392=CARTESIAN_POINT('',(72.5775641491992,202.49377028534,23.4913203435596)) ;
#77393=CARTESIAN_POINT('',(72.4710003713497,202.438596367132,23.3713203435596)) ;
#77394=CARTESIAN_POINT('Origin',(72.4710003713497,202.438596367132,23.4913203435596)) ;
#77395=CARTESIAN_POINT('Ctrl Pts',(72.4710003713497,202.438596367132,23.3713203435596)) ;
#77396=CARTESIAN_POINT('Ctrl Pts',(72.4871463781874,202.40741171428,23.3713203435596)) ;
#77397=CARTESIAN_POINT('Ctrl Pts',(72.5005099444522,202.335617710977,23.3713203435596)) ;
#77398=CARTESIAN_POINT('Ctrl Pts',(72.4506823622179,202.217096002582,23.3713203435596)) ;
#77399=CARTESIAN_POINT('Ctrl Pts',(72.363829615569,202.17583548982,23.3713203435596)) ;
#77400=CARTESIAN_POINT('Ctrl Pts',(72.3111547045756,202.17583548982,23.3713203435596)) ;
#77401=CARTESIAN_POINT('Ctrl Pts',(72.3111547045756,202.05583548982,23.4913203435596)) ;
#77402=CARTESIAN_POINT('Ctrl Pts',(72.398946222898,202.05583548982,23.4913203435596)) ;
#77403=CARTESIAN_POINT('Ctrl Pts',(72.5437008006462,202.12460301109,23.4913203435596)) ;
#77404=CARTESIAN_POINT('Ctrl Pts',(72.6267467710367,202.322139191748,23.4913203435596)) ;
#77405=CARTESIAN_POINT('Ctrl Pts',(72.6044741605953,202.441795863921,23.4913203435596)) ;
#77406=CARTESIAN_POINT('Ctrl Pts',(72.5775641491992,202.49377028534,23.4913203435596)) ;
#77407=CARTESIAN_POINT('Ctrl Pts',(69.4984736650468,211.623322295552,23.4913203435596)) ;
#77408=CARTESIAN_POINT('Ctrl Pts',(70.0303479865131,208.443107464909,23.4913203435596)) ;
#77409=CARTESIAN_POINT('Ctrl Pts',(71.0942570395756,205.358653085868,23.4913203435596)) ;
#77410=CARTESIAN_POINT('Ctrl Pts',(72.5775641491992,202.49377028534,23.4913203435596)) ;
#77411=CARTESIAN_POINT('Ctrl Pts',(69.4984736650468,211.623322295552,23.4554164275186)) ;
#77412=CARTESIAN_POINT('Ctrl Pts',(70.0303412850924,208.443147534446,23.4554164275186)) ;
#77413=CARTESIAN_POINT('Ctrl Pts',(71.0942731909361,205.358621890875,23.4554164275186)) ;
#77414=CARTESIAN_POINT('Ctrl Pts',(72.5775641491992,202.49377028534,23.4554164275186)) ;
#77415=CARTESIAN_POINT('Ctrl Pts',(69.4687283004056,211.618347538663,23.3932839428985)) ;
#77416=CARTESIAN_POINT('Ctrl Pts',(70.0011311659099,208.434972405821,23.3932839428985)) ;
#77417=CARTESIAN_POINT('Ctrl Pts',(71.0662014800548,205.347247095261,23.3932839428985)) ;
#77418=CARTESIAN_POINT('Ctrl Pts',(72.5507824546696,202.479903931751,23.3932839428985)) ;
#77419=CARTESIAN_POINT('Ctrl Pts',(69.4066765679416,211.607969710479,23.3713203435596)) ;
#77420=CARTESIAN_POINT('Ctrl Pts',(69.9401782226795,208.418024631175,23.3713203435596)) ;
#77421=CARTESIAN_POINT('Ctrl Pts',(71.0076840169658,205.323435373038,23.3713203435596)) ;
#77422=CARTESIAN_POINT('Ctrl Pts',(72.4949132271805,202.450977365426,23.3713203435596)) ;
#77423=CARTESIAN_POINT('Ctrl Pts',(69.3801175085246,211.603527846499,23.3713203435596)) ;
#77424=CARTESIAN_POINT('Ctrl Pts',(69.9140887480339,208.410774997776,23.3713203435596)) ;
#77425=CARTESIAN_POINT('Ctrl Pts',(70.9826393962153,205.313240283402,23.3713203435596)) ;
#77426=CARTESIAN_POINT('Ctrl Pts',(72.4710003713498,202.438596367132,23.3713203435596)) ;
#77427=CARTESIAN_POINT('',(69.4984736650468,211.623322295552,23.4913203435596)) ;
#77428=CARTESIAN_POINT('Origin',(96.3696349527109,211.612385354758,23.4913203435596)) ;
#77429=CARTESIAN_POINT('',(69.3801175085246,211.603527846499,23.3713203435596)) ;
#77430=CARTESIAN_POINT('Origin',(69.3801175085246,211.603527846499,23.4913203435596)) ;
#77431=CARTESIAN_POINT('Ctrl Pts',(69.3801175085246,211.603527846499,23.3713203435596)) ;
#77432=CARTESIAN_POINT('Ctrl Pts',(69.9140887480339,208.410774997776,23.3713203435596)) ;
#77433=CARTESIAN_POINT('Ctrl Pts',(70.9826393962153,205.313240283402,23.3713203435596)) ;
#77434=CARTESIAN_POINT('Ctrl Pts',(72.4710003713498,202.438596367132,23.3713203435596)) ;
#77435=CARTESIAN_POINT('Ctrl Pts',(69.3801175085246,211.603527846499,23.3713203435596)) ;
#77436=CARTESIAN_POINT('Ctrl Pts',(69.3745683386693,211.63670777559,23.3713203435596)) ;
#77437=CARTESIAN_POINT('Ctrl Pts',(69.3393549802969,211.7104711332,23.3713203435596)) ;
#77438=CARTESIAN_POINT('Ctrl Pts',(69.2646228246277,211.74865896028,23.3713203435596)) ;
#77439=CARTESIAN_POINT('Ctrl Pts',(69.2199784169118,211.752993670653,23.3713203435596)) ;
#77440=CARTESIAN_POINT('Ctrl Pts',(69.4155295877472,211.609450331806,23.3713203435596)) ;
#77441=CARTESIAN_POINT('Ctrl Pts',(69.4088687502309,211.649277210824,23.3713203435596)) ;
#77442=CARTESIAN_POINT('Ctrl Pts',(69.3666495153969,211.737772406659,23.3713203435596)) ;
#77443=CARTESIAN_POINT('Ctrl Pts',(69.2770362017587,211.783526451141,23.3713203435596)) ;
#77444=CARTESIAN_POINT('Ctrl Pts',(69.2234481600225,211.788729535969,23.3713203435596)) ;
#77445=CARTESIAN_POINT('Ctrl Pts',(69.4768109371944,211.619699317454,23.4014788412624)) ;
#77446=CARTESIAN_POINT('Ctrl Pts',(69.4682405818884,211.670943699722,23.4014788412624)) ;
#77447=CARTESIAN_POINT('Ctrl Pts',(69.4138440642718,211.784877572449,23.4014788412624)) ;
#77448=CARTESIAN_POINT('Ctrl Pts',(69.2984031957674,211.843876507565,23.4014788412624)) ;
#77449=CARTESIAN_POINT('Ctrl Pts',(69.2294526236045,211.850571204073,23.4014788412624)) ;
#77450=CARTESIAN_POINT('Ctrl Pts',(69.4984736650468,211.623322295552,23.4643924065289)) ;
#77451=CARTESIAN_POINT('Ctrl Pts',(69.4892220419163,211.678640155241,23.4643924065289)) ;
#77452=CARTESIAN_POINT('Ctrl Pts',(69.4305443951831,211.801590709054,23.4643924065289)) ;
#77453=CARTESIAN_POINT('Ctrl Pts',(69.3060067148841,211.865205136511,23.4643924065289)) ;
#77454=CARTESIAN_POINT('Ctrl Pts',(69.2315751790255,211.872432002476,23.4643924065289)) ;
#77455=CARTESIAN_POINT('Ctrl Pts',(69.4984736650468,211.623322295552,23.4913203435596)) ;
#77456=CARTESIAN_POINT('Ctrl Pts',(69.4892250486213,211.67862217737,23.4913203435596)) ;
#77457=CARTESIAN_POINT('Ctrl Pts',(69.4305361180006,211.801561106719,23.4913203435596)) ;
#77458=CARTESIAN_POINT('Ctrl Pts',(69.3059825252186,211.865207485186,23.4913203435596)) ;
#77459=CARTESIAN_POINT('Ctrl Pts',(69.2315751790255,211.872432002476,23.4913203435596)) ;
#77460=CARTESIAN_POINT('',(69.2315751790255,211.872432002476,23.4913203435596)) ;
#77461=CARTESIAN_POINT('',(69.2199784169118,211.752993670653,23.3713203435596)) ;
#77462=CARTESIAN_POINT('Origin',(69.2199784169118,211.752993670653,23.4913203435596)) ;
#77463=CARTESIAN_POINT('Ctrl Pts',(69.2199784169118,211.752993670653,23.3713203435596)) ;
#77464=CARTESIAN_POINT('Ctrl Pts',(69.2646228246277,211.74865896028,23.3713203435596)) ;
#77465=CARTESIAN_POINT('Ctrl Pts',(69.3393549802969,211.7104711332,23.3713203435596)) ;
#77466=CARTESIAN_POINT('Ctrl Pts',(69.3745683386693,211.63670777559,23.3713203435596)) ;
#77467=CARTESIAN_POINT('Ctrl Pts',(69.3801175085246,211.603527846499,23.3713203435596)) ;
#77468=CARTESIAN_POINT('Ctrl Pts',(69.4984736650468,211.623322295552,23.4913203435596)) ;
#77469=CARTESIAN_POINT('Ctrl Pts',(69.4892250486213,211.67862217737,23.4913203435596)) ;
#77470=CARTESIAN_POINT('Ctrl Pts',(69.4305361180006,211.801561106719,23.4913203435596)) ;
#77471=CARTESIAN_POINT('Ctrl Pts',(69.3059825252186,211.865207485186,23.4913203435596)) ;
#77472=CARTESIAN_POINT('Ctrl Pts',(69.2315751790255,211.872432002476,23.4913203435596)) ;
#77473=CARTESIAN_POINT('Origin',(65.2251874189933,212.140864467154,23.4913203435596)) ;
#77474=CARTESIAN_POINT('',(65.236784181107,212.260302798977,23.4913203435596)) ;
#77475=CARTESIAN_POINT('',(65.2251874189933,212.140864467154,23.3713203435596)) ;
#77476=CARTESIAN_POINT('Origin',(67.6088474917769,207.295232147432,23.3713203435596)) ;
#77477=CARTESIAN_POINT('Ctrl Pts',(68.2200057399177,200.43583548982,23.3713203435596)) ;
#77478=CARTESIAN_POINT('Ctrl Pts',(68.1824073171725,200.43583548982,23.3713203435596)) ;
#77479=CARTESIAN_POINT('Ctrl Pts',(68.1076443008799,200.411538289219,23.3713203435596)) ;
#77480=CARTESIAN_POINT('Ctrl Pts',(68.0256156592925,200.299810943276,23.3713203435596)) ;
#77481=CARTESIAN_POINT('Ctrl Pts',(68.0408878207066,200.196696127704,23.3713203435596)) ;
#77482=CARTESIAN_POINT('Ctrl Pts',(68.073772979818,200.150878451592,23.3713203435596)) ;
#77483=CARTESIAN_POINT('Ctrl Pts',(68.2200057399177,200.471739405861,23.3713203435596)) ;
#77484=CARTESIAN_POINT('Ctrl Pts',(68.1748752084499,200.471739405861,23.3713203435596)) ;
#77485=CARTESIAN_POINT('Ctrl Pts',(68.0851812979518,200.442665155226,23.3713203435596)) ;
#77486=CARTESIAN_POINT('Ctrl Pts',(67.9867254555472,200.308566385953,23.3713203435596)) ;
#77487=CARTESIAN_POINT('Ctrl Pts',(68.0051314291745,200.1849394215,23.3713203435596)) ;
#77488=CARTESIAN_POINT('Ctrl Pts',(68.044604486812,200.129943069989,23.3713203435596)) ;
#77489=CARTESIAN_POINT('Ctrl Pts',(68.2200057399177,200.533872085375,23.4014786778375)) ;
#77490=CARTESIAN_POINT('Ctrl Pts',(68.1619372629609,200.533872085375,23.4014786778375)) ;
#77491=CARTESIAN_POINT('Ctrl Pts',(68.0464591301393,200.496324714954,23.4014786778375)) ;
#77492=CARTESIAN_POINT('Ctrl Pts',(67.9197695231301,200.323765978659,23.4014786778375)) ;
#77493=CARTESIAN_POINT('Ctrl Pts',(67.9433385076373,200.164476450385,23.4014786778375)) ;
#77494=CARTESIAN_POINT('Ctrl Pts',(67.9941276356022,200.09371383655,23.4014786778375)) ;
#77495=CARTESIAN_POINT('Ctrl Pts',(68.2200057399177,200.55583548982,23.4643924065289)) ;
#77496=CARTESIAN_POINT('Ctrl Pts',(68.1573213300674,200.55583548982,23.4643924065289)) ;
#77497=CARTESIAN_POINT('Ctrl Pts',(68.0327048929491,200.515383677869,23.4643924065289)) ;
#77498=CARTESIAN_POINT('Ctrl Pts',(67.895949576542,200.329117772152,23.4643924065289)) ;
#77499=CARTESIAN_POINT('Ctrl Pts',(67.9214580564103,200.15729471167,23.4643924065289)) ;
#77500=CARTESIAN_POINT('Ctrl Pts',(67.9762844730848,200.080907092773,23.4643924065289)) ;
#77501=CARTESIAN_POINT('Ctrl Pts',(68.2200057399177,200.55583548982,23.4913203435596)) ;
#77502=CARTESIAN_POINT('Ctrl Pts',(68.1573417020091,200.55583548982,23.4913203435596)) ;
#77503=CARTESIAN_POINT('Ctrl Pts',(68.0327366748546,200.515340155485,23.4913203435596)) ;
#77504=CARTESIAN_POINT('Ctrl Pts',(67.8960222722091,200.329127912246,23.4913203435596)) ;
#77505=CARTESIAN_POINT('Ctrl Pts',(67.9214758745658,200.157269886293,23.4913203435596)) ;
#77506=CARTESIAN_POINT('Ctrl Pts',(67.9762844730848,200.080907092773,23.4913203435596)) ;
#77507=CARTESIAN_POINT('',(67.9762844730848,200.080907092773,23.4913203435596)) ;
#77508=CARTESIAN_POINT('',(68.073772979818,200.150878451592,23.3713203435596)) ;
#77509=CARTESIAN_POINT('Origin',(68.073772979818,200.150878451592,23.4913203435596)) ;
#77510=CARTESIAN_POINT('',(68.2200057399177,200.43583548982,23.3713203435596)) ;
#77511=CARTESIAN_POINT('Ctrl Pts',(68.073772979818,200.150878451592,23.3713203435596)) ;
#77512=CARTESIAN_POINT('Ctrl Pts',(68.0408878207066,200.196696127704,23.3713203435596)) ;
#77513=CARTESIAN_POINT('Ctrl Pts',(68.0256156592925,200.299810943276,23.3713203435596)) ;
#77514=CARTESIAN_POINT('Ctrl Pts',(68.1076443008799,200.411538289219,23.3713203435596)) ;
#77515=CARTESIAN_POINT('Ctrl Pts',(68.1824073171725,200.43583548982,23.3713203435596)) ;
#77516=CARTESIAN_POINT('Ctrl Pts',(68.2200057399177,200.43583548982,23.3713203435596)) ;
#77517=CARTESIAN_POINT('',(68.2200057399177,200.55583548982,23.4913203435596)) ;
#77518=CARTESIAN_POINT('Origin',(68.2200057399177,200.43583548982,23.4913203435596)) ;
#77519=CARTESIAN_POINT('Ctrl Pts',(68.2200057399177,200.55583548982,23.4913203435596)) ;
#77520=CARTESIAN_POINT('Ctrl Pts',(68.1573417020091,200.55583548982,23.4913203435596)) ;
#77521=CARTESIAN_POINT('Ctrl Pts',(68.0327366748546,200.515340155485,23.4913203435596)) ;
#77522=CARTESIAN_POINT('Ctrl Pts',(67.8960222722091,200.329127912246,23.4913203435596)) ;
#77523=CARTESIAN_POINT('Ctrl Pts',(67.9214758745658,200.157269886293,23.4913203435596)) ;
#77524=CARTESIAN_POINT('Ctrl Pts',(67.9762844730848,200.080907092773,23.4913203435596)) ;
#77525=CARTESIAN_POINT('Ctrl Pts',(77.5627334640076,190.683545731522,23.4913203435596)) ;
#77526=CARTESIAN_POINT('Ctrl Pts',(73.9435688224726,193.341467670589,23.4913203435596)) ;
#77527=CARTESIAN_POINT('Ctrl Pts',(70.5986101113225,196.427317753425,23.4913203435596)) ;
#77528=CARTESIAN_POINT('Ctrl Pts',(67.9762844730849,200.080907092773,23.4913203435596)) ;
#77529=CARTESIAN_POINT('Ctrl Pts',(77.5627334640076,190.683545731522,23.4554164275186)) ;
#77530=CARTESIAN_POINT('Ctrl Pts',(73.9435444773532,193.341485549695,23.4554164275186)) ;
#77531=CARTESIAN_POINT('Ctrl Pts',(70.5986406627929,196.427275187191,23.4554164275186)) ;
#77532=CARTESIAN_POINT('Ctrl Pts',(67.9762844730849,200.080907092773,23.4554164275186)) ;
#77533=CARTESIAN_POINT('Ctrl Pts',(77.5805848919263,190.707853163496,23.3932837400762)) ;
#77534=CARTESIAN_POINT('Ctrl Pts',(73.9633403608045,193.364364969535,23.3932837400762)) ;
#77535=CARTESIAN_POINT('Ctrl Pts',(70.6207012559953,196.448260130978,23.3932837400762)) ;
#77536=CARTESIAN_POINT('Ctrl Pts',(68.0007852258362,200.098492252496,23.3932837400762)) ;
#77537=CARTESIAN_POINT('Ctrl Pts',(77.6178250208571,190.758561258377,23.3713203435596)) ;
#77538=CARTESIAN_POINT('Ctrl Pts',(74.0045722037604,193.412141541445,23.3713203435596)) ;
#77539=CARTESIAN_POINT('Ctrl Pts',(70.6668033103964,196.491924107876,23.3713203435596)) ;
#77540=CARTESIAN_POINT('Ctrl Pts',(68.0518966100636,200.13517691539,23.3713203435596)) ;
#77541=CARTESIAN_POINT('Ctrl Pts',(77.6337643041011,190.780265014789,23.3713203435596)) ;
#77542=CARTESIAN_POINT('Ctrl Pts',(74.0222174084502,193.432592465647,23.3713203435596)) ;
#77543=CARTESIAN_POINT('Ctrl Pts',(70.6865388646701,196.510608363121,23.3713203435596)) ;
#77544=CARTESIAN_POINT('Ctrl Pts',(68.073772979818,200.150878451592,23.3713203435596)) ;
#77545=CARTESIAN_POINT('Ctrl Pts',(67.9762844730849,200.080907092773,23.4913203435596)) ;
#77546=CARTESIAN_POINT('Ctrl Pts',(70.5986101113225,196.427317753425,23.4913203435596)) ;
#77547=CARTESIAN_POINT('Ctrl Pts',(73.9435688224726,193.341467670589,23.4913203435596)) ;
#77548=CARTESIAN_POINT('Ctrl Pts',(77.5627334640076,190.683545731522,23.4913203435596)) ;
#77549=CARTESIAN_POINT('',(77.6337643041011,190.780265014789,23.3713203435596)) ;
#77550=CARTESIAN_POINT('Origin',(77.6337643041011,190.780265014789,23.4913203435596)) ;
#77551=CARTESIAN_POINT('Ctrl Pts',(77.6337643041011,190.780265014789,23.3713203435596)) ;
#77552=CARTESIAN_POINT('Ctrl Pts',(74.0222174084502,193.432592465647,23.3713203435596)) ;
#77553=CARTESIAN_POINT('Ctrl Pts',(70.6865388646701,196.510608363121,23.3713203435596)) ;
#77554=CARTESIAN_POINT('Ctrl Pts',(68.073772979818,200.150878451592,23.3713203435596)) ;
#77555=CARTESIAN_POINT('Ctrl Pts',(77.6337643041011,190.780265014789,23.3713203435596)) ;
#77556=CARTESIAN_POINT('Ctrl Pts',(77.7835229891055,190.670281929225,23.3713203435596)) ;
#77557=CARTESIAN_POINT('Ctrl Pts',(77.9688509344519,190.609539758744,23.3713203435596)) ;
#77558=CARTESIAN_POINT('Ctrl Pts',(78.1546571314538,190.609539758744,23.3713203435596)) ;
#77559=CARTESIAN_POINT('Ctrl Pts',(77.6125119264424,190.751326672906,23.3713203435596)) ;
#77560=CARTESIAN_POINT('Ctrl Pts',(77.7684072254185,190.63683684545,23.3713203435596)) ;
#77561=CARTESIAN_POINT('Ctrl Pts',(77.9612372130539,190.573635842703,23.3713203435596)) ;
#77562=CARTESIAN_POINT('Ctrl Pts',(78.1546571314538,190.573635842703,23.3713203435596)) ;
#77563=CARTESIAN_POINT('Ctrl Pts',(77.5757341216353,190.701248102578,23.4014786760343)) ;
#77564=CARTESIAN_POINT('Ctrl Pts',(77.7421703169228,190.579017019241,23.4014786760343)) ;
#77565=CARTESIAN_POINT('Ctrl Pts',(77.9481590810139,190.511503161025,23.4014786760343)) ;
#77566=CARTESIAN_POINT('Ctrl Pts',(78.1546571314538,190.511503161025,23.4014786760343)) ;
#77567=CARTESIAN_POINT('Ctrl Pts',(77.5627334640076,190.683545731522,23.4643924065289)) ;
#77568=CARTESIAN_POINT('Ctrl Pts',(77.7329303854515,190.558552763179,23.4643924065289)) ;
#77569=CARTESIAN_POINT('Ctrl Pts',(77.943493133092,190.489539758744,23.4643924065289)) ;
#77570=CARTESIAN_POINT('Ctrl Pts',(78.1546571314538,190.489539758744,23.4643924065289)) ;
#77571=CARTESIAN_POINT('Ctrl Pts',(77.5627334640076,190.683545731522,23.4913203435596)) ;
#77572=CARTESIAN_POINT('Ctrl Pts',(77.7329137878762,190.558564952473,23.4913203435596)) ;
#77573=CARTESIAN_POINT('Ctrl Pts',(77.9435137257698,190.489539758744,23.4913203435596)) ;
#77574=CARTESIAN_POINT('Ctrl Pts',(78.1546571314538,190.489539758744,23.4913203435596)) ;
#77575=CARTESIAN_POINT('',(78.1546571314538,190.609539758744,23.3713203435596)) ;
#77576=CARTESIAN_POINT('Origin',(78.1546571314538,190.609539758744,23.4913203435596)) ;
#77577=CARTESIAN_POINT('Origin',(78.0868516728036,191.282661304515,23.3713203435596)) ;
#77578=CARTESIAN_POINT('Origin',(78.07353074889,190.609539758744,23.4913203435596)) ;
#77579=CARTESIAN_POINT('',(80.8501919227397,190.609539758744,23.3713203435596)) ;
#77580=CARTESIAN_POINT('Origin',(80.8501919227397,190.609539758744,23.4913203435596)) ;
#77581=CARTESIAN_POINT('',(78.07353074889,190.609539758744,23.3713203435596)) ;
#77582=CARTESIAN_POINT('Ctrl Pts',(80.8501919227397,190.609539758744,23.3713203435596)) ;
#77583=CARTESIAN_POINT('Ctrl Pts',(80.8900960147986,190.609539758744,23.3713203435596)) ;
#77584=CARTESIAN_POINT('Ctrl Pts',(80.9697731323004,190.637124645342,23.3713203435596)) ;
#77585=CARTESIAN_POINT('Ctrl Pts',(81.0384684533381,190.743413070952,23.3713203435596)) ;
#77586=CARTESIAN_POINT('Ctrl Pts',(81.0287354417464,190.84834644111,23.3713203435596)) ;
#77587=CARTESIAN_POINT('Ctrl Pts',(80.9947301225929,190.898658010764,23.3713203435596)) ;
#77588=CARTESIAN_POINT('Ctrl Pts',(80.9810274260323,190.913160432898,23.3713203435596)) ;
#77589=CARTESIAN_POINT('Ctrl Pts',(80.8501919227397,190.573635842703,23.3713203435596)) ;
#77590=CARTESIAN_POINT('Ctrl Pts',(80.8980900192787,190.573635842703,23.3713203435596)) ;
#77591=CARTESIAN_POINT('Ctrl Pts',(80.9936901650968,190.606657008214,23.3713203435596)) ;
#77592=CARTESIAN_POINT('Ctrl Pts',(81.0761224171995,190.734180607265,23.3713203435596)) ;
#77593=CARTESIAN_POINT('Ctrl Pts',(81.064410508624,190.860067831686,23.3713203435596)) ;
#77594=CARTESIAN_POINT('Ctrl Pts',(81.0235724505757,190.920410880242,23.3713203435596)) ;
#77595=CARTESIAN_POINT('Ctrl Pts',(81.0071246867289,190.937818579041,23.3713203435596)) ;
#77596=CARTESIAN_POINT('Ctrl Pts',(80.8501919227397,190.511503216626,23.4014787223741)) ;
#77597=CARTESIAN_POINT('Ctrl Pts',(80.9118213657063,190.511503216626,23.4014787223741)) ;
#77598=CARTESIAN_POINT('Ctrl Pts',(81.034887159699,190.554128041159,23.4014787223741)) ;
#77599=CARTESIAN_POINT('Ctrl Pts',(81.1409888893296,190.718297939174,23.4014787223741)) ;
#77600=CARTESIAN_POINT('Ctrl Pts',(81.1259638528477,190.880377412799,23.4014787223741)) ;
#77601=CARTESIAN_POINT('Ctrl Pts',(81.073449631436,190.958092009754,23.4014787223741)) ;
#77602=CARTESIAN_POINT('Ctrl Pts',(81.0522866500825,190.98049011861,23.4014787223741)) ;
#77603=CARTESIAN_POINT('Ctrl Pts',(80.8501919227397,190.489539758744,23.4643924065289)) ;
#77604=CARTESIAN_POINT('Ctrl Pts',(80.9167203640597,190.489539758744,23.4643924065289)) ;
#77605=CARTESIAN_POINT('Ctrl Pts',(81.0495344536617,190.535473208199,23.4643924065289)) ;
#77606=CARTESIAN_POINT('Ctrl Pts',(81.164048307672,190.7126420413,23.4643924065289)) ;
#77607=CARTESIAN_POINT('Ctrl Pts',(81.1478031175844,190.887545532602,23.4643924065289)) ;
#77608=CARTESIAN_POINT('Ctrl Pts',(81.0910963470228,190.971395654268,23.4643924065289)) ;
#77609=CARTESIAN_POINT('Ctrl Pts',(81.068251094894,190.995574215667,23.4643924065289)) ;
#77610=CARTESIAN_POINT('Ctrl Pts',(80.8501919227397,190.489539758744,23.4913203435596)) ;
#77611=CARTESIAN_POINT('Ctrl Pts',(80.9166987428379,190.489539758744,23.4913203435596)) ;
#77612=CARTESIAN_POINT('Ctrl Pts',(81.0494939386742,190.535514569741,23.4913203435596)) ;
#77613=CARTESIAN_POINT('Ctrl Pts',(81.1639861404037,190.712661945758,23.4913203435596)) ;
#77614=CARTESIAN_POINT('Ctrl Pts',(81.1477644544174,190.887550896021,23.4913203435596)) ;
#77615=CARTESIAN_POINT('Ctrl Pts',(81.091088922495,190.971403512111,23.4913203435596)) ;
#77616=CARTESIAN_POINT('Ctrl Pts',(81.068251094894,190.995574215667,23.4913203435596)) ;
#77617=CARTESIAN_POINT('',(80.9810274260323,190.913160432898,23.3713203435596)) ;
#77618=CARTESIAN_POINT('Origin',(80.9810274260323,190.913160432898,23.4913203435596)) ;
#77619=CARTESIAN_POINT('Ctrl Pts',(80.9810274260323,190.913160432898,23.3713203435596)) ;
#77620=CARTESIAN_POINT('Ctrl Pts',(80.9947301225929,190.898658010764,23.3713203435596)) ;
#77621=CARTESIAN_POINT('Ctrl Pts',(81.0287354417464,190.84834644111,23.3713203435596)) ;
#77622=CARTESIAN_POINT('Ctrl Pts',(81.0384684533381,190.743413070952,23.3713203435596)) ;
#77623=CARTESIAN_POINT('Ctrl Pts',(80.9697731323004,190.637124645342,23.3713203435596)) ;
#77624=CARTESIAN_POINT('Ctrl Pts',(80.8900960147986,190.609539758744,23.3713203435596)) ;
#77625=CARTESIAN_POINT('Ctrl Pts',(80.8501919227397,190.609539758744,23.3713203435596)) ;
#77626=CARTESIAN_POINT('Ctrl Pts',(73.7436956568154,200.410454788892,23.4913203435596)) ;
#77627=CARTESIAN_POINT('Ctrl Pts',(75.7953376765802,196.999191831293,23.4913203435596)) ;
#77628=CARTESIAN_POINT('Ctrl Pts',(78.3304755598256,193.893133563934,23.4913203435596)) ;
#77629=CARTESIAN_POINT('Ctrl Pts',(81.0682510948939,190.995574215667,23.4913203435596)) ;
#77630=CARTESIAN_POINT('Ctrl Pts',(73.7436956568154,200.410454788892,23.4554164275186)) ;
#77631=CARTESIAN_POINT('Ctrl Pts',(75.795318037376,196.999224485377,23.4554164275186)) ;
#77632=CARTESIAN_POINT('Ctrl Pts',(78.3304892457748,193.893119079237,23.4554164275186)) ;
#77633=CARTESIAN_POINT('Ctrl Pts',(81.0682510948939,190.995574215667,23.4554164275186)) ;
#77634=CARTESIAN_POINT('Ctrl Pts',(73.7178513760089,200.394911216575,23.3932838348228)) ;
#77635=CARTESIAN_POINT('Ctrl Pts',(75.7710423485568,196.981072816866,23.3932838348228)) ;
#77636=CARTESIAN_POINT('Ctrl Pts',(78.3074750856353,193.873563742023,23.3932838348228)) ;
#77637=CARTESIAN_POINT('Ctrl Pts',(81.0463300376127,190.974861979224,23.3932838348228)) ;
#77638=CARTESIAN_POINT('Ctrl Pts',(73.6639374467842,200.362485665093,23.3713203435596)) ;
#77639=CARTESIAN_POINT('Ctrl Pts',(75.7203485344392,196.943293183495,23.3713203435596)) ;
#77640=CARTESIAN_POINT('Ctrl Pts',(78.2595014217398,193.832730768784,23.3713203435596)) ;
#77641=CARTESIAN_POINT('Ctrl Pts',(81.0006003715547,190.931654042505,23.3713203435596)) ;
#77642=CARTESIAN_POINT('Ctrl Pts',(73.6408615205729,200.348607069263,23.3713203435596)) ;
#77643=CARTESIAN_POINT('Ctrl Pts',(75.6986487748031,196.927126436994,23.3713203435596)) ;
#77644=CARTESIAN_POINT('Ctrl Pts',(78.2389694686303,193.81525213698,23.3713203435596)) ;
#77645=CARTESIAN_POINT('Ctrl Pts',(80.9810274260322,190.913160432898,23.3713203435596)) ;
#77646=CARTESIAN_POINT('',(73.6408615205729,200.348607069263,23.3713203435596)) ;
#77647=CARTESIAN_POINT('Origin',(73.6408615205729,200.348607069263,23.4913203435596)) ;
#77648=CARTESIAN_POINT('Ctrl Pts',(73.6408615205729,200.348607069263,23.3713203435596)) ;
#77649=CARTESIAN_POINT('Ctrl Pts',(75.6986487748031,196.927126436994,23.3713203435596)) ;
#77650=CARTESIAN_POINT('Ctrl Pts',(78.2389694686303,193.81525213698,23.3713203435596)) ;
#77651=CARTESIAN_POINT('Ctrl Pts',(80.9810274260322,190.913160432898,23.3713203435596)) ;
#77652=CARTESIAN_POINT('Ctrl Pts',(73.6408615205729,200.348607069263,23.3713203435596)) ;
#77653=CARTESIAN_POINT('Ctrl Pts',(73.609031832983,200.401530256243,23.3713203435596)) ;
#77654=CARTESIAN_POINT('Ctrl Pts',(73.548367847994,200.43583548982,23.3713203435596)) ;
#77655=CARTESIAN_POINT('Ctrl Pts',(73.4866103162092,200.43583548982,23.3713203435596)) ;
#77656=CARTESIAN_POINT('Ctrl Pts',(73.6716294221879,200.367111863704,23.3713203435596)) ;
#77657=CARTESIAN_POINT('Ctrl Pts',(73.6334232791504,200.430637176229,23.3713203435596)) ;
#77658=CARTESIAN_POINT('Ctrl Pts',(73.5607397617575,200.471739405861,23.3713203435596)) ;
#77659=CARTESIAN_POINT('Ctrl Pts',(73.4866103162092,200.471739405861,23.3713203435596)) ;
#77660=CARTESIAN_POINT('Ctrl Pts',(73.7248740178776,200.399134856713,23.4014787503538)) ;
#77661=CARTESIAN_POINT('Ctrl Pts',(73.6757150014773,200.480871499881,23.4014787503538)) ;
#77662=CARTESIAN_POINT('Ctrl Pts',(73.5819910675684,200.533871998366,23.4014787503538)) ;
#77663=CARTESIAN_POINT('Ctrl Pts',(73.4866103162092,200.533871998366,23.4014787503538)) ;
#77664=CARTESIAN_POINT('Ctrl Pts',(73.7436956568153,200.410454788892,23.4643924065289)) ;
#77665=CARTESIAN_POINT('Ctrl Pts',(73.6906289312292,200.498688775878,23.4643924065289)) ;
#77666=CARTESIAN_POINT('Ctrl Pts',(73.5895729979147,200.55583548982,23.4643924065289)) ;
#77667=CARTESIAN_POINT('Ctrl Pts',(73.4866103162092,200.55583548982,23.4643924065289)) ;
#77668=CARTESIAN_POINT('Ctrl Pts',(73.7436956568153,200.410454788892,23.4913203435596)) ;
#77669=CARTESIAN_POINT('Ctrl Pts',(73.6906461774989,200.498660100524,23.4913203435596)) ;
#77670=CARTESIAN_POINT('Ctrl Pts',(73.5895395358505,200.55583548982,23.4913203435596)) ;
#77671=CARTESIAN_POINT('Ctrl Pts',(73.4866103162092,200.55583548982,23.4913203435596)) ;
#77672=CARTESIAN_POINT('',(73.4866103162092,200.55583548982,23.4913203435596)) ;
#77673=CARTESIAN_POINT('',(73.4866103162092,200.43583548982,23.3713203435596)) ;
#77674=CARTESIAN_POINT('Origin',(73.4866103162092,200.43583548982,23.4913203435596)) ;
#77675=CARTESIAN_POINT('Origin',(73.5079774294674,200.293620227099,23.3713203435596)) ;
#77676=CARTESIAN_POINT('Origin',(73.5222221716416,200.318810051951,23.4913203435596)) ;
#77677=CARTESIAN_POINT('Origin',(71.1190430355237,200.43583548982,23.4913203435596)) ;
#77678=CARTESIAN_POINT('',(71.1190430355237,200.55583548982,23.4913203435596)) ;
#77679=CARTESIAN_POINT('',(71.1190430355237,200.43583548982,23.3713203435596)) ;
#77680=CARTESIAN_POINT('Ctrl Pts',(77.8285014478222,190.489539758744,17.8547522895864)) ;
#77681=CARTESIAN_POINT('Ctrl Pts',(77.8285014478222,190.489539758744,32.8746339543542)) ;
#77682=CARTESIAN_POINT('Ctrl Pts',(73.8355349189945,193.386814152385,17.8547522895863)) ;
#77683=CARTESIAN_POINT('Ctrl Pts',(73.8355349189945,193.386814152385,32.8746339543541)) ;
#77684=CARTESIAN_POINT('Ctrl Pts',(70.4532522157592,196.594204259059,17.8547522895864)) ;
#77685=CARTESIAN_POINT('Ctrl Pts',(70.4532522157592,196.594204259059,32.8746339543542)) ;
#77686=CARTESIAN_POINT('Ctrl Pts',(67.88518965836,200.208466979566,17.8547522895864)) ;
#77687=CARTESIAN_POINT('Ctrl Pts',(67.88518965836,200.208466979566,32.8746339543542)) ;
#77688=CARTESIAN_POINT('Ctrl Pts',(67.8032385132701,200.323804110956,17.8547522895864)) ;
#77689=CARTESIAN_POINT('Ctrl Pts',(67.8032385132701,200.323804110956,32.8746339543542)) ;
#77690=CARTESIAN_POINT('Ctrl Pts',(67.7220901562832,200.439592363042,17.8547522895864)) ;
#77691=CARTESIAN_POINT('Ctrl Pts',(67.7220901562832,200.439592363042,32.8746339543542)) ;
#77692=CARTESIAN_POINT('Ctrl Pts',(67.6417475736103,200.555835489811,17.8547522895864)) ;
#77693=CARTESIAN_POINT('Ctrl Pts',(67.6417475736103,200.555835489811,32.8746339543542)) ;
#77694=CARTESIAN_POINT('',(67.9762844730848,200.080907092773,30.2513203435596)) ;
#77695=CARTESIAN_POINT('Ctrl Pts',(67.9762844730848,200.080907092773,23.4913203435596)) ;
#77696=CARTESIAN_POINT('Ctrl Pts',(67.9762844730848,200.080907092773,31.6033203435596)) ;
#77697=CARTESIAN_POINT('Ctrl Pts',(67.9397439452691,200.131817658927,23.4913203435596)) ;
#77698=CARTESIAN_POINT('Ctrl Pts',(67.9397439452691,200.131817658927,31.6033203435596)) ;
#77699=CARTESIAN_POINT('Ctrl Pts',(67.8999789504624,200.256667577061,23.4913203435596)) ;
#77700=CARTESIAN_POINT('Ctrl Pts',(67.8999789504624,200.256667577061,31.6033203435596)) ;
#77701=CARTESIAN_POINT('Ctrl Pts',(67.9715322297243,200.476322658598,23.4913203435596)) ;
#77702=CARTESIAN_POINT('Ctrl Pts',(67.9715322297243,200.476322658598,31.6033203435596)) ;
#77703=CARTESIAN_POINT('Ctrl Pts',(68.1260059217369,200.55583548982,23.4913203435596)) ;
#77704=CARTESIAN_POINT('Ctrl Pts',(68.1260059217369,200.55583548982,31.6033203435596)) ;
#77705=CARTESIAN_POINT('Ctrl Pts',(68.2200057399177,200.55583548982,23.4913203435596)) ;
#77706=CARTESIAN_POINT('Ctrl Pts',(68.2200057399177,200.55583548982,31.6033203435596)) ;
#77707=CARTESIAN_POINT('',(68.2200057399177,200.55583548982,23.4913203435596)) ;
#77708=CARTESIAN_POINT('Origin',(74.5963384974435,195.522687624282,23.3713203435596)) ;
#77709=CARTESIAN_POINT('Origin',(73.5885500808522,200.43583548982,19.2513203435596)) ;
#77710=CARTESIAN_POINT('',(73.5885500808522,200.55583548982,19.2513203435596)) ;
#77711=CARTESIAN_POINT('',(73.5885500808522,200.43583548982,19.3713203435596)) ;
#77712=CARTESIAN_POINT('Origin',(73.5885500808522,200.43583548982,19.2513203435596)) ;
#77713=CARTESIAN_POINT('',(73.6915408905797,200.497421958396,19.2513203435596)) ;
#77714=CARTESIAN_POINT('Origin',(73.5885500808522,200.43583548982,19.2513203435596)) ;
#77715=CARTESIAN_POINT('Origin',(73.5885500808522,200.43583548982,19.2513203435596)) ;
#77716=CARTESIAN_POINT('Ctrl Pts',(73.6915408905803,200.497421958395,17.9913203435596)) ;
#77717=CARTESIAN_POINT('Ctrl Pts',(73.6824627768405,200.512603252379,17.9913203435596)) ;
#77718=CARTESIAN_POINT('Ctrl Pts',(73.6533226941628,200.543288099199,17.9913203435596)) ;
#77719=CARTESIAN_POINT('Ctrl Pts',(73.6121347778153,200.55583548982,17.9913203435596)) ;
#77720=CARTESIAN_POINT('Ctrl Pts',(73.5885500808522,200.55583548982,17.9913203435596)) ;
#77721=CARTESIAN_POINT('Ctrl Pts',(73.6915408905803,200.497421958395,17.9554164275186)) ;
#77722=CARTESIAN_POINT('Ctrl Pts',(73.6824917890662,200.512554735348,17.9554164275186)) ;
#77723=CARTESIAN_POINT('Ctrl Pts',(73.653329650592,200.543206850976,17.9554164275186)) ;
#77724=CARTESIAN_POINT('Ctrl Pts',(73.612059404828,200.55583548982,17.9554164275186)) ;
#77725=CARTESIAN_POINT('Ctrl Pts',(73.5885500808522,200.55583548982,17.9554164275186)) ;
#77726=CARTESIAN_POINT('Ctrl Pts',(73.7174244840934,200.512899835719,17.8932837474712)) ;
#77727=CARTESIAN_POINT('Ctrl Pts',(73.7060581631873,200.531907689569,17.8932837474712)) ;
#77728=CARTESIAN_POINT('Ctrl Pts',(73.6695997049772,200.570311794726,17.8932837474712)) ;
#77729=CARTESIAN_POINT('Ctrl Pts',(73.6180794789012,200.585993823654,17.8932837474712)) ;
#77730=CARTESIAN_POINT('Ctrl Pts',(73.5885500808522,200.585993823654,17.8932837474712)) ;
#77731=CARTESIAN_POINT('Ctrl Pts',(73.7714206166492,200.545188455739,17.8713203435596)) ;
#77732=CARTESIAN_POINT('Ctrl Pts',(73.755297346051,200.572151337892,17.8713203435596)) ;
#77733=CARTESIAN_POINT('Ctrl Pts',(73.703559367871,200.626640069246,17.8713203435596)) ;
#77734=CARTESIAN_POINT('Ctrl Pts',(73.6304379071134,200.648907552789,17.8713203435596)) ;
#77735=CARTESIAN_POINT('Ctrl Pts',(73.5885500808522,200.648907552789,17.8713203435596)) ;
#77736=CARTESIAN_POINT('Ctrl Pts',(73.7945317003084,200.55900842697,17.8713203435596)) ;
#77737=CARTESIAN_POINT('Ctrl Pts',(73.7763754728287,200.589371014938,17.8713203435596)) ;
#77738=CARTESIAN_POINT('Ctrl Pts',(73.7180953074733,200.650740708578,17.8713203435596)) ;
#77739=CARTESIAN_POINT('Ctrl Pts',(73.6357194747785,200.67583548982,17.8713203435596)) ;
#77740=CARTESIAN_POINT('Ctrl Pts',(73.5885500808522,200.67583548982,17.8713203435596)) ;
#77741=CARTESIAN_POINT('',(73.6915408905803,200.497421958395,17.9913203435596)) ;
#77742=CARTESIAN_POINT('',(73.7945317003084,200.55900842697,17.8713203435596)) ;
#77743=CARTESIAN_POINT('Origin',(73.7945317003084,200.55900842697,17.9913203435596)) ;
#77744=CARTESIAN_POINT('',(73.5885500808522,200.55583548982,17.9913203435596)) ;
#77745=CARTESIAN_POINT('Origin',(73.5831295493737,200.427665247194,17.9913203435596)) ;
#77746=CARTESIAN_POINT('',(73.5885500808522,200.67583548982,17.8713203435596)) ;
#77747=CARTESIAN_POINT('Origin',(73.5885500808522,200.67583548982,17.9913203435596)) ;
#77748=CARTESIAN_POINT('Ctrl Pts',(73.5885500808522,200.67583548982,17.8713203435596)) ;
#77749=CARTESIAN_POINT('Ctrl Pts',(73.6357194747785,200.67583548982,17.8713203435596)) ;
#77750=CARTESIAN_POINT('Ctrl Pts',(73.7180953074733,200.650740708578,17.8713203435596)) ;
#77751=CARTESIAN_POINT('Ctrl Pts',(73.7763754728287,200.589371014938,17.8713203435596)) ;
#77752=CARTESIAN_POINT('Ctrl Pts',(73.7945317003084,200.55900842697,17.8713203435596)) ;
#77753=CARTESIAN_POINT('Ctrl Pts',(73.6915408905803,200.497421958395,19.2513203435596)) ;
#77754=CARTESIAN_POINT('Ctrl Pts',(73.6915408905803,200.497421958395,17.7393203435596)) ;
#77755=CARTESIAN_POINT('Ctrl Pts',(73.6703579522658,200.532846103015,19.2513203435596)) ;
#77756=CARTESIAN_POINT('Ctrl Pts',(73.6703579522658,200.532846103015,17.7393203435596)) ;
#77757=CARTESIAN_POINT('Ctrl Pts',(73.6298246117119,200.55583548982,19.2513203435596)) ;
#77758=CARTESIAN_POINT('Ctrl Pts',(73.6298246117119,200.55583548982,17.7393203435596)) ;
#77759=CARTESIAN_POINT('Ctrl Pts',(73.5885500808522,200.55583548982,19.2513203435596)) ;
#77760=CARTESIAN_POINT('Ctrl Pts',(73.5885500808522,200.55583548982,17.7393203435596)) ;
#77761=CARTESIAN_POINT('',(73.6915408905803,200.497421958395,17.9913203435596)) ;
#77762=CARTESIAN_POINT('',(73.5885500808522,200.55583548982,19.2513203435596)) ;
#77763=CARTESIAN_POINT('Origin',(67.8715456014014,200.43583548982,19.2513203435596)) ;
#77764=CARTESIAN_POINT('',(67.8715456014017,200.55583548982,19.2513203435596)) ;
#77765=CARTESIAN_POINT('',(67.8530878290255,200.554407453787,19.2513203435596)) ;
#77766=CARTESIAN_POINT('Origin',(67.8715456014017,200.43583548982,19.2513203435596)) ;
#77767=CARTESIAN_POINT('',(67.8715456014015,200.43583548982,19.3713203435596)) ;
#77768=CARTESIAN_POINT('Origin',(67.8715456014014,200.43583548982,19.2513203435596)) ;
#77769=CARTESIAN_POINT('',(67.7733141415173,200.366911043569,19.2513203435596)) ;
#77770=CARTESIAN_POINT('Origin',(67.8715456014017,200.43583548982,19.2513203435596)) ;
#77771=CARTESIAN_POINT('',(67.7526891574347,200.452362610789,19.2513203435596)) ;
#77772=CARTESIAN_POINT('Origin',(67.8715456014017,200.43583548982,19.2513203435596)) ;
#77773=CARTESIAN_POINT('Origin',(67.8715456014017,200.43583548982,19.2513203435596)) ;
#77774=CARTESIAN_POINT('Origin',(71.1190430355237,200.43583548982,19.2513203435596)) ;
#77775=CARTESIAN_POINT('',(71.1190430355237,200.55583548982,19.2513203435596)) ;
#77776=CARTESIAN_POINT('',(71.1190430355237,200.43583548982,19.3713203435596)) ;
#77777=CARTESIAN_POINT('Ctrl Pts',(67.7733141381132,200.366911041181,19.2513203435596)) ;
#77778=CARTESIAN_POINT('Ctrl Pts',(70.4235001348744,196.589852920486,19.2513203435596)) ;
#77779=CARTESIAN_POINT('Ctrl Pts',(73.8497225151601,193.410388591247,19.2513203435596)) ;
#77780=CARTESIAN_POINT('Ctrl Pts',(77.5627334640076,190.683545731522,19.2513203435596)) ;
#77781=CARTESIAN_POINT('Ctrl Pts',(67.7733141381132,200.366911041181,19.2872242596007)) ;
#77782=CARTESIAN_POINT('Ctrl Pts',(70.4235312581646,196.58980856342,19.2872242596007)) ;
#77783=CARTESIAN_POINT('Ctrl Pts',(73.8496975387625,193.410406933965,19.2872242596007)) ;
#77784=CARTESIAN_POINT('Ctrl Pts',(77.5627334640076,190.683545731522,19.2872242596007)) ;
#77785=CARTESIAN_POINT('Ctrl Pts',(67.7980015646804,200.384233060089,19.3493570138488)) ;
#77786=CARTESIAN_POINT('Ctrl Pts',(70.4457328536727,196.610673400983,19.3493570138488)) ;
#77787=CARTESIAN_POINT('Ctrl Pts',(73.8695438097236,193.433249280034,19.3493570138488)) ;
#77788=CARTESIAN_POINT('Ctrl Pts',(77.5805848589692,190.70785311862,19.3493570138488)) ;
#77789=CARTESIAN_POINT('Ctrl Pts',(67.8495025125859,200.420368879713,19.3713203435596)) ;
#77790=CARTESIAN_POINT('Ctrl Pts',(70.4921307140883,196.654082166003,19.3713203435596)) ;
#77791=CARTESIAN_POINT('Ctrl Pts',(73.9108791922903,193.480949881322,19.3713203435597)) ;
#77792=CARTESIAN_POINT('Ctrl Pts',(77.6178250208571,190.758561258377,19.3713203435597)) ;
#77793=CARTESIAN_POINT('Ctrl Pts',(67.8715456014015,200.43583548982,19.3713203435596)) ;
#77794=CARTESIAN_POINT('Ctrl Pts',(70.5119929186185,196.672656983123,19.3713203435596)) ;
#77795=CARTESIAN_POINT('Ctrl Pts',(73.9285686321681,193.501368319111,19.3713203435597)) ;
#77796=CARTESIAN_POINT('Ctrl Pts',(77.6337643041012,190.780265014789,19.3713203435597)) ;
#77797=CARTESIAN_POINT('',(77.6337643041012,190.780265014789,19.3713203435596)) ;
#77798=CARTESIAN_POINT('Ctrl Pts',(67.8715456014015,200.43583548982,19.3713203435596)) ;
#77799=CARTESIAN_POINT('Ctrl Pts',(70.5119929186185,196.672656983123,19.3713203435596)) ;
#77800=CARTESIAN_POINT('Ctrl Pts',(73.9285686321681,193.501368319111,19.3713203435597)) ;
#77801=CARTESIAN_POINT('Ctrl Pts',(77.6337643041012,190.780265014789,19.3713203435597)) ;
#77802=CARTESIAN_POINT('',(77.5627294322141,190.683540239233,19.2513203435596)) ;
#77803=CARTESIAN_POINT('Origin',(77.6337643041012,190.780265014789,19.2513203435596)) ;
#77804=CARTESIAN_POINT('Ctrl Pts',(77.5627126756809,190.683517412735,19.2513203435596)) ;
#77805=CARTESIAN_POINT('Ctrl Pts',(73.685331711946,193.529834997272,19.2513203435595)) ;
#77806=CARTESIAN_POINT('Ctrl Pts',(70.3960766724624,196.674672483662,19.2513203435596)) ;
#77807=CARTESIAN_POINT('Ctrl Pts',(67.88518965836,200.208466979566,19.2513203435596)) ;
#77808=CARTESIAN_POINT('Ctrl Pts',(67.8477299947086,200.261187294135,19.2513203435596)) ;
#77809=CARTESIAN_POINT('Ctrl Pts',(67.8104380640988,200.314001865016,19.2513203435596)) ;
#77810=CARTESIAN_POINT('Ctrl Pts',(67.7733141517289,200.366911050735,19.2513203435596)) ;
#77811=CARTESIAN_POINT('Ctrl Pts',(78.1546571314538,190.609539758744,19.3713203435596)) ;
#77812=CARTESIAN_POINT('Ctrl Pts',(77.9688509344519,190.609539758744,19.3713203435596)) ;
#77813=CARTESIAN_POINT('Ctrl Pts',(77.7835229891055,190.670281929225,19.3713203435596)) ;
#77814=CARTESIAN_POINT('Ctrl Pts',(77.6337643041011,190.780265014789,19.3713203435596)) ;
#77815=CARTESIAN_POINT('Ctrl Pts',(78.1546571314538,190.573635842703,19.3713203435596)) ;
#77816=CARTESIAN_POINT('Ctrl Pts',(77.9612372130539,190.573635842703,19.3713203435596)) ;
#77817=CARTESIAN_POINT('Ctrl Pts',(77.7684072254185,190.63683684545,19.3713203435596)) ;
#77818=CARTESIAN_POINT('Ctrl Pts',(77.6125119264425,190.751326672906,19.3713203435596)) ;
#77819=CARTESIAN_POINT('Ctrl Pts',(78.1546571314538,190.511503094374,19.3411620666336)) ;
#77820=CARTESIAN_POINT('Ctrl Pts',(77.9481590810139,190.511503094374,19.3411620666336)) ;
#77821=CARTESIAN_POINT('Ctrl Pts',(77.7421702774708,190.579016965521,19.3411620666336)) ;
#77822=CARTESIAN_POINT('Ctrl Pts',(77.5757340821833,190.701248048858,19.3411620666336)) ;
#77823=CARTESIAN_POINT('Ctrl Pts',(78.1546571314538,190.489539758744,19.2782482805904)) ;
#77824=CARTESIAN_POINT('Ctrl Pts',(77.943493133092,190.489539758744,19.2782482805904)) ;
#77825=CARTESIAN_POINT('Ctrl Pts',(77.7329303854515,190.558552763179,19.2782482805904)) ;
#77826=CARTESIAN_POINT('Ctrl Pts',(77.5627334640076,190.683545731522,19.2782482805904)) ;
#77827=CARTESIAN_POINT('Ctrl Pts',(78.1546571314538,190.489539758744,19.2513203435596)) ;
#77828=CARTESIAN_POINT('Ctrl Pts',(77.9435137257698,190.489539758744,19.2513203435596)) ;
#77829=CARTESIAN_POINT('Ctrl Pts',(77.7329137878762,190.558564952473,19.2513203435596)) ;
#77830=CARTESIAN_POINT('Ctrl Pts',(77.5627334640076,190.683545731522,19.2513203435596)) ;
#77831=CARTESIAN_POINT('',(78.1546571314538,190.609539758744,19.3713203435596)) ;
#77832=CARTESIAN_POINT('Origin',(78.0868516728187,191.282661304554,19.3713203435596)) ;
#77833=CARTESIAN_POINT('',(78.1546571314538,190.489539758744,19.2513203435596)) ;
#77834=CARTESIAN_POINT('Origin',(78.1546571314538,190.609539758744,19.2513203435596)) ;
#77835=CARTESIAN_POINT('Origin',(78.0776054738855,191.254450606202,19.2513203435596)) ;
#77836=CARTESIAN_POINT('Origin',(78.07353074889,190.609539758744,19.2513203435596)) ;
#77837=CARTESIAN_POINT('',(80.8501919227397,190.609539758744,19.3713203435596)) ;
#77838=CARTESIAN_POINT('',(80.8501919227397,190.489539758744,19.2513203435596)) ;
#77839=CARTESIAN_POINT('Origin',(80.8501919227397,190.609539758744,19.2513203435596)) ;
#77840=CARTESIAN_POINT('',(78.07353074889,190.489539758744,19.2513203435596)) ;
#77841=CARTESIAN_POINT('',(78.07353074889,190.609539758744,19.3713203435596)) ;
#77842=CARTESIAN_POINT('Ctrl Pts',(80.9810274260323,190.913160432898,19.3713203435596)) ;
#77843=CARTESIAN_POINT('Ctrl Pts',(80.9947301225928,190.898658010764,19.3713203435596)) ;
#77844=CARTESIAN_POINT('Ctrl Pts',(81.0287354417307,190.848346441009,19.3713203435596)) ;
#77845=CARTESIAN_POINT('Ctrl Pts',(81.0384684533216,190.7434130708,19.3713203435596)) ;
#77846=CARTESIAN_POINT('Ctrl Pts',(80.9697731322889,190.6371246451,19.3713203435596)) ;
#77847=CARTESIAN_POINT('Ctrl Pts',(80.8900960147986,190.609539758744,19.3713203435596)) ;
#77848=CARTESIAN_POINT('Ctrl Pts',(80.8501919227397,190.609539758744,19.3713203435596)) ;
#77849=CARTESIAN_POINT('Ctrl Pts',(81.0071246867289,190.937818579041,19.3713203435596)) ;
#77850=CARTESIAN_POINT('Ctrl Pts',(81.0235724505757,190.920410880242,19.3713203435596)) ;
#77851=CARTESIAN_POINT('Ctrl Pts',(81.064410508442,190.860067831628,19.3713203435596)) ;
#77852=CARTESIAN_POINT('Ctrl Pts',(81.0761224169453,190.734180607184,19.3713203435596)) ;
#77853=CARTESIAN_POINT('Ctrl Pts',(80.9936901648285,190.606657008059,19.3713203435596)) ;
#77854=CARTESIAN_POINT('Ctrl Pts',(80.8980900192786,190.573635842703,19.3713203435596)) ;
#77855=CARTESIAN_POINT('Ctrl Pts',(80.8501919227397,190.573635842703,19.3713203435596)) ;
#77856=CARTESIAN_POINT('Ctrl Pts',(81.0522866998738,190.980490165656,19.3411620218365)) ;
#77857=CARTESIAN_POINT('Ctrl Pts',(81.0734496812273,190.9580920568,19.3411620218365)) ;
#77858=CARTESIAN_POINT('Ctrl Pts',(81.1259638936544,190.880377438774,19.3411620218365)) ;
#77859=CARTESIAN_POINT('Ctrl Pts',(81.1409889173476,190.718297935341,19.3411620218365)) ;
#77860=CARTESIAN_POINT('Ctrl Pts',(81.0348871767947,190.5541280118,19.3411620218365)) ;
#77861=CARTESIAN_POINT('Ctrl Pts',(80.9118213657062,190.511503148125,19.3411620218365)) ;
#77862=CARTESIAN_POINT('Ctrl Pts',(80.8501919227397,190.511503148125,19.3411620218365)) ;
#77863=CARTESIAN_POINT('Ctrl Pts',(81.068251094894,190.995574215667,19.2782482805904)) ;
#77864=CARTESIAN_POINT('Ctrl Pts',(81.0910963470228,190.971395654268,19.2782482805904)) ;
#77865=CARTESIAN_POINT('Ctrl Pts',(81.147803117456,190.887545532474,19.2782482805904)) ;
#77866=CARTESIAN_POINT('Ctrl Pts',(81.1640483074976,190.71264204111,19.2782482805904)) ;
#77867=CARTESIAN_POINT('Ctrl Pts',(81.049534453483,190.53547320788,19.2782482805904)) ;
#77868=CARTESIAN_POINT('Ctrl Pts',(80.9167203640596,190.489539758744,19.2782482805904)) ;
#77869=CARTESIAN_POINT('Ctrl Pts',(80.8501919227397,190.489539758744,19.2782482805904)) ;
#77870=CARTESIAN_POINT('Ctrl Pts',(81.068251094894,190.995574215667,19.2513203435596)) ;
#77871=CARTESIAN_POINT('Ctrl Pts',(81.091088922495,190.971403512111,19.2513203435596)) ;
#77872=CARTESIAN_POINT('Ctrl Pts',(81.1477644543914,190.887550895852,19.2513203435596)) ;
#77873=CARTESIAN_POINT('Ctrl Pts',(81.1639861403761,190.712661945505,19.2513203435596)) ;
#77874=CARTESIAN_POINT('Ctrl Pts',(81.0494939386551,190.535514569337,19.2513203435596)) ;
#77875=CARTESIAN_POINT('Ctrl Pts',(80.9166987428378,190.489539758744,19.2513203435596)) ;
#77876=CARTESIAN_POINT('Ctrl Pts',(80.8501919227397,190.489539758744,19.2513203435596)) ;
#77877=CARTESIAN_POINT('',(80.9810274260323,190.913160432898,19.3713203435596)) ;
#77878=CARTESIAN_POINT('Ctrl Pts',(80.8501919227397,190.609539758744,19.3713203435596)) ;
#77879=CARTESIAN_POINT('Ctrl Pts',(80.8900960147986,190.609539758744,19.3713203435596)) ;
#77880=CARTESIAN_POINT('Ctrl Pts',(80.9697731322889,190.6371246451,19.3713203435596)) ;
#77881=CARTESIAN_POINT('Ctrl Pts',(81.0384684533216,190.7434130708,19.3713203435596)) ;
#77882=CARTESIAN_POINT('Ctrl Pts',(81.0287354417307,190.848346441009,19.3713203435596)) ;
#77883=CARTESIAN_POINT('Ctrl Pts',(80.9947301225928,190.898658010764,19.3713203435596)) ;
#77884=CARTESIAN_POINT('Ctrl Pts',(80.9810274260323,190.913160432898,19.3713203435596)) ;
#77885=CARTESIAN_POINT('',(81.068251094894,190.995574215667,19.2513203435596)) ;
#77886=CARTESIAN_POINT('Origin',(80.9810274260323,190.913160432898,19.2513203435596)) ;
#77887=CARTESIAN_POINT('Ctrl Pts',(81.068251094894,190.995574215667,19.2513203435596)) ;
#77888=CARTESIAN_POINT('Ctrl Pts',(81.1139288980579,190.947230535233,19.2513203435596)) ;
#77889=CARTESIAN_POINT('Ctrl Pts',(81.1716387139396,190.819103811481,19.2513203435596)) ;
#77890=CARTESIAN_POINT('Ctrl Pts',(81.1216272913293,190.614215808398,19.2513203435596)) ;
#77891=CARTESIAN_POINT('Ctrl Pts',(80.9833036543213,190.505926496137,19.2513203435596)) ;
#77892=CARTESIAN_POINT('Ctrl Pts',(80.8834468965772,190.489539758744,19.2513203435596)) ;
#77893=CARTESIAN_POINT('Ctrl Pts',(80.8501919227397,190.489539758744,19.2513203435596)) ;
#77894=CARTESIAN_POINT('Ctrl Pts',(81.068251094894,190.995574215666,19.2513203435596)) ;
#77895=CARTESIAN_POINT('Ctrl Pts',(78.3073761253817,193.917581142398,19.2513203435596)) ;
#77896=CARTESIAN_POINT('Ctrl Pts',(75.75172156108,197.052189907425,19.2513203435596)) ;
#77897=CARTESIAN_POINT('Ctrl Pts',(73.6915408905803,200.497421958395,19.2513203435596)) ;
#77898=CARTESIAN_POINT('Ctrl Pts',(81.068251094894,190.995574215666,19.2872242596007)) ;
#77899=CARTESIAN_POINT('Ctrl Pts',(78.3073899268033,193.917566535489,19.2872242596007)) ;
#77900=CARTESIAN_POINT('Ctrl Pts',(75.7517017249926,197.052223079236,19.2872242596007)) ;
#77901=CARTESIAN_POINT('Ctrl Pts',(73.6915408905803,200.497421958395,19.2872242596007)) ;
#77902=CARTESIAN_POINT('Ctrl Pts',(81.0463300781923,190.974862017566,19.3493569192823)) ;
#77903=CARTESIAN_POINT('Ctrl Pts',(78.2843665844062,193.898020997724,19.3493569192823)) ;
#77904=CARTESIAN_POINT('Ctrl Pts',(75.7274024340457,197.034095745875,19.3493569192823)) ;
#77905=CARTESIAN_POINT('Ctrl Pts',(73.6656572824995,200.48194407236,19.3493569192823)) ;
#77906=CARTESIAN_POINT('Ctrl Pts',(81.0006003715548,190.931654042505,19.3713203435596)) ;
#77907=CARTESIAN_POINT('Ctrl Pts',(78.2363739466475,193.857208024423,19.3713203435596)) ;
#77908=CARTESIAN_POINT('Ctrl Pts',(75.676658712843,196.996368164185,19.3713203435596)) ;
#77909=CARTESIAN_POINT('Ctrl Pts',(73.6116611645114,200.449655461051,19.3713203435596)) ;
#77910=CARTESIAN_POINT('Ctrl Pts',(80.9810274260323,190.913160432897,19.3713203435596)) ;
#77911=CARTESIAN_POINT('Ctrl Pts',(78.215833902103,193.839737956291,19.3713203435596)) ;
#77912=CARTESIAN_POINT('Ctrl Pts',(75.6549375918393,196.980223763859,19.3713203435596)) ;
#77913=CARTESIAN_POINT('Ctrl Pts',(73.5885500808522,200.43583548982,19.3713203435596)) ;
#77914=CARTESIAN_POINT('Ctrl Pts',(73.6915408905803,200.497421958395,19.2513203435596)) ;
#77915=CARTESIAN_POINT('Ctrl Pts',(75.75172156108,197.052189907425,19.2513203435596)) ;
#77916=CARTESIAN_POINT('Ctrl Pts',(78.3073761253817,193.917581142398,19.2513203435596)) ;
#77917=CARTESIAN_POINT('Ctrl Pts',(81.068251094894,190.995574215666,19.2513203435596)) ;
#77918=CARTESIAN_POINT('Ctrl Pts',(80.9810274260323,190.913160432897,19.3713203435596)) ;
#77919=CARTESIAN_POINT('Ctrl Pts',(78.215833902103,193.839737956291,19.3713203435596)) ;
#77920=CARTESIAN_POINT('Ctrl Pts',(75.6549375918393,196.980223763859,19.3713203435596)) ;
#77921=CARTESIAN_POINT('Ctrl Pts',(73.5885500808522,200.43583548982,19.3713203435596)) ;
#77922=CARTESIAN_POINT('Ctrl Pts',(67.8715456014017,200.55583548982,17.9913203435596)) ;
#77923=CARTESIAN_POINT('Ctrl Pts',(67.8466022358902,200.55583548982,17.9913203435596)) ;
#77924=CARTESIAN_POINT('Ctrl Pts',(67.8093588147496,200.543700298089,17.9913203435596)) ;
#77925=CARTESIAN_POINT('Ctrl Pts',(67.7643817760585,200.499332389917,17.9913203435596)) ;
#77926=CARTESIAN_POINT('Ctrl Pts',(67.7435398814255,200.437381726819,17.9913203435596)) ;
#77927=CARTESIAN_POINT('Ctrl Pts',(67.7589874071544,200.387329568627,17.9913203435596)) ;
#77928=CARTESIAN_POINT('Ctrl Pts',(67.7733141381135,200.366911041181,17.9913203435596)) ;
#77929=CARTESIAN_POINT('Ctrl Pts',(67.8715456014017,200.55583548982,17.9554164275186)) ;
#77930=CARTESIAN_POINT('Ctrl Pts',(67.8466819509688,200.55583548982,17.9554164275186)) ;
#77931=CARTESIAN_POINT('Ctrl Pts',(67.8094573381231,200.543546439635,17.9554164275186)) ;
#77932=CARTESIAN_POINT('Ctrl Pts',(67.764591266304,200.499257277487,17.9554164275186)) ;
#77933=CARTESIAN_POINT('Ctrl Pts',(67.7437368491879,200.437352434046,17.9554164275186)) ;
#77934=CARTESIAN_POINT('Ctrl Pts',(67.7590331931363,200.38726431422,17.9554164275186)) ;
#77935=CARTESIAN_POINT('Ctrl Pts',(67.7733141381135,200.366911041181,17.9554164275186)) ;
#77936=CARTESIAN_POINT('Ctrl Pts',(67.8715456014017,200.585993742446,17.8932836500338)) ;
#77937=CARTESIAN_POINT('Ctrl Pts',(67.84031507213,200.585993742446,17.8932836500338)) ;
#77938=CARTESIAN_POINT('Ctrl Pts',(67.7937073322049,200.570844316766,17.8932836500338)) ;
#77939=CARTESIAN_POINT('Ctrl Pts',(67.7374010671215,200.515307716645,17.8932836500337)) ;
#77940=CARTESIAN_POINT('Ctrl Pts',(67.7113241079541,200.437777096827,17.8932836500338)) ;
#77941=CARTESIAN_POINT('Ctrl Pts',(67.7306888356429,200.375154204976,17.8932836500338)) ;
#77942=CARTESIAN_POINT('Ctrl Pts',(67.7486267273993,200.349589033396,17.8932836500338)) ;
#77943=CARTESIAN_POINT('Ctrl Pts',(67.8715456014017,200.648907552789,17.8713203435596)) ;
#77944=CARTESIAN_POINT('Ctrl Pts',(67.8272446988906,200.648907552789,17.8713203435596)) ;
#77945=CARTESIAN_POINT('Ctrl Pts',(67.7611125593011,200.62738239895,17.8713203435596)) ;
#77946=CARTESIAN_POINT('Ctrl Pts',(67.6812353674285,200.548591407486,17.8713203435596)) ;
#77947=CARTESIAN_POINT('Ctrl Pts',(67.6442302870083,200.43858519642,17.8713203435596)) ;
#77948=CARTESIAN_POINT('Ctrl Pts',(67.671680636309,200.349717723304,17.8713203435596)) ;
#77949=CARTESIAN_POINT('Ctrl Pts',(67.6971257636407,200.313453202648,17.8713203435596)) ;
#77950=CARTESIAN_POINT('Ctrl Pts',(67.8715456014017,200.67583548982,17.8713203435596)) ;
#77951=CARTESIAN_POINT('Ctrl Pts',(67.8216588703786,200.67583548982,17.8713203435596)) ;
#77952=CARTESIAN_POINT('Ctrl Pts',(67.7471720280976,200.651565106359,17.8713203435596)) ;
#77953=CARTESIAN_POINT('Ctrl Pts',(67.6572179507153,200.562829290015,17.8713203435596)) ;
#77954=CARTESIAN_POINT('Ctrl Pts',(67.6155341614493,200.438927963818,17.8713203435596)) ;
#77955=CARTESIAN_POINT('Ctrl Pts',(67.646429212907,200.338823647433,17.8713203435596)) ;
#77956=CARTESIAN_POINT('Ctrl Pts',(67.6750826748252,200.297986592541,17.8713203435596)) ;
#77957=CARTESIAN_POINT('',(67.654399260129,200.537671106355,17.8713203435596)) ;
#77958=CARTESIAN_POINT('',(67.6638006826676,200.555777405267,17.8713203435596)) ;
#77959=CARTESIAN_POINT('Origin',(67.8164545295421,200.45482568124,17.8713203435596)) ;
#77960=CARTESIAN_POINT('',(67.8715456014017,200.67583548982,17.8713203435596)) ;
#77961=CARTESIAN_POINT('Ctrl Pts',(67.6638006825543,200.55577740507,17.8713203435596)) ;
#77962=CARTESIAN_POINT('Ctrl Pts',(67.6682504093187,200.563528431557,17.8713203435596)) ;
#77963=CARTESIAN_POINT('Ctrl Pts',(67.686751282339,200.59196264747,17.8713203435596)) ;
#77964=CARTESIAN_POINT('Ctrl Pts',(67.7471720280976,200.651565106359,17.8713203435596)) ;
#77965=CARTESIAN_POINT('Ctrl Pts',(67.8216588703786,200.67583548982,17.8713203435596)) ;
#77966=CARTESIAN_POINT('Ctrl Pts',(67.8715456014017,200.67583548982,17.8713203435596)) ;
#77967=CARTESIAN_POINT('',(67.8715456014017,200.55583548982,17.9913203435596)) ;
#77968=CARTESIAN_POINT('Origin',(67.8715456014017,200.67583548982,17.9913203435596)) ;
#77969=CARTESIAN_POINT('',(67.7733141381135,200.366911041181,17.9913203435596)) ;
#77970=CARTESIAN_POINT('Ctrl Pts',(67.8715456014017,200.55583548982,17.9913203435596)) ;
#77971=CARTESIAN_POINT('Ctrl Pts',(67.8528373343895,200.55583548982,17.9913203435596)) ;
#77972=CARTESIAN_POINT('Ctrl Pts',(67.8091125279312,200.54551389311,17.9913203435596)) ;
#77973=CARTESIAN_POINT('Ctrl Pts',(67.7626667658301,200.499540877992,17.9913203435596)) ;
#77974=CARTESIAN_POINT('Ctrl Pts',(67.7455875249419,200.431050106803,17.9913203435596)) ;
#77975=CARTESIAN_POINT('Ctrl Pts',(67.7589868382377,200.387330379449,17.9913203435596)) ;
#77976=CARTESIAN_POINT('Ctrl Pts',(67.7733141381135,200.366911041181,17.9913203435596)) ;
#77977=CARTESIAN_POINT('',(67.6750826748252,200.297986592541,17.8713203435596)) ;
#77978=CARTESIAN_POINT('Origin',(67.6750826748252,200.297986592541,17.9913203435596)) ;
#77979=CARTESIAN_POINT('Ctrl Pts',(67.6750826748252,200.297986592541,17.8713203435596)) ;
#77980=CARTESIAN_POINT('Ctrl Pts',(67.646429212907,200.338823647433,17.8713203435596)) ;
#77981=CARTESIAN_POINT('Ctrl Pts',(67.6204094720538,200.423131271072,17.8713203435596)) ;
#77982=CARTESIAN_POINT('Ctrl Pts',(67.6399564441711,200.506741474643,17.8713203435596)) ;
#77983=CARTESIAN_POINT('Ctrl Pts',(67.6543992598854,200.537671105833,17.8713203435596)) ;
#77984=CARTESIAN_POINT('Ctrl Pts',(67.7733141381135,200.366911041181,17.9913203435596)) ;
#77985=CARTESIAN_POINT('Ctrl Pts',(67.7733141381135,200.366911041181,19.5033203435596)) ;
#77986=CARTESIAN_POINT('Ctrl Pts',(67.7589868382377,200.387330379449,17.9913203435596)) ;
#77987=CARTESIAN_POINT('Ctrl Pts',(67.7589868382377,200.387330379449,19.5033203435596)) ;
#77988=CARTESIAN_POINT('Ctrl Pts',(67.7455875249419,200.431050106803,17.9913203435596)) ;
#77989=CARTESIAN_POINT('Ctrl Pts',(67.7455875249419,200.431050106803,19.5033203435596)) ;
#77990=CARTESIAN_POINT('Ctrl Pts',(67.7626667658301,200.499540877992,17.9913203435596)) ;
#77991=CARTESIAN_POINT('Ctrl Pts',(67.7626667658301,200.499540877992,19.5033203435596)) ;
#77992=CARTESIAN_POINT('Ctrl Pts',(67.8091125279312,200.54551389311,17.9913203435596)) ;
#77993=CARTESIAN_POINT('Ctrl Pts',(67.8091125279312,200.54551389311,19.5033203435596)) ;
#77994=CARTESIAN_POINT('Ctrl Pts',(67.8528373343895,200.55583548982,17.9913203435596)) ;
#77995=CARTESIAN_POINT('Ctrl Pts',(67.8528373343895,200.55583548982,19.5033203435596)) ;
#77996=CARTESIAN_POINT('Ctrl Pts',(67.8715456014017,200.55583548982,17.9913203435596)) ;
#77997=CARTESIAN_POINT('Ctrl Pts',(67.8715456014017,200.55583548982,19.5033203435596)) ;
#77998=CARTESIAN_POINT('',(67.7733141381135,200.366911041181,19.2513203435596)) ;
#77999=CARTESIAN_POINT('',(67.8715456014017,200.55583548982,17.9913203435596)) ;
#78000=CARTESIAN_POINT('Ctrl Pts',(67.7733141381135,200.366911041181,17.9913203435596)) ;
#78001=CARTESIAN_POINT('Ctrl Pts',(70.4189965819413,196.596271406283,17.9913203435596)) ;
#78002=CARTESIAN_POINT('Ctrl Pts',(73.8443753644747,193.414315549682,17.9913203435596)) ;
#78003=CARTESIAN_POINT('Ctrl Pts',(77.5627334640076,190.683545731522,17.9913203435596)) ;
#78004=CARTESIAN_POINT('Ctrl Pts',(67.7733141381135,200.366911041181,17.9554164275186)) ;
#78005=CARTESIAN_POINT('Ctrl Pts',(70.4189655115399,196.596315687972,17.9554164275186)) ;
#78006=CARTESIAN_POINT('Ctrl Pts',(73.8444003768411,193.414297180549,17.9554164275186)) ;
#78007=CARTESIAN_POINT('Ctrl Pts',(77.5627334640076,190.683545731522,17.9554164275186)) ;
#78008=CARTESIAN_POINT('Ctrl Pts',(67.7486267295111,200.349589034877,17.8932836469385)) ;
#78009=CARTESIAN_POINT('Ctrl Pts',(70.3967597097377,196.575456883448,17.8932836469385)) ;
#78010=CARTESIAN_POINT('Ctrl Pts',(73.8245512460258,193.39145696199,17.8932836469385)) ;
#78011=CARTESIAN_POINT('Ctrl Pts',(77.5448820820363,190.659238362113,17.8932836469385)) ;
#78012=CARTESIAN_POINT('Ctrl Pts',(67.6971257636408,200.313453202648,17.8713203435596)) ;
#78013=CARTESIAN_POINT('Ctrl Pts',(70.3503531595038,196.532060464991,17.8713203435596)) ;
#78014=CARTESIAN_POINT('Ctrl Pts',(73.7832099528935,193.343760674206,17.8713203435596)) ;
#78015=CARTESIAN_POINT('Ctrl Pts',(77.5076419071581,190.608530204668,17.8713203435596)) ;
#78016=CARTESIAN_POINT('Ctrl Pts',(67.6750826748252,200.297986592541,17.8713203435596)) ;
#78017=CARTESIAN_POINT('Ctrl Pts',(70.3304872489213,196.513490929755,17.8713203435596)) ;
#78018=CARTESIAN_POINT('Ctrl Pts',(73.7655179925946,193.323344087419,17.8713203435596)) ;
#78019=CARTESIAN_POINT('Ctrl Pts',(77.4917026239141,190.586826448256,17.8713203435596)) ;
#78020=CARTESIAN_POINT('',(77.5627334640076,190.683545731522,17.9913203435596)) ;
#78021=CARTESIAN_POINT('Ctrl Pts',(67.7733141381135,200.366911041181,17.9913203435596)) ;
#78022=CARTESIAN_POINT('Ctrl Pts',(70.4189965819413,196.596271406283,17.9913203435596)) ;
#78023=CARTESIAN_POINT('Ctrl Pts',(73.8443753644747,193.414315549682,17.9913203435596)) ;
#78024=CARTESIAN_POINT('Ctrl Pts',(77.5627334640076,190.683545731522,17.9913203435596)) ;
#78025=CARTESIAN_POINT('',(77.4917026239141,190.586826448256,17.8713203435596)) ;
#78026=CARTESIAN_POINT('Origin',(77.4917026239141,190.586826448256,17.9913203435596)) ;
#78027=CARTESIAN_POINT('Ctrl Pts',(77.4917026239141,190.586826448256,17.8713203435596)) ;
#78028=CARTESIAN_POINT('Ctrl Pts',(73.7655179925946,193.323344087419,17.8713203435596)) ;
#78029=CARTESIAN_POINT('Ctrl Pts',(70.3304872489213,196.513490929755,17.8713203435596)) ;
#78030=CARTESIAN_POINT('Ctrl Pts',(67.6750826748252,200.297986592541,17.8713203435596)) ;
#78031=CARTESIAN_POINT('Ctrl Pts',(78.1546571314538,190.369539758744,17.8713203435596)) ;
#78032=CARTESIAN_POINT('Ctrl Pts',(77.9181765170877,190.369539758744,17.8713203435596)) ;
#78033=CARTESIAN_POINT('Ctrl Pts',(77.6823045866469,190.44684797572,17.8713203435596)) ;
#78034=CARTESIAN_POINT('Ctrl Pts',(77.4917026239141,190.586826448256,17.8713203435596)) ;
#78035=CARTESIAN_POINT('Ctrl Pts',(78.1546571314538,190.405443674785,17.8713203435596)) ;
#78036=CARTESIAN_POINT('Ctrl Pts',(77.9257902384857,190.405443674785,17.8713203435596)) ;
#78037=CARTESIAN_POINT('Ctrl Pts',(77.6974203503338,190.480293059496,17.8713203435596)) ;
#78038=CARTESIAN_POINT('Ctrl Pts',(77.5129550015728,190.615764790139,17.8713203435596)) ;
#78039=CARTESIAN_POINT('Ctrl Pts',(78.1546571314538,190.467576448569,17.9014785992702)) ;
#78040=CARTESIAN_POINT('Ctrl Pts',(77.9388683705259,190.467576448569,17.9014785992702)) ;
#78041=CARTESIAN_POINT('Ctrl Pts',(77.7236573133492,190.538112959941,17.9014785992701)) ;
#78042=CARTESIAN_POINT('Ctrl Pts',(77.5497328608997,190.665843434703,17.9014785992701)) ;
#78043=CARTESIAN_POINT('Ctrl Pts',(78.1546571314538,190.489539758744,17.9643924065289)) ;
#78044=CARTESIAN_POINT('Ctrl Pts',(77.9435343184478,190.489539758744,17.9643924065289)) ;
#78045=CARTESIAN_POINT('Ctrl Pts',(77.7328971903008,190.558577141766,17.9643924065289)) ;
#78046=CARTESIAN_POINT('Ctrl Pts',(77.5627334640076,190.683545731522,17.9643924065289)) ;
#78047=CARTESIAN_POINT('Ctrl Pts',(78.1546571314538,190.489539758744,17.9913203435596)) ;
#78048=CARTESIAN_POINT('Ctrl Pts',(77.94351372577,190.489539758744,17.9913203435596)) ;
#78049=CARTESIAN_POINT('Ctrl Pts',(77.7329137878761,190.558564952473,17.9913203435596)) ;
#78050=CARTESIAN_POINT('Ctrl Pts',(77.5627334640076,190.683545731522,17.9913203435596)) ;
#78051=CARTESIAN_POINT('',(78.1546571314538,190.489539758744,17.9913203435596)) ;
#78052=CARTESIAN_POINT('Origin',(78.0776054738942,191.254450606233,17.9913203435596)) ;
#78053=CARTESIAN_POINT('',(78.1546571314538,190.369539758744,17.8713203435596)) ;
#78054=CARTESIAN_POINT('Origin',(78.1546571314538,190.369539758744,17.9913203435596)) ;
#78055=CARTESIAN_POINT('Origin',(78.0683592750173,191.22623990799,17.8713203435596)) ;
#78056=CARTESIAN_POINT('Origin',(73.6548295654295,190.369539758744,17.9913203435596)) ;
#78057=CARTESIAN_POINT('',(80.8501919227397,190.489539758744,17.9913203435596)) ;
#78058=CARTESIAN_POINT('',(80.8501919227397,190.369539758744,17.8713203435596)) ;
#78059=CARTESIAN_POINT('Origin',(80.8501919227397,190.369539758744,17.9913203435596)) ;
#78060=CARTESIAN_POINT('',(73.6548295654295,190.369539758744,17.8713203435596)) ;
#78061=CARTESIAN_POINT('',(73.6548295654295,190.489539758744,17.9913203435596)) ;
#78062=CARTESIAN_POINT('Ctrl Pts',(81.1554747637557,191.077987998436,17.8713203435596)) ;
#78063=CARTESIAN_POINT('Ctrl Pts',(81.2513936396798,190.976471043503,17.8713203435596)) ;
#78064=CARTESIAN_POINT('Ctrl Pts',(81.316638910935,190.723383706498,17.8713203435596)) ;
#78065=CARTESIAN_POINT('Ctrl Pts',(81.1283155314175,190.433679019485,17.8713203435596)) ;
#78066=CARTESIAN_POINT('Ctrl Pts',(80.9433014708773,190.369539758744,17.8713203435596)) ;
#78067=CARTESIAN_POINT('Ctrl Pts',(80.8501919227397,190.369539758744,17.8713203435596)) ;
#78068=CARTESIAN_POINT('Ctrl Pts',(81.129377503059,191.053329852293,17.8713203435596)) ;
#78069=CARTESIAN_POINT('Ctrl Pts',(81.2170611771247,190.960528727356,17.8713203435596)) ;
#78070=CARTESIAN_POINT('Ctrl Pts',(81.2766261409266,190.728987825454,17.8713203435596)) ;
#78071=CARTESIAN_POINT('Ctrl Pts',(81.1044711159146,190.464155266563,17.8713203435596)) ;
#78072=CARTESIAN_POINT('Ctrl Pts',(80.9353074663972,190.405443674785,17.8713203435596)) ;
#78073=CARTESIAN_POINT('Ctrl Pts',(80.8501919227397,190.405443674785,17.8713203435596)) ;
#78074=CARTESIAN_POINT('Ctrl Pts',(81.0842154748565,191.01065825145,17.9014786480176)) ;
#78075=CARTESIAN_POINT('Ctrl Pts',(81.1577534964021,190.932828356686,17.9014786480176)) ;
#78076=CARTESIAN_POINT('Ctrl Pts',(81.2077940098548,190.738838272952,17.9014786480176)) ;
#78077=CARTESIAN_POINT('Ctrl Pts',(81.0634124040283,190.51673086814,17.9014786480176)) ;
#78078=CARTESIAN_POINT('Ctrl Pts',(80.9215761199696,190.467576390079,17.9014786480176)) ;
#78079=CARTESIAN_POINT('Ctrl Pts',(80.8501919227397,190.467576390079,17.9014786480176)) ;
#78080=CARTESIAN_POINT('Ctrl Pts',(81.068251094894,190.995574215667,17.9643924065289)) ;
#78081=CARTESIAN_POINT('Ctrl Pts',(81.1367423041135,190.923085678529,17.9643924065289)) ;
#78082=CARTESIAN_POINT('Ctrl Pts',(81.1832816311425,190.742253295466,17.9643924065289)) ;
#78083=CARTESIAN_POINT('Ctrl Pts',(81.0488084622043,190.535388191718,17.9643924065289)) ;
#78084=CARTESIAN_POINT('Ctrl Pts',(80.9166771216162,190.489539758744,17.9643924065289)) ;
#78085=CARTESIAN_POINT('Ctrl Pts',(80.8501919227397,190.489539758744,17.9643924065289)) ;
#78086=CARTESIAN_POINT('Ctrl Pts',(81.068251094894,190.995574215667,17.9913203435596)) ;
#78087=CARTESIAN_POINT('Ctrl Pts',(81.1367645776969,190.923062105,17.9913203435596)) ;
#78088=CARTESIAN_POINT('Ctrl Pts',(81.1833683428792,190.742285435711,17.9913203435596)) ;
#78089=CARTESIAN_POINT('Ctrl Pts',(81.0488516432238,190.535353516416,17.9913203435596)) ;
#78090=CARTESIAN_POINT('Ctrl Pts',(80.916698742838,190.489539758744,17.9913203435596)) ;
#78091=CARTESIAN_POINT('Ctrl Pts',(80.8501919227397,190.489539758744,17.9913203435596)) ;
#78092=CARTESIAN_POINT('',(81.068251094894,190.995574215667,17.9913203435596)) ;
#78093=CARTESIAN_POINT('Ctrl Pts',(80.8501919227397,190.489539758744,17.9913203435596)) ;
#78094=CARTESIAN_POINT('Ctrl Pts',(80.916698742838,190.489539758744,17.9913203435596)) ;
#78095=CARTESIAN_POINT('Ctrl Pts',(81.0488516432238,190.535353516416,17.9913203435596)) ;
#78096=CARTESIAN_POINT('Ctrl Pts',(81.1833683428792,190.742285435711,17.9913203435596)) ;
#78097=CARTESIAN_POINT('Ctrl Pts',(81.1367645776969,190.923062105,17.9913203435596)) ;
#78098=CARTESIAN_POINT('Ctrl Pts',(81.068251094894,190.995574215667,17.9913203435596)) ;
#78099=CARTESIAN_POINT('',(81.1554747637557,191.077987998436,17.8713203435596)) ;
#78100=CARTESIAN_POINT('Origin',(81.1554747637557,191.077987998436,17.9913203435596)) ;
#78101=CARTESIAN_POINT('Ctrl Pts',(81.1554747637557,191.077987998436,17.8713203435596)) ;
#78102=CARTESIAN_POINT('Ctrl Pts',(81.2513936396798,190.976471043503,17.8713203435596)) ;
#78103=CARTESIAN_POINT('Ctrl Pts',(81.316638910935,190.723383706498,17.8713203435596)) ;
#78104=CARTESIAN_POINT('Ctrl Pts',(81.1283155314175,190.433679019485,17.8713203435596)) ;
#78105=CARTESIAN_POINT('Ctrl Pts',(80.9433014708773,190.369539758744,17.8713203435596)) ;
#78106=CARTESIAN_POINT('Ctrl Pts',(80.8501919227397,190.369539758744,17.8713203435596)) ;
#78107=CARTESIAN_POINT('Ctrl Pts',(81.068251094894,190.995574215667,17.9913203435596)) ;
#78108=CARTESIAN_POINT('Ctrl Pts',(78.3107281673276,193.914033466429,17.9913203435596)) ;
#78109=CARTESIAN_POINT('Ctrl Pts',(75.7551903021708,197.046389145311,17.9913203435596)) ;
#78110=CARTESIAN_POINT('Ctrl Pts',(73.6915408905803,200.497421958395,17.9913203435596)) ;
#78111=CARTESIAN_POINT('Ctrl Pts',(81.068251094894,190.995574215667,17.9554164275186)) ;
#78112=CARTESIAN_POINT('Ctrl Pts',(78.3107143826626,193.914048055604,17.9554164275186)) ;
#78113=CARTESIAN_POINT('Ctrl Pts',(75.7552101716563,197.046355917648,17.9554164275186)) ;
#78114=CARTESIAN_POINT('Ctrl Pts',(73.6915408905803,200.497421958395,17.9554164275186)) ;
#78115=CARTESIAN_POINT('Ctrl Pts',(81.0901720991602,191.016286402018,17.8932837473092)) ;
#78116=CARTESIAN_POINT('Ctrl Pts',(78.3337363742652,193.933594998089,17.8932837473092)) ;
#78117=CARTESIAN_POINT('Ctrl Pts',(75.7795067803935,197.064487703123,17.8932837473092)) ;
#78118=CARTESIAN_POINT('Ctrl Pts',(73.7174244839775,200.51289983565,17.8932837473092)) ;
#78119=CARTESIAN_POINT('Ctrl Pts',(81.1359018182332,191.059494388828,17.8713203435596)) ;
#78120=CARTESIAN_POINT('Ctrl Pts',(78.3817262769825,193.974410890966,17.8713203435596)) ;
#78121=CARTESIAN_POINT('Ctrl Pts',(75.8302450401957,197.102224451227,17.8713203435596)) ;
#78122=CARTESIAN_POINT('Ctrl Pts',(73.7714206166491,200.545188455739,17.8713203435596)) ;
#78123=CARTESIAN_POINT('Ctrl Pts',(81.1554747637557,191.077987998436,17.8713203435596)) ;
#78124=CARTESIAN_POINT('Ctrl Pts',(78.4022651473499,193.991882201803,17.8713203435596)) ;
#78125=CARTESIAN_POINT('Ctrl Pts',(75.8519638209093,197.118372765211,17.8713203435596)) ;
#78126=CARTESIAN_POINT('Ctrl Pts',(73.7945317003083,200.55900842697,17.8713203435596)) ;
#78127=CARTESIAN_POINT('Ctrl Pts',(73.7945317003083,200.55900842697,17.8713203435596)) ;
#78128=CARTESIAN_POINT('Ctrl Pts',(75.8519638209093,197.118372765211,17.8713203435596)) ;
#78129=CARTESIAN_POINT('Ctrl Pts',(78.4022651473499,193.991882201803,17.8713203435596)) ;
#78130=CARTESIAN_POINT('Ctrl Pts',(81.1554747637557,191.077987998436,17.8713203435596)) ;
#78131=CARTESIAN_POINT('Ctrl Pts',(81.068251094894,190.995574215667,17.9913203435596)) ;
#78132=CARTESIAN_POINT('Ctrl Pts',(78.3107281673276,193.914033466429,17.9913203435596)) ;
#78133=CARTESIAN_POINT('Ctrl Pts',(75.7551903021708,197.046389145311,17.9913203435596)) ;
#78134=CARTESIAN_POINT('Ctrl Pts',(73.6915408905803,200.497421958395,17.9913203435596)) ;
#78135=CARTESIAN_POINT('Origin',(66.7003418520632,200.67583548982,17.9913203435596)) ;
#78136=CARTESIAN_POINT('',(66.7003418520632,200.67583548982,17.8713203435596)) ;
#78137=CARTESIAN_POINT('',(66.7003418520632,200.55583548982,17.9913203435596)) ;
#78138=CARTESIAN_POINT('Ctrl Pts',(81.068251094894,190.995574215667,17.9913203435596)) ;
#78139=CARTESIAN_POINT('Ctrl Pts',(81.068251094894,190.995574215667,19.5033203435596)) ;
#78140=CARTESIAN_POINT('Ctrl Pts',(81.1139288980579,190.947230535233,17.9913203435596)) ;
#78141=CARTESIAN_POINT('Ctrl Pts',(81.1139288980579,190.947230535233,19.5033203435596)) ;
#78142=CARTESIAN_POINT('Ctrl Pts',(81.1716387139396,190.819103811481,17.9913203435596)) ;
#78143=CARTESIAN_POINT('Ctrl Pts',(81.1716387139396,190.819103811481,19.5033203435596)) ;
#78144=CARTESIAN_POINT('Ctrl Pts',(81.1216272913293,190.614215808398,17.9913203435596)) ;
#78145=CARTESIAN_POINT('Ctrl Pts',(81.1216272913293,190.614215808398,19.5033203435596)) ;
#78146=CARTESIAN_POINT('Ctrl Pts',(80.9833036543213,190.505926496137,17.9913203435596)) ;
#78147=CARTESIAN_POINT('Ctrl Pts',(80.9833036543213,190.505926496137,19.5033203435596)) ;
#78148=CARTESIAN_POINT('Ctrl Pts',(80.8834468965772,190.489539758744,17.9913203435596)) ;
#78149=CARTESIAN_POINT('Ctrl Pts',(80.8834468965772,190.489539758744,19.5033203435596)) ;
#78150=CARTESIAN_POINT('Ctrl Pts',(80.8501919227397,190.489539758744,17.9913203435596)) ;
#78151=CARTESIAN_POINT('Ctrl Pts',(80.8501919227397,190.489539758744,19.5033203435596)) ;
#78152=CARTESIAN_POINT('',(80.8501919227397,190.489539758744,17.9913203435596)) ;
#78153=CARTESIAN_POINT('',(81.068251094894,190.995574215667,19.2513203435596)) ;
#78154=CARTESIAN_POINT('Ctrl Pts',(77.8285014478222,190.489539758744,17.8547522895864)) ;
#78155=CARTESIAN_POINT('Ctrl Pts',(77.8285014478222,190.489539758744,32.8746339543542)) ;
#78156=CARTESIAN_POINT('Ctrl Pts',(73.8355349189945,193.386814152385,17.8547522895863)) ;
#78157=CARTESIAN_POINT('Ctrl Pts',(73.8355349189945,193.386814152385,32.8746339543541)) ;
#78158=CARTESIAN_POINT('Ctrl Pts',(70.4532522157592,196.594204259059,17.8547522895864)) ;
#78159=CARTESIAN_POINT('Ctrl Pts',(70.4532522157592,196.594204259059,32.8746339543542)) ;
#78160=CARTESIAN_POINT('Ctrl Pts',(67.88518965836,200.208466979566,17.8547522895864)) ;
#78161=CARTESIAN_POINT('Ctrl Pts',(67.88518965836,200.208466979566,32.8746339543542)) ;
#78162=CARTESIAN_POINT('Ctrl Pts',(67.8032385132701,200.323804110956,17.8547522895864)) ;
#78163=CARTESIAN_POINT('Ctrl Pts',(67.8032385132701,200.323804110956,32.8746339543542)) ;
#78164=CARTESIAN_POINT('Ctrl Pts',(67.7220901562832,200.439592363042,17.8547522895864)) ;
#78165=CARTESIAN_POINT('Ctrl Pts',(67.7220901562832,200.439592363042,32.8746339543542)) ;
#78166=CARTESIAN_POINT('Ctrl Pts',(67.6417475736103,200.555835489811,17.8547522895864)) ;
#78167=CARTESIAN_POINT('Ctrl Pts',(67.6417475736103,200.555835489811,32.8746339543542)) ;
#78168=CARTESIAN_POINT('',(77.5627334640076,190.683545731522,17.9913203435596)) ;
#78169=CARTESIAN_POINT('Origin',(81.5507230003364,190.489539758744,23.8713203435596)) ;
#78170=CARTESIAN_POINT('',(78.1546571314538,190.489539758744,19.2513203435596)) ;
#78171=CARTESIAN_POINT('Ctrl Pts',(78.1546571314538,190.489539758744,17.9913203435596)) ;
#78172=CARTESIAN_POINT('Ctrl Pts',(78.1546571314538,190.489539758744,19.5033203435596)) ;
#78173=CARTESIAN_POINT('Ctrl Pts',(77.9435093125031,190.489539758744,17.9913203435596)) ;
#78174=CARTESIAN_POINT('Ctrl Pts',(77.9435093125031,190.489539758744,19.5033203435596)) ;
#78175=CARTESIAN_POINT('Ctrl Pts',(77.7329173449427,190.558562340156,17.9913203435596)) ;
#78176=CARTESIAN_POINT('Ctrl Pts',(77.7329173449427,190.558562340156,19.5033203435596)) ;
#78177=CARTESIAN_POINT('Ctrl Pts',(77.5627334640076,190.683545731522,17.9913203435596)) ;
#78178=CARTESIAN_POINT('Ctrl Pts',(77.5627334640076,190.683545731522,19.5033203435596)) ;
#78179=CARTESIAN_POINT('Origin',(65.7589361305225,212.963038649314,17.8713203435596)) ;
#78180=CARTESIAN_POINT('',(60.9557289922431,214.062457733496,17.8713203435596)) ;
#78181=CARTESIAN_POINT('',(61.2615982170329,212.685341204933,17.8713203435596)) ;
#78182=CARTESIAN_POINT('Origin',(186.600966963329,306.450327238289,17.8713203435596)) ;
#78183=CARTESIAN_POINT('',(70.2265094709067,213.162319271896,17.8713203435596)) ;
#78184=CARTESIAN_POINT('',(67.5325794977657,213.423884085911,17.8713203435596)) ;
#78185=CARTESIAN_POINT('',(70.3877178199639,213.005540169192,17.8713203435596)) ;
#78186=CARTESIAN_POINT('Ctrl Pts',(70.3877178199639,213.005540169192,17.8713203435596)) ;
#78187=CARTESIAN_POINT('Ctrl Pts',(70.3834041808396,213.039967616326,17.8713203435596)) ;
#78188=CARTESIAN_POINT('Ctrl Pts',(70.3494702400649,213.117382991064,17.8713203435596)) ;
#78189=CARTESIAN_POINT('Ctrl Pts',(70.2725551198838,213.157848509207,17.8713203435596)) ;
#78190=CARTESIAN_POINT('Ctrl Pts',(70.2265094709067,213.162319271896,17.8713203435596)) ;
#78191=CARTESIAN_POINT('',(74.071363112532,201.997275065426,17.8713203435596)) ;
#78192=CARTESIAN_POINT('Ctrl Pts',(74.0713631125318,201.997275065426,17.8713203435596)) ;
#78193=CARTESIAN_POINT('Ctrl Pts',(72.9854321297061,203.939567940643,17.8713203435596)) ;
#78194=CARTESIAN_POINT('Ctrl Pts',(71.4053737386935,207.523894544389,17.8713203435596)) ;
#78195=CARTESIAN_POINT('Ctrl Pts',(70.5952077140308,211.34954921747,17.8713203435596)) ;
#78196=CARTESIAN_POINT('Ctrl Pts',(70.3877178199639,213.005540169192,17.8713203435596)) ;
#78197=CARTESIAN_POINT('',(83.4878143389934,190.058573545737,17.8713203435596)) ;
#78198=CARTESIAN_POINT('Ctrl Pts',(83.4878143389934,190.058573545737,17.8713203435596)) ;
#78199=CARTESIAN_POINT('Ctrl Pts',(81.4305821636459,192.110706612955,17.8713203435596)) ;
#78200=CARTESIAN_POINT('Ctrl Pts',(78.0106503827396,195.884693008864,17.8713203435596)) ;
#78201=CARTESIAN_POINT('Ctrl Pts',(75.1348798094609,200.095072314249,17.8713203435596)) ;
#78202=CARTESIAN_POINT('Ctrl Pts',(74.071363112532,201.997275065426,17.8713203435596)) ;
#78203=CARTESIAN_POINT('',(83.2194473860051,189.409539758744,17.8713203435596)) ;
#78204=CARTESIAN_POINT('Ctrl Pts',(83.2194473860051,189.409539758744,17.8713203435596)) ;
#78205=CARTESIAN_POINT('Ctrl Pts',(83.3047606779792,189.409539758744,17.8713203435596)) ;
#78206=CARTESIAN_POINT('Ctrl Pts',(83.4319242412693,189.454563257398,17.8713203435596)) ;
#78207=CARTESIAN_POINT('Ctrl Pts',(83.5764307889551,189.615888430006,17.8713203435596)) ;
#78208=CARTESIAN_POINT('Ctrl Pts',(83.6266013556018,189.835500488137,17.8713203435596)) ;
#78209=CARTESIAN_POINT('Ctrl Pts',(83.5482147548371,189.998322839904,17.8713203435596)) ;
#78210=CARTESIAN_POINT('Ctrl Pts',(83.4878143389934,190.058573545737,17.8713203435596)) ;
#78211=CARTESIAN_POINT('',(77.8285014478222,189.409539758744,17.8713203435596)) ;
#78212=CARTESIAN_POINT('',(71.6000791389318,189.409539758744,17.8713203435596)) ;
#78213=CARTESIAN_POINT('',(77.1942359127805,189.615407485539,17.8713203435596)) ;
#78214=CARTESIAN_POINT('Origin',(77.7459982214612,190.235352500613,17.8713203435596)) ;
#78215=CARTESIAN_POINT('',(66.2956301826422,200.621620147878,17.8713203435596)) ;
#78216=CARTESIAN_POINT('Ctrl Pts',(66.2956301826426,200.621620147878,17.8713203435596)) ;
#78217=CARTESIAN_POINT('Ctrl Pts',(67.9219091272743,198.140564861203,17.8713203435596)) ;
#78218=CARTESIAN_POINT('Ctrl Pts',(71.3588126586277,194.203339283954,17.8713203435596)) ;
#78219=CARTESIAN_POINT('Ctrl Pts',(75.3934324114903,190.922060530236,17.8713203435596)) ;
#78220=CARTESIAN_POINT('Ctrl Pts',(77.1942359127805,189.615407485539,17.8713203435596)) ;
#78221=CARTESIAN_POINT('',(65.3716786148033,202.116206289769,17.8713203435596)) ;
#78222=CARTESIAN_POINT('Origin',(94.003679466336,218.783592840001,17.8713203435596)) ;
#78223=CARTESIAN_POINT('Origin',(136.119542118164,279.889814321892,17.8713203435596)) ;
#78224=CARTESIAN_POINT('',(62.3340105195836,212.340553587281,17.8713203435596)) ;
#78225=CARTESIAN_POINT('',(62.589983859128,212.63785590951,17.8713203435596)) ;
#78226=CARTESIAN_POINT('Ctrl Pts',(62.3340105195836,212.340553587281,17.8713203435596)) ;
#78227=CARTESIAN_POINT('Ctrl Pts',(62.3233636275578,212.382972990323,17.8713203435596)) ;
#78228=CARTESIAN_POINT('Ctrl Pts',(62.325696101677,212.462284462768,17.8713203435596)) ;
#78229=CARTESIAN_POINT('Ctrl Pts',(62.385161130142,212.569871661429,17.8713203435596)) ;
#78230=CARTESIAN_POINT('Ctrl Pts',(62.4795535223665,212.632687025067,17.8713203435596)) ;
#78231=CARTESIAN_POINT('Ctrl Pts',(62.5573360365752,212.641025821764,17.8713203435596)) ;
#78232=CARTESIAN_POINT('Ctrl Pts',(62.589983859128,212.63785590951,17.8713203435596)) ;
#78233=CARTESIAN_POINT('',(66.527756290484,202.051005908224,17.8713203435596)) ;
#78234=CARTESIAN_POINT('Ctrl Pts',(66.527756290484,202.051005908224,17.8713203435596)) ;
#78235=CARTESIAN_POINT('Ctrl Pts',(64.5939733104855,205.226459086719,17.8713203435596)) ;
#78236=CARTESIAN_POINT('Ctrl Pts',(63.2390973142897,208.73450203348,17.8713203435596)) ;
#78237=CARTESIAN_POINT('Ctrl Pts',(62.3340105195836,212.340553587281,17.8713203435596)) ;
#78238=CARTESIAN_POINT('',(66.7327381812905,201.93583548982,17.8713203435596)) ;
#78239=CARTESIAN_POINT('Ctrl Pts',(66.7327381812905,201.93583548982,17.8713203435596)) ;
#78240=CARTESIAN_POINT('Ctrl Pts',(66.6859373054892,201.93583548982,17.8713203435596)) ;
#78241=CARTESIAN_POINT('Ctrl Pts',(66.6041999927209,201.960528245756,17.8713203435596)) ;
#78242=CARTESIAN_POINT('Ctrl Pts',(66.5460129584359,202.021026745683,17.8713203435596)) ;
#78243=CARTESIAN_POINT('Ctrl Pts',(66.5277562904841,202.051005908224,17.8713203435596)) ;
#78244=CARTESIAN_POINT('',(72.60844030336,201.93583548982,17.8713203435596)) ;
#78245=CARTESIAN_POINT('',(69.2835637989163,201.93583548982,17.8713203435596)) ;
#78246=CARTESIAN_POINT('',(72.8206412688368,202.287954846983,17.8713203435596)) ;
#78247=CARTESIAN_POINT('Ctrl Pts',(72.8206412688368,202.287954846983,17.8713203435596)) ;
#78248=CARTESIAN_POINT('Ctrl Pts',(72.8426038333632,202.246387739262,17.8713203435596)) ;
#78249=CARTESIAN_POINT('Ctrl Pts',(72.8613131310738,202.149998406772,17.8713203435596)) ;
#78250=CARTESIAN_POINT('Ctrl Pts',(72.8140046703539,202.036931343871,17.8713203435596)) ;
#78251=CARTESIAN_POINT('Ctrl Pts',(72.7257128617816,201.957306367625,17.8713203435596)) ;
#78252=CARTESIAN_POINT('Ctrl Pts',(72.6554528408887,201.93583548982,17.8713203435596)) ;
#78253=CARTESIAN_POINT('Ctrl Pts',(72.60844030336,201.93583548982,17.8713203435596)) ;
#78254=CARTESIAN_POINT('',(69.5945599532053,211.778145438093,17.8713203435596)) ;
#78255=CARTESIAN_POINT('Ctrl Pts',(69.5945599532053,211.778145438093,17.8713203435596)) ;
#78256=CARTESIAN_POINT('Ctrl Pts',(70.1332499807628,208.465417915073,17.8713203435596)) ;
#78257=CARTESIAN_POINT('Ctrl Pts',(71.2527352912136,205.255427820841,17.8713203435596)) ;
#78258=CARTESIAN_POINT('Ctrl Pts',(72.8206412688369,202.287954846983,17.8713203435596)) ;
#78259=CARTESIAN_POINT('',(69.3808650318164,211.978501142072,17.8713203435596)) ;
#78260=CARTESIAN_POINT('Ctrl Pts',(69.3808650318164,211.978501142072,17.8713203435596)) ;
#78261=CARTESIAN_POINT('Ctrl Pts',(69.4256633316016,211.97415148968,17.8713203435596)) ;
#78262=CARTESIAN_POINT('Ctrl Pts',(69.5273477579344,211.933842521524,17.8713203435596)) ;
#78263=CARTESIAN_POINT('Ctrl Pts',(69.5849277942338,211.837379350916,17.8713203435596)) ;
#78264=CARTESIAN_POINT('Ctrl Pts',(69.5945599532053,211.778145438093,17.8713203435596)) ;
#78265=CARTESIAN_POINT('',(64.0594779752363,212.495176642042,17.8713203435596)) ;
#78266=CARTESIAN_POINT('Origin',(67.6417475736039,200.55583548982,23.8713203435596)) ;
#78267=CARTESIAN_POINT('Origin',(74.5963384974435,195.522687624282,19.3713203435596)) ;
#78268=CARTESIAN_POINT('Ctrl Pts',(72.60844030336,202.05583548982,17.9913203435596)) ;
#78269=CARTESIAN_POINT('Ctrl Pts',(72.6319465721243,202.05583548982,17.9913203435596)) ;
#78270=CARTESIAN_POINT('Ctrl Pts',(72.6670765825708,202.066570928722,17.9913203435596)) ;
#78271=CARTESIAN_POINT('Ctrl Pts',(72.7112224868569,202.106383416845,17.9913203435596)) ;
#78272=CARTESIAN_POINT('Ctrl Pts',(72.7348767172168,202.162916948296,17.9913203435596)) ;
#78273=CARTESIAN_POINT('Ctrl Pts',(72.7255220683616,202.211111614541,17.9913203435596)) ;
#78274=CARTESIAN_POINT('Ctrl Pts',(72.7145407860984,202.231895168402,17.9913203435596)) ;
#78275=CARTESIAN_POINT('Ctrl Pts',(72.60844030336,202.05583548982,17.9554164275186)) ;
#78276=CARTESIAN_POINT('Ctrl Pts',(72.6318714497812,202.05583548982,17.9554164275186)) ;
#78277=CARTESIAN_POINT('Ctrl Pts',(72.6669974209846,202.066716144597,17.9554164275186)) ;
#78278=CARTESIAN_POINT('Ctrl Pts',(72.711037641787,202.106460151246,17.9554164275186)) ;
#78279=CARTESIAN_POINT('Ctrl Pts',(72.734701742353,202.162954813346,17.9554164275186)) ;
#78280=CARTESIAN_POINT('Ctrl Pts',(72.7254869739082,202.211178035515,17.9554164275186)) ;
#78281=CARTESIAN_POINT('Ctrl Pts',(72.7145407860984,202.231895168402,17.9554164275186)) ;
#78282=CARTESIAN_POINT('Ctrl Pts',(72.60844030336,202.025677145806,17.8932837596863)) ;
#78283=CARTESIAN_POINT('Ctrl Pts',(72.6378715047901,202.025677145806,17.8932837596863)) ;
#78284=CARTESIAN_POINT('Ctrl Pts',(72.6818313058633,202.039077075185,17.8932837596863)) ;
#78285=CARTESIAN_POINT('Ctrl Pts',(72.7370963439361,202.088911033826,17.8932837596863)) ;
#78286=CARTESIAN_POINT('Ctrl Pts',(72.766693065086,202.159661522209,17.8932837596863)) ;
#78287=CARTESIAN_POINT('Ctrl Pts',(72.7549551073561,202.219961855007,17.8932837596863)) ;
#78288=CARTESIAN_POINT('Ctrl Pts',(72.7412059099191,202.245984060668,17.8932837596863)) ;
#78289=CARTESIAN_POINT('Ctrl Pts',(72.60844030336,201.962763426851,17.8713203435596)) ;
#78290=CARTESIAN_POINT('Ctrl Pts',(72.6501888364698,201.962763426851,17.8713203435596)) ;
#78291=CARTESIAN_POINT('Ctrl Pts',(72.7125662816165,201.981804420182,17.8713203435596)) ;
#78292=CARTESIAN_POINT('Ctrl Pts',(72.7909669519409,202.052505331102,17.8713203435596)) ;
#78293=CARTESIAN_POINT('Ctrl Pts',(72.8329659981049,202.152891882086,17.8713203435596)) ;
#78294=CARTESIAN_POINT('Ctrl Pts',(72.8163357874141,202.238462255222,17.8713203435596)) ;
#78295=CARTESIAN_POINT('Ctrl Pts',(72.7968323761858,202.275375084527,17.8713203435596)) ;
#78296=CARTESIAN_POINT('Ctrl Pts',(72.60844030336,201.93583548982,17.8713203435596)) ;
#78297=CARTESIAN_POINT('Ctrl Pts',(72.6554528408887,201.93583548982,17.8713203435596)) ;
#78298=CARTESIAN_POINT('Ctrl Pts',(72.7257128617816,201.957306367625,17.8713203435596)) ;
#78299=CARTESIAN_POINT('Ctrl Pts',(72.8140046703539,202.036931343871,17.8713203435596)) ;
#78300=CARTESIAN_POINT('Ctrl Pts',(72.8613131310738,202.149998406772,17.8713203435596)) ;
#78301=CARTESIAN_POINT('Ctrl Pts',(72.8426038333632,202.246387739262,17.8713203435596)) ;
#78302=CARTESIAN_POINT('Ctrl Pts',(72.8206412688368,202.287954846983,17.8713203435596)) ;
#78303=CARTESIAN_POINT('',(72.60844030336,202.05583548982,17.9913203435596)) ;
#78304=CARTESIAN_POINT('Origin',(72.60844030336,201.93583548982,17.9913203435596)) ;
#78305=CARTESIAN_POINT('',(72.7145407860984,202.231895168402,17.9913203435596)) ;
#78306=CARTESIAN_POINT('Ctrl Pts',(72.60844030336,202.05583548982,17.9913203435596)) ;
#78307=CARTESIAN_POINT('Ctrl Pts',(72.6319474672212,202.05583548982,17.9913203435596)) ;
#78308=CARTESIAN_POINT('Ctrl Pts',(72.6729579207971,202.068347425336,17.9913203435596)) ;
#78309=CARTESIAN_POINT('Ctrl Pts',(72.7188163051483,202.116230495061,17.9913203435596)) ;
#78310=CARTESIAN_POINT('Ctrl Pts',(72.7339278206143,202.175611043943,17.9913203435596)) ;
#78311=CARTESIAN_POINT('Ctrl Pts',(72.7227770614135,202.216306909442,17.9913203435596)) ;
#78312=CARTESIAN_POINT('Ctrl Pts',(72.7145407860984,202.231895168402,17.9913203435596)) ;
#78313=CARTESIAN_POINT('Origin',(72.8206412688368,202.287954846983,17.9913203435596)) ;
#78314=CARTESIAN_POINT('Origin',(72.60844030336,202.17583548982,19.2513203435596)) ;
#78315=CARTESIAN_POINT('',(72.7145407860985,202.231895168402,19.2513203435596)) ;
#78316=CARTESIAN_POINT('',(72.60844030336,202.17583548982,19.3713203435596)) ;
#78317=CARTESIAN_POINT('Origin',(72.6084403033599,202.17583548982,19.2513203435596)) ;
#78318=CARTESIAN_POINT('',(72.60844030336,202.05583548982,19.2513203435596)) ;
#78319=CARTESIAN_POINT('Origin',(72.60844030336,202.17583548982,19.2513203435596)) ;
#78320=CARTESIAN_POINT('Origin',(72.60844030336,202.17583548982,19.2513203435596)) ;
#78321=CARTESIAN_POINT('Ctrl Pts',(72.60844030336,202.05583548982,19.2513203435596)) ;
#78322=CARTESIAN_POINT('Ctrl Pts',(72.60844030336,202.05583548982,17.7393203435596)) ;
#78323=CARTESIAN_POINT('Ctrl Pts',(72.6319474672212,202.05583548982,19.2513203435596)) ;
#78324=CARTESIAN_POINT('Ctrl Pts',(72.6319474672212,202.05583548982,17.7393203435596)) ;
#78325=CARTESIAN_POINT('Ctrl Pts',(72.6729579207971,202.068347425336,19.2513203435596)) ;
#78326=CARTESIAN_POINT('Ctrl Pts',(72.6729579207971,202.068347425336,17.7393203435596)) ;
#78327=CARTESIAN_POINT('Ctrl Pts',(72.7188163051483,202.116230495061,19.2513203435596)) ;
#78328=CARTESIAN_POINT('Ctrl Pts',(72.7188163051483,202.116230495061,17.7393203435596)) ;
#78329=CARTESIAN_POINT('Ctrl Pts',(72.7339278206143,202.175611043943,19.2513203435596)) ;
#78330=CARTESIAN_POINT('Ctrl Pts',(72.7339278206143,202.175611043943,17.7393203435596)) ;
#78331=CARTESIAN_POINT('Ctrl Pts',(72.7227770614135,202.216306909442,19.2513203435596)) ;
#78332=CARTESIAN_POINT('Ctrl Pts',(72.7227770614135,202.216306909442,17.7393203435596)) ;
#78333=CARTESIAN_POINT('Ctrl Pts',(72.7145407860984,202.231895168402,19.2513203435596)) ;
#78334=CARTESIAN_POINT('Ctrl Pts',(72.7145407860984,202.231895168402,17.7393203435596)) ;
#78335=CARTESIAN_POINT('',(72.60844030336,202.05583548982,17.9913203435596)) ;
#78336=CARTESIAN_POINT('',(72.7145407860984,202.231895168402,19.2513203435596)) ;
#78337=CARTESIAN_POINT('Ctrl Pts',(66.6302472358873,202.113420699022,17.9913203435596)) ;
#78338=CARTESIAN_POINT('Ctrl Pts',(66.6393755698632,202.098431117751,17.9913203435596)) ;
#78339=CARTESIAN_POINT('Ctrl Pts',(66.6684690870057,202.068181867788,17.9913203435596)) ;
#78340=CARTESIAN_POINT('Ctrl Pts',(66.7093377433898,202.05583548982,17.9913203435596)) ;
#78341=CARTESIAN_POINT('Ctrl Pts',(66.7327381812905,202.05583548982,17.9913203435596)) ;
#78342=CARTESIAN_POINT('Ctrl Pts',(66.6302472358873,202.113420699022,17.9554164275186)) ;
#78343=CARTESIAN_POINT('Ctrl Pts',(66.6393463971415,202.098479022099,17.9554164275186)) ;
#78344=CARTESIAN_POINT('Ctrl Pts',(66.6684615598882,202.068262037652,17.9554164275186)) ;
#78345=CARTESIAN_POINT('Ctrl Pts',(66.7094125275141,202.05583548982,17.9554164275186)) ;
#78346=CARTESIAN_POINT('Ctrl Pts',(66.7327381812905,202.05583548982,17.9554164275186)) ;
#78347=CARTESIAN_POINT('Ctrl Pts',(66.6044893329729,202.09773468778,17.8932836561957)) ;
#78348=CARTESIAN_POINT('Ctrl Pts',(66.6159185325052,202.078966869282,17.8932836561957)) ;
#78349=CARTESIAN_POINT('Ctrl Pts',(66.652318794356,202.04110795527,17.8932836561957)) ;
#78350=CARTESIAN_POINT('Ctrl Pts',(66.703439486193,202.025677232058,17.8932836561957)) ;
#78351=CARTESIAN_POINT('Ctrl Pts',(66.7327381812905,202.025677232058,17.8932836561957)) ;
#78352=CARTESIAN_POINT('Ctrl Pts',(66.5507552048511,202.065011754527,17.8713203435596)) ;
#78353=CARTESIAN_POINT('Ctrl Pts',(66.5669676695792,202.03838936557,17.8713203435596)) ;
#78354=CARTESIAN_POINT('Ctrl Pts',(66.618623024887,201.984674147107,17.8713203435596)) ;
#78355=CARTESIAN_POINT('Ctrl Pts',(66.6911776100968,201.962763426851,17.8713203435596)) ;
#78356=CARTESIAN_POINT('Ctrl Pts',(66.7327381812905,201.962763426851,17.8713203435596)) ;
#78357=CARTESIAN_POINT('Ctrl Pts',(66.5277562904841,202.051005908224,17.8713203435596)) ;
#78358=CARTESIAN_POINT('Ctrl Pts',(66.5460129584359,202.021026745683,17.8713203435596)) ;
#78359=CARTESIAN_POINT('Ctrl Pts',(66.6041999927209,201.960528245756,17.8713203435596)) ;
#78360=CARTESIAN_POINT('Ctrl Pts',(66.6859373054892,201.93583548982,17.8713203435596)) ;
#78361=CARTESIAN_POINT('Ctrl Pts',(66.7327381812905,201.93583548982,17.8713203435596)) ;
#78362=CARTESIAN_POINT('',(66.6302472358873,202.113420699022,17.9913203435596)) ;
#78363=CARTESIAN_POINT('Origin',(66.527756290484,202.051005908224,17.9913203435596)) ;
#78364=CARTESIAN_POINT('',(66.7327381812905,202.05583548982,17.9913203435596)) ;
#78365=CARTESIAN_POINT('Origin',(66.7381174716576,202.184021451547,17.9913203435596)) ;
#78366=CARTESIAN_POINT('Origin',(66.7327381812905,201.93583548982,17.9913203435596)) ;
#78367=CARTESIAN_POINT('Ctrl Pts',(69.4761157303972,211.75888495826,17.9913203435596)) ;
#78368=CARTESIAN_POINT('Ctrl Pts',(69.4712996509114,211.788501914672,17.9913203435596)) ;
#78369=CARTESIAN_POINT('Ctrl Pts',(69.4425096327617,211.836733499976,17.9913203435596)) ;
#78370=CARTESIAN_POINT('Ctrl Pts',(69.3916674195954,211.856887984054,17.9913203435596)) ;
#78371=CARTESIAN_POINT('Ctrl Pts',(69.3692682697028,211.85906281025,17.9913203435596)) ;
#78372=CARTESIAN_POINT('Ctrl Pts',(69.4761157303972,211.75888495826,17.9554164275186)) ;
#78373=CARTESIAN_POINT('Ctrl Pts',(69.4713150423451,211.788407263531,17.9554164275186)) ;
#78374=CARTESIAN_POINT('Ctrl Pts',(69.4423950698463,211.836692828306,17.9554164275186)) ;
#78375=CARTESIAN_POINT('Ctrl Pts',(69.3915958354303,211.856894934457,17.9554164275186)) ;
#78376=CARTESIAN_POINT('Ctrl Pts',(69.3692682697028,211.85906281025,17.9554164275186)) ;
#78377=CARTESIAN_POINT('Ctrl Pts',(69.5058831605967,211.763725506625,17.8932838610488)) ;
#78378=CARTESIAN_POINT('Ctrl Pts',(69.4998531518842,211.800807640699,17.8932838610488)) ;
#78379=CARTESIAN_POINT('Ctrl Pts',(69.4638576015521,211.861148345767,17.8932838610488)) ;
#78380=CARTESIAN_POINT('Ctrl Pts',(69.4002277955916,211.88635707259,17.8932838610488)) ;
#78381=CARTESIAN_POINT('Ctrl Pts',(69.3721827707107,211.889080080163,17.8932838610488)) ;
#78382=CARTESIAN_POINT('Ctrl Pts',(69.56798113176,211.773823396525,17.8713203435596)) ;
#78383=CARTESIAN_POINT('Ctrl Pts',(69.5594274877986,211.826424874784,17.8713203435596)) ;
#78384=CARTESIAN_POINT('Ctrl Pts',(69.5083265820412,211.912057149791,17.8713203435596)) ;
#78385=CARTESIAN_POINT('Ctrl Pts',(69.4180449485487,211.947836622252,17.8713203435596)) ;
#78386=CARTESIAN_POINT('Ctrl Pts',(69.3782627244835,211.951699243085,17.8713203435596)) ;
#78387=CARTESIAN_POINT('Ctrl Pts',(69.5945599532053,211.778145438093,17.8713203435596)) ;
#78388=CARTESIAN_POINT('Ctrl Pts',(69.5849277942338,211.837379350916,17.8713203435596)) ;
#78389=CARTESIAN_POINT('Ctrl Pts',(69.5273477579344,211.933842521524,17.8713203435596)) ;
#78390=CARTESIAN_POINT('Ctrl Pts',(69.4256633316016,211.97415148968,17.8713203435596)) ;
#78391=CARTESIAN_POINT('Ctrl Pts',(69.3808650318164,211.978501142072,17.8713203435596)) ;
#78392=CARTESIAN_POINT('',(69.4761157303972,211.75888495826,17.9913203435596)) ;
#78393=CARTESIAN_POINT('Origin',(69.5945599532053,211.778145438093,17.9913203435596)) ;
#78394=CARTESIAN_POINT('',(69.3692682697028,211.85906281025,17.9913203435596)) ;
#78395=CARTESIAN_POINT('Ctrl Pts',(69.4761157303972,211.75888495826,17.9913203435596)) ;
#78396=CARTESIAN_POINT('Ctrl Pts',(69.4725035530572,211.781098399535,17.9913203435596)) ;
#78397=CARTESIAN_POINT('Ctrl Pts',(69.4491186156896,211.830541090259,17.9913203435596)) ;
#78398=CARTESIAN_POINT('Ctrl Pts',(69.3991347762822,211.856162947478,17.9913203435596)) ;
#78399=CARTESIAN_POINT('Ctrl Pts',(69.3692682697028,211.85906281025,17.9913203435596)) ;
#78400=CARTESIAN_POINT('Origin',(69.3808650318164,211.978501142072,17.9913203435596)) ;
#78401=CARTESIAN_POINT('Origin',(66.7327381812904,202.17583548982,19.2513203435596)) ;
#78402=CARTESIAN_POINT('',(66.7327381812904,202.05583548982,19.2513203435596)) ;
#78403=CARTESIAN_POINT('',(66.7327381812905,202.17583548982,19.3713203435596)) ;
#78404=CARTESIAN_POINT('Origin',(66.7327381812904,202.17583548982,19.2513203435596)) ;
#78405=CARTESIAN_POINT('',(66.6302472358883,202.11342069902,19.2513203435596)) ;
#78406=CARTESIAN_POINT('Origin',(66.7327381812904,202.17583548982,19.2513203435596)) ;
#78407=CARTESIAN_POINT('Origin',(66.7327381812905,202.17583548982,19.2513203435596)) ;
#78408=CARTESIAN_POINT('Ctrl Pts',(66.6302472358873,202.113420699022,19.2513203435596)) ;
#78409=CARTESIAN_POINT('Ctrl Pts',(66.6302472358873,202.113420699022,17.7393203435596)) ;
#78410=CARTESIAN_POINT('Ctrl Pts',(66.6515473457387,202.078443919192,19.2513203435596)) ;
#78411=CARTESIAN_POINT('Ctrl Pts',(66.6515473457387,202.078443919192,17.7393203435596)) ;
#78412=CARTESIAN_POINT('Ctrl Pts',(66.6917861385215,202.05583548982,19.2513203435596)) ;
#78413=CARTESIAN_POINT('Ctrl Pts',(66.6917861385215,202.05583548982,17.7393203435596)) ;
#78414=CARTESIAN_POINT('Ctrl Pts',(66.7327381812904,202.05583548982,19.2513203435596)) ;
#78415=CARTESIAN_POINT('Ctrl Pts',(66.7327381812904,202.05583548982,17.7393203435596)) ;
#78416=CARTESIAN_POINT('',(66.6302472358873,202.113420699022,17.9913203435596)) ;
#78417=CARTESIAN_POINT('',(66.7327381812904,202.05583548982,19.2513203435596)) ;
#78418=CARTESIAN_POINT('Origin',(69.3576715158512,211.739624427619,19.2513203435596)) ;
#78419=CARTESIAN_POINT('',(69.4761157303957,211.758884958269,19.2513203435596)) ;
#78420=CARTESIAN_POINT('',(69.3692682697028,211.85906281025,19.2513203435596)) ;
#78421=CARTESIAN_POINT('Origin',(69.3576715075891,211.739624478427,19.2513203435596)) ;
#78422=CARTESIAN_POINT('',(69.3576715245022,211.739624453345,19.3713203435596)) ;
#78423=CARTESIAN_POINT('Origin',(69.3576715158512,211.739624427619,19.2513203435596)) ;
#78424=CARTESIAN_POINT('Origin',(69.3576715075891,211.739624478427,19.2513203435596)) ;
#78425=CARTESIAN_POINT('Ctrl Pts',(72.7145407860984,202.231895168402,19.2513203435596)) ;
#78426=CARTESIAN_POINT('Ctrl Pts',(71.1398059575599,205.212292661218,19.2513203435596)) ;
#78427=CARTESIAN_POINT('Ctrl Pts',(70.0168498128443,208.433587317836,19.2513203435596)) ;
#78428=CARTESIAN_POINT('Ctrl Pts',(69.4761157303972,211.75888495826,19.2513203435596)) ;
#78429=CARTESIAN_POINT('Ctrl Pts',(72.7145407860984,202.231895168402,19.2872242596007)) ;
#78430=CARTESIAN_POINT('Ctrl Pts',(71.1398228541547,205.212260682139,19.2872242596007)) ;
#78431=CARTESIAN_POINT('Ctrl Pts',(70.016843012287,208.433629138534,19.2872242596007)) ;
#78432=CARTESIAN_POINT('Ctrl Pts',(69.4761157303972,211.75888495826,19.2872242596007)) ;
#78433=CARTESIAN_POINT('Ctrl Pts',(72.6878755734951,202.217806229225,19.349356806951)) ;
#78434=CARTESIAN_POINT('Ctrl Pts',(71.1118081030027,205.200725926204,19.349356806951)) ;
#78435=CARTESIAN_POINT('Ctrl Pts',(69.9876187299006,208.425448349774,19.349356806951)) ;
#78436=CARTESIAN_POINT('Ctrl Pts',(69.4463482844696,211.754044407338,19.349356806951)) ;
#78437=CARTESIAN_POINT('Ctrl Pts',(72.632249196011,202.188415252277,19.3713203435596)) ;
#78438=CARTESIAN_POINT('Ctrl Pts',(71.0534112985986,205.176578354872,19.3713203435596)) ;
#78439=CARTESIAN_POINT('Ctrl Pts',(69.9266358184916,208.408493389076,19.3713203435596)) ;
#78440=CARTESIAN_POINT('Ctrl Pts',(69.3842503290344,211.743946519995,19.3713203435596)) ;
#78441=CARTESIAN_POINT('Ctrl Pts',(72.60844030336,202.17583548982,19.3713203435596)) ;
#78442=CARTESIAN_POINT('Ctrl Pts',(71.0284184206553,205.166239443848,19.3713203435596)) ;
#78443=CARTESIAN_POINT('Ctrl Pts',(69.9005335285577,208.401240869919,19.3713203435596)) ;
#78444=CARTESIAN_POINT('Ctrl Pts',(69.3576715075891,211.739624478427,19.3713203435596)) ;
#78445=CARTESIAN_POINT('Ctrl Pts',(69.4761157303972,211.75888495826,19.2513203435596)) ;
#78446=CARTESIAN_POINT('Ctrl Pts',(70.0168498128443,208.433587317836,19.2513203435596)) ;
#78447=CARTESIAN_POINT('Ctrl Pts',(71.1398059575599,205.212292661218,19.2513203435596)) ;
#78448=CARTESIAN_POINT('Ctrl Pts',(72.7145407860984,202.231895168402,19.2513203435596)) ;
#78449=CARTESIAN_POINT('Ctrl Pts',(72.60844030336,202.17583548982,19.3713203435596)) ;
#78450=CARTESIAN_POINT('Ctrl Pts',(71.0284184249332,205.166239435752,19.3713203435596)) ;
#78451=CARTESIAN_POINT('Ctrl Pts',(69.9005335346653,208.401240852402,19.3713203435596)) ;
#78452=CARTESIAN_POINT('Ctrl Pts',(69.3576715119986,211.739624451311,19.3713203435596)) ;
#78453=CARTESIAN_POINT('Ctrl Pts',(62.5783870970144,212.518417577687,17.9913203435596)) ;
#78454=CARTESIAN_POINT('Ctrl Pts',(62.562063185738,212.520002533814,17.9913203435596)) ;
#78455=CARTESIAN_POINT('Ctrl Pts',(62.5231719286336,212.515833135466,17.9913203435596)) ;
#78456=CARTESIAN_POINT('Ctrl Pts',(62.4759757325213,212.484425453647,17.9913203435596)) ;
#78457=CARTESIAN_POINT('Ctrl Pts',(62.4462432182888,212.430631854317,17.9913203435596)) ;
#78458=CARTESIAN_POINT('Ctrl Pts',(62.4450769812292,212.390976118094,17.9913203435596)) ;
#78459=CARTESIAN_POINT('Ctrl Pts',(62.4504004272421,212.369766416573,17.9913203435596)) ;
#78460=CARTESIAN_POINT('Ctrl Pts',(62.5783870970144,212.518417577687,17.9554164275186)) ;
#78461=CARTESIAN_POINT('Ctrl Pts',(62.5621153543946,212.519997468544,17.9554164275186)) ;
#78462=CARTESIAN_POINT('Ctrl Pts',(62.5232486540694,212.515725612279,17.9554164275186)) ;
#78463=CARTESIAN_POINT('Ctrl Pts',(62.4760976399362,212.484295588733,17.9554164275186)) ;
#78464=CARTESIAN_POINT('Ctrl Pts',(62.4464066667739,212.430611808364,17.9554164275186)) ;
#78465=CARTESIAN_POINT('Ctrl Pts',(62.4450939941266,212.390908335219,17.9554164275186)) ;
#78466=CARTESIAN_POINT('Ctrl Pts',(62.4504004272421,212.369766416573,17.9554164275186)) ;
#78467=CARTESIAN_POINT('Ctrl Pts',(62.5813015900153,212.548434765134,17.8932837616354)) ;
#78468=CARTESIAN_POINT('Ctrl Pts',(62.560863113551,212.55041922143,17.8932837616354)) ;
#78469=CARTESIAN_POINT('Ctrl Pts',(62.5121920524828,212.545225632173,17.8932837616354)) ;
#78470=CARTESIAN_POINT('Ctrl Pts',(62.4531240959624,212.505929745317,17.8932837616354)) ;
#78471=CARTESIAN_POINT('Ctrl Pts',(62.4159096267281,212.438591402704,17.8932837616354)) ;
#78472=CARTESIAN_POINT('Ctrl Pts',(62.4144841075688,212.388980428609,17.8932837616354)) ;
#78473=CARTESIAN_POINT('Ctrl Pts',(62.4211493683755,212.362424661549,17.8932837616354)) ;
#78474=CARTESIAN_POINT('Ctrl Pts',(62.5873815517951,212.611054010523,17.8713203435596)) ;
#78475=CARTESIAN_POINT('Ctrl Pts',(62.5583893132889,212.613868986988,17.8713203435596)) ;
#78476=CARTESIAN_POINT('Ctrl Pts',(62.4893304496322,212.606480517307,17.8713203435596)) ;
#78477=CARTESIAN_POINT('Ctrl Pts',(62.4055223694806,212.550716229971,17.8713203435596)) ;
#78478=CARTESIAN_POINT('Ctrl Pts',(62.3527233349889,212.455184513277,17.8713203435596)) ;
#78479=CARTESIAN_POINT('Ctrl Pts',(62.3506735966604,212.384778623772,17.8713203435596)) ;
#78480=CARTESIAN_POINT('Ctrl Pts',(62.3601283537873,212.347108930845,17.8713203435596)) ;
#78481=CARTESIAN_POINT('Ctrl Pts',(62.589983859128,212.63785590951,17.8713203435596)) ;
#78482=CARTESIAN_POINT('Ctrl Pts',(62.5573360365752,212.641025821764,17.8713203435596)) ;
#78483=CARTESIAN_POINT('Ctrl Pts',(62.4795535223665,212.632687025067,17.8713203435596)) ;
#78484=CARTESIAN_POINT('Ctrl Pts',(62.385161130142,212.569871661429,17.8713203435596)) ;
#78485=CARTESIAN_POINT('Ctrl Pts',(62.325696101677,212.462284462768,17.8713203435596)) ;
#78486=CARTESIAN_POINT('Ctrl Pts',(62.3233636275578,212.382972990323,17.8713203435596)) ;
#78487=CARTESIAN_POINT('Ctrl Pts',(62.3340105195836,212.340553587281,17.8713203435596)) ;
#78488=CARTESIAN_POINT('',(62.5783870970144,212.518417577687,17.9913203435596)) ;
#78489=CARTESIAN_POINT('Origin',(62.589983859128,212.63785590951,17.9913203435596)) ;
#78490=CARTESIAN_POINT('',(62.4504004272421,212.369766416573,17.9913203435596)) ;
#78491=CARTESIAN_POINT('Ctrl Pts',(62.5783870970144,212.518417577687,17.9913203435596)) ;
#78492=CARTESIAN_POINT('Ctrl Pts',(62.562063185738,212.520002533814,17.9913203435596)) ;
#78493=CARTESIAN_POINT('Ctrl Pts',(62.5231719286336,212.515833135466,17.9913203435596)) ;
#78494=CARTESIAN_POINT('Ctrl Pts',(62.4759757325213,212.484425453647,17.9913203435596)) ;
#78495=CARTESIAN_POINT('Ctrl Pts',(62.4462432182888,212.430631854317,17.9913203435596)) ;
#78496=CARTESIAN_POINT('Ctrl Pts',(62.4450769812292,212.390976118094,17.9913203435596)) ;
#78497=CARTESIAN_POINT('Ctrl Pts',(62.4504004272421,212.369766416573,17.9913203435596)) ;
#78498=CARTESIAN_POINT('Origin',(62.3340105195836,212.340553587281,17.9913203435596)) ;
#78499=CARTESIAN_POINT('Origin',(62.5667903349007,212.398979245865,19.2513203435596)) ;
#78500=CARTESIAN_POINT('',(62.450400427238,212.36976641659,19.2513203435596)) ;
#78501=CARTESIAN_POINT('',(62.5667903349007,212.398979245865,19.3713203435596)) ;
#78502=CARTESIAN_POINT('Origin',(62.5667903349007,212.398979245865,19.2513203435596)) ;
#78503=CARTESIAN_POINT('',(62.4617165382906,212.456940416194,19.2513203435596)) ;
#78504=CARTESIAN_POINT('Origin',(62.5667903349007,212.398979245865,19.2513203435596)) ;
#78505=CARTESIAN_POINT('',(62.5783870970144,212.518417577687,19.2513203435596)) ;
#78506=CARTESIAN_POINT('Origin',(62.5667903349007,212.398979245865,19.2513203435596)) ;
#78507=CARTESIAN_POINT('Origin',(62.5667903349007,212.398979245865,19.2513203435596)) ;
#78508=CARTESIAN_POINT('Ctrl Pts',(62.5783870970144,212.518417577687,19.2513203435596)) ;
#78509=CARTESIAN_POINT('Ctrl Pts',(62.5783870970144,212.518417577687,17.7393203435596)) ;
#78510=CARTESIAN_POINT('Ctrl Pts',(62.5566209022384,212.520530947651,19.2513203435596)) ;
#78511=CARTESIAN_POINT('Ctrl Pts',(62.5566209022384,212.520530947651,17.7393203435596)) ;
#78512=CARTESIAN_POINT('Ctrl Pts',(62.5175562241547,212.513505863603,19.2513203435596)) ;
#78513=CARTESIAN_POINT('Ctrl Pts',(62.5175562241547,212.513505863603,17.7393203435596)) ;
#78514=CARTESIAN_POINT('Ctrl Pts',(62.473284759297,212.47948630102,19.2513203435596)) ;
#78515=CARTESIAN_POINT('Ctrl Pts',(62.473284759297,212.47948630102,17.7393203435596)) ;
#78516=CARTESIAN_POINT('Ctrl Pts',(62.446220083906,212.43065192189,19.2513203435596)) ;
#78517=CARTESIAN_POINT('Ctrl Pts',(62.446220083906,212.43065192189,17.7393203435596)) ;
#78518=CARTESIAN_POINT('Ctrl Pts',(62.4450767415993,212.390977072829,19.2513203435596)) ;
#78519=CARTESIAN_POINT('Ctrl Pts',(62.4450767415993,212.390977072829,17.7393203435596)) ;
#78520=CARTESIAN_POINT('Ctrl Pts',(62.4504004272421,212.369766416573,19.2513203435596)) ;
#78521=CARTESIAN_POINT('Ctrl Pts',(62.4504004272421,212.369766416573,17.7393203435596)) ;
#78522=CARTESIAN_POINT('',(62.5783870970144,212.518417577687,17.9913203435596)) ;
#78523=CARTESIAN_POINT('',(62.4504004272421,212.369766416573,19.2513203435596)) ;
#78524=CARTESIAN_POINT('Origin',(65.2251874189933,212.140864467154,19.2513203435596)) ;
#78525=CARTESIAN_POINT('',(65.236784181107,212.260302798977,19.2513203435596)) ;
#78526=CARTESIAN_POINT('',(65.2251874189933,212.140864467154,19.3713203435596)) ;
#78527=CARTESIAN_POINT('Ctrl Pts',(62.4504004272421,212.369766416573,19.2513203435596)) ;
#78528=CARTESIAN_POINT('Ctrl Pts',(63.3519937332128,208.777633638912,19.2513203435596)) ;
#78529=CARTESIAN_POINT('Ctrl Pts',(64.7017677689033,205.280165011303,19.2513203435596)) ;
#78530=CARTESIAN_POINT('Ctrl Pts',(66.6302472358874,202.113420699022,19.2513203435596)) ;
#78531=CARTESIAN_POINT('Ctrl Pts',(62.4504004272421,212.369766416573,19.2872242596007)) ;
#78532=CARTESIAN_POINT('Ctrl Pts',(63.3520013377904,208.777603340714,19.2872242596007)) ;
#78533=CARTESIAN_POINT('Ctrl Pts',(64.701744667191,205.280202946483,19.2872242596007)) ;
#78534=CARTESIAN_POINT('Ctrl Pts',(66.6302472358874,202.113420699022,19.2872242596007)) ;
#78535=CARTESIAN_POINT('Ctrl Pts',(62.4796515023926,212.377108175684,19.3493569053396)) ;
#78536=CARTESIAN_POINT('Ctrl Pts',(63.3806450319406,208.787365030391,19.3493569053396)) ;
#78537=CARTESIAN_POINT('Ctrl Pts',(64.7293478035486,205.29285911243,19.3493569053396)) ;
#78538=CARTESIAN_POINT('Ctrl Pts',(66.6560052281957,202.129106764703,19.3493569053396)) ;
#78539=CARTESIAN_POINT('Ctrl Pts',(62.540672500697,212.392423902301,19.3713203435596)) ;
#78540=CARTESIAN_POINT('Ctrl Pts',(63.4404191561371,208.807648559368,19.3713203435596)) ;
#78541=CARTESIAN_POINT('Ctrl Pts',(64.7868696827578,205.319362001607,19.3713203435596)) ;
#78542=CARTESIAN_POINT('Ctrl Pts',(66.7097392669236,202.161829643516,19.3713203435596)) ;
#78543=CARTESIAN_POINT('Ctrl Pts',(62.5667903349007,212.398979245865,19.3713203435596)) ;
#78544=CARTESIAN_POINT('Ctrl Pts',(63.4660041191814,208.816326970999,19.3713203435596)) ;
#78545=CARTESIAN_POINT('Ctrl Pts',(64.8114873900217,205.330709638017,19.3713203435596)) ;
#78546=CARTESIAN_POINT('Ctrl Pts',(66.7327381812906,202.17583548982,19.3713203435596)) ;
#78547=CARTESIAN_POINT('Ctrl Pts',(66.6302472358874,202.113420699022,19.2513203435596)) ;
#78548=CARTESIAN_POINT('Ctrl Pts',(64.7017677689033,205.280165011303,19.2513203435596)) ;
#78549=CARTESIAN_POINT('Ctrl Pts',(63.3519937332128,208.777633638912,19.2513203435596)) ;
#78550=CARTESIAN_POINT('Ctrl Pts',(62.4504004272421,212.369766416573,19.2513203435596)) ;
#78551=CARTESIAN_POINT('Origin',(125.251450136782,268.303013522014,19.3713203435596)) ;
#78552=CARTESIAN_POINT('Ctrl Pts',(62.4504004272422,212.369766416573,17.9913203435596)) ;
#78553=CARTESIAN_POINT('Ctrl Pts',(63.3531047679701,208.773207048405,17.9913203435596)) ;
#78554=CARTESIAN_POINT('Ctrl Pts',(64.703685742309,205.277015518929,17.9913203435596)) ;
#78555=CARTESIAN_POINT('Ctrl Pts',(66.6302472358872,202.113420699022,17.9913203435596)) ;
#78556=CARTESIAN_POINT('Ctrl Pts',(62.4504004272422,212.369766416573,17.9554164275186)) ;
#78557=CARTESIAN_POINT('Ctrl Pts',(63.3530971540214,208.77323738394,17.9554164275186)) ;
#78558=CARTESIAN_POINT('Ctrl Pts',(64.7037088210454,205.276977621478,17.9554164275186)) ;
#78559=CARTESIAN_POINT('Ctrl Pts',(66.6302472358872,202.113420699022,17.9554164275186)) ;
#78560=CARTESIAN_POINT('Ctrl Pts',(62.4211493721785,212.362424662504,17.8932837569307)) ;
#78561=CARTESIAN_POINT('Ctrl Pts',(63.3244542284346,208.76347271722,17.8932837569307)) ;
#78562=CARTESIAN_POINT('Ctrl Pts',(64.6761075374679,205.264318452909,17.8932837569307)) ;
#78563=CARTESIAN_POINT('Ctrl Pts',(66.6044892612671,202.097734644113,17.8932837569307)) ;
#78564=CARTESIAN_POINT('Ctrl Pts',(62.3601283537873,212.347108930845,17.8713203435596)) ;
#78565=CARTESIAN_POINT('Ctrl Pts',(63.264681620676,208.743183061372,17.8713203435596)) ;
#78566=CARTESIAN_POINT('Ctrl Pts',(64.6185894077755,205.237809366857,17.8713203435596)) ;
#78567=CARTESIAN_POINT('Ctrl Pts',(66.550755204851,202.065011754527,17.8713203435596)) ;
#78568=CARTESIAN_POINT('Ctrl Pts',(62.3340105195836,212.340553587281,17.8713203435596)) ;
#78569=CARTESIAN_POINT('Ctrl Pts',(63.2390973142897,208.73450203348,17.8713203435596)) ;
#78570=CARTESIAN_POINT('Ctrl Pts',(64.5939733104855,205.226459086719,17.8713203435596)) ;
#78571=CARTESIAN_POINT('Ctrl Pts',(66.527756290484,202.051005908224,17.8713203435596)) ;
#78572=CARTESIAN_POINT('Origin',(124.881953702128,267.85635873889,17.9913203435596)) ;
#78573=CARTESIAN_POINT('Origin',(64.0594779752363,212.495176642042,17.9913203435596)) ;
#78574=CARTESIAN_POINT('',(64.0478812131227,212.37573831022,17.9913203435596)) ;
#78575=CARTESIAN_POINT('Ctrl Pts',(69.3692682697028,211.85906281025,17.9913203435596)) ;
#78576=CARTESIAN_POINT('Ctrl Pts',(69.3692682697028,211.85906281025,19.5033203435596)) ;
#78577=CARTESIAN_POINT('Ctrl Pts',(69.3991347762822,211.856162947478,17.9913203435596)) ;
#78578=CARTESIAN_POINT('Ctrl Pts',(69.3991347762822,211.856162947478,19.5033203435596)) ;
#78579=CARTESIAN_POINT('Ctrl Pts',(69.4491186156896,211.830541090259,17.9913203435596)) ;
#78580=CARTESIAN_POINT('Ctrl Pts',(69.4491186156896,211.830541090259,19.5033203435596)) ;
#78581=CARTESIAN_POINT('Ctrl Pts',(69.4725035530572,211.781098399535,17.9913203435596)) ;
#78582=CARTESIAN_POINT('Ctrl Pts',(69.4725035530572,211.781098399535,19.5033203435596)) ;
#78583=CARTESIAN_POINT('Ctrl Pts',(69.4761157303972,211.75888495826,17.9913203435596)) ;
#78584=CARTESIAN_POINT('Ctrl Pts',(69.4761157303972,211.75888495826,19.5033203435596)) ;
#78585=CARTESIAN_POINT('',(69.3692682697028,211.85906281025,19.2513203435596)) ;
#78586=CARTESIAN_POINT('',(69.4761157303972,211.75888495826,17.9913203435596)) ;
#78587=CARTESIAN_POINT('Origin',(70.2085194795435,202.17583548982,19.2513203435596)) ;
#78588=CARTESIAN_POINT('',(70.2085194795435,202.05583548982,19.2513203435596)) ;
#78589=CARTESIAN_POINT('',(70.2085194795435,202.17583548982,19.3713203435596)) ;
#78590=CARTESIAN_POINT('Ctrl Pts',(72.7145407860985,202.231895168401,17.9913203435596)) ;
#78591=CARTESIAN_POINT('Ctrl Pts',(71.1413529482141,205.209364773308,17.9913203435596)) ;
#78592=CARTESIAN_POINT('Ctrl Pts',(70.0169340278858,208.433069429121,17.9913203435596)) ;
#78593=CARTESIAN_POINT('Ctrl Pts',(69.4761157303972,211.75888495826,17.9913203435596)) ;
#78594=CARTESIAN_POINT('Ctrl Pts',(72.7145407860985,202.231895168401,17.9554164275186)) ;
#78595=CARTESIAN_POINT('Ctrl Pts',(71.1413360682183,205.209396720971,17.9554164275186)) ;
#78596=CARTESIAN_POINT('Ctrl Pts',(70.0169408295022,208.433027601909,17.9554164275186)) ;
#78597=CARTESIAN_POINT('Ctrl Pts',(69.4761157303972,211.75888495826,17.9554164275186)) ;
#78598=CARTESIAN_POINT('Ctrl Pts',(72.7412059838746,202.245984099743,17.8932838600471)) ;
#78599=CARTESIAN_POINT('Ctrl Pts',(71.1693494787811,205.220933978255,17.8932838600471)) ;
#78600=CARTESIAN_POINT('Ctrl Pts',(70.046165010743,208.441208908193,17.8932838600471)) ;
#78601=CARTESIAN_POINT('Ctrl Pts',(69.5058831597727,211.763725506491,17.8932838600471)) ;
#78602=CARTESIAN_POINT('Ctrl Pts',(72.7968323761859,202.275375084526,17.8713203435596)) ;
#78603=CARTESIAN_POINT('Ctrl Pts',(71.2277435763958,205.245086708446,17.8713203435596)) ;
#78604=CARTESIAN_POINT('Ctrl Pts',(70.1071477650449,208.458164939517,17.8713203435596)) ;
#78605=CARTESIAN_POINT('Ctrl Pts',(69.56798113176,211.773823396525,17.8713203435596)) ;
#78606=CARTESIAN_POINT('Ctrl Pts',(72.8206412688369,202.287954846983,17.8713203435596)) ;
#78607=CARTESIAN_POINT('Ctrl Pts',(71.2527352912136,205.255427820841,17.8713203435596)) ;
#78608=CARTESIAN_POINT('Ctrl Pts',(70.1332499807628,208.465417915073,17.8713203435596)) ;
#78609=CARTESIAN_POINT('Ctrl Pts',(69.5945599532053,211.778145438093,17.8713203435596)) ;
#78610=CARTESIAN_POINT('Ctrl Pts',(72.7145407860985,202.231895168401,17.9913203435596)) ;
#78611=CARTESIAN_POINT('Ctrl Pts',(71.1413529482141,205.209364773308,17.9913203435596)) ;
#78612=CARTESIAN_POINT('Ctrl Pts',(70.0169340278858,208.433069429121,17.9913203435596)) ;
#78613=CARTESIAN_POINT('Ctrl Pts',(69.4761157303972,211.75888495826,17.9913203435596)) ;
#78614=CARTESIAN_POINT('Origin',(69.2835637989163,201.93583548982,17.9913203435596)) ;
#78615=CARTESIAN_POINT('',(69.2835637989163,202.05583548982,17.9913203435596)) ;
#78616=CARTESIAN_POINT('Ctrl Pts',(69.4614223697787,211.850115187154,17.854339447693)) ;
#78617=CARTESIAN_POINT('Ctrl Pts',(69.4614223697787,211.850115187154,32.8747165227329)) ;
#78618=CARTESIAN_POINT('Ctrl Pts',(69.905975823669,209.06303762573,17.854339447693)) ;
#78619=CARTESIAN_POINT('Ctrl Pts',(69.905975823669,209.06303762573,32.8747165227329)) ;
#78620=CARTESIAN_POINT('Ctrl Pts',(70.7494560159525,206.30693385077,17.854339447693)) ;
#78621=CARTESIAN_POINT('Ctrl Pts',(70.7494560159525,206.30693385077,32.8747165227329)) ;
#78622=CARTESIAN_POINT('Ctrl Pts',(72.0309081730459,203.597341394065,17.854339447693)) ;
#78623=CARTESIAN_POINT('Ctrl Pts',(72.0309081730459,203.597341394065,32.8747165227329)) ;
#78624=CARTESIAN_POINT('Ctrl Pts',(72.2749463865981,203.081329852839,17.854339447693)) ;
#78625=CARTESIAN_POINT('Ctrl Pts',(72.2749463865981,203.081329852839,32.8747165227329)) ;
#78626=CARTESIAN_POINT('Ctrl Pts',(72.5341913976221,202.567520362575,17.854339447693)) ;
#78627=CARTESIAN_POINT('Ctrl Pts',(72.5341913976221,202.567520362575,32.8747165227329)) ;
#78628=CARTESIAN_POINT('Ctrl Pts',(72.8081914673101,202.05583548982,17.854339447693)) ;
#78629=CARTESIAN_POINT('Ctrl Pts',(72.8081914673101,202.05583548982,32.8747165227329)) ;
#78630=CARTESIAN_POINT('Origin',(72.8081914673101,202.05583548982,23.8713203435596)) ;
#78631=CARTESIAN_POINT('Origin',(67.6088474917769,207.295232147432,19.3713203435596)) ;
#78632=CARTESIAN_POINT('Ctrl Pts',(66.6653986331397,202.05583548982,17.8547522895864)) ;
#78633=CARTESIAN_POINT('Ctrl Pts',(66.6653986331397,202.05583548982,32.8746339543542)) ;
#78634=CARTESIAN_POINT('Ctrl Pts',(64.7175672988148,205.239235006074,17.8547522895864)) ;
#78635=CARTESIAN_POINT('Ctrl Pts',(64.7175672988148,205.239235006074,32.8746339543542)) ;
#78636=CARTESIAN_POINT('Ctrl Pts',(63.3441806268929,208.750326110011,17.8547522895864)) ;
#78637=CARTESIAN_POINT('Ctrl Pts',(63.3441806268929,208.750326110011,32.8746339543542)) ;
#78638=CARTESIAN_POINT('Ctrl Pts',(62.4092970952969,212.53483522599,17.8547522895864)) ;
#78639=CARTESIAN_POINT('Ctrl Pts',(62.4092970952969,212.53483522599,32.8746339543542)) ;
#78640=CARTESIAN_POINT('Origin',(62.4092970952969,212.53483522599,23.8713203435596)) ;
#78641=CARTESIAN_POINT('Ctrl Pts',(70.3912832946837,219.697039770423,23.9913203435596)) ;
#78642=CARTESIAN_POINT('Ctrl Pts',(70.3892097227702,219.672192168808,23.9913203435596)) ;
#78643=CARTESIAN_POINT('Ctrl Pts',(70.3871361508568,219.647344567192,23.9913203435596)) ;
#78644=CARTESIAN_POINT('Ctrl Pts',(70.3850625789433,219.622496965577,23.9913203435596)) ;
#78645=CARTESIAN_POINT('Ctrl Pts',(70.3491825816751,219.192547142135,23.9913203435596)) ;
#78646=CARTESIAN_POINT('Ctrl Pts',(70.3215247358121,218.761924034176,23.9913203435596)) ;
#78647=CARTESIAN_POINT('Ctrl Pts',(70.3022814706893,218.330941191344,23.9913203435596)) ;
#78648=CARTESIAN_POINT('Ctrl Pts',(70.3912832946837,219.697039770423,23.9554164275186)) ;
#78649=CARTESIAN_POINT('Ctrl Pts',(70.3892097227702,219.672192168808,23.9554164275186)) ;
#78650=CARTESIAN_POINT('Ctrl Pts',(70.3871361508568,219.647344567192,23.9554164275186)) ;
#78651=CARTESIAN_POINT('Ctrl Pts',(70.3850625789433,219.622496965577,23.9554164275186)) ;
#78652=CARTESIAN_POINT('Ctrl Pts',(70.3491825816751,219.192547142135,23.9554164275186)) ;
#78653=CARTESIAN_POINT('Ctrl Pts',(70.3215247358121,218.761924034176,23.9554164275186)) ;
#78654=CARTESIAN_POINT('Ctrl Pts',(70.3022814706893,218.330941191344,23.9554164275186)) ;
#78655=CARTESIAN_POINT('Ctrl Pts',(70.3612291512671,219.699547836539,23.8932840823134)) ;
#78656=CARTESIAN_POINT('Ctrl Pts',(70.3591555793536,219.674700234924,23.8932840823134)) ;
#78657=CARTESIAN_POINT('Ctrl Pts',(70.3570820074401,219.649852633308,23.8932840823134)) ;
#78658=CARTESIAN_POINT('Ctrl Pts',(70.3550084355267,219.625005031693,23.8932840823134)) ;
#78659=CARTESIAN_POINT('Ctrl Pts',(70.3190964567053,219.194672012347,23.8932840823134)) ;
#78660=CARTESIAN_POINT('Ctrl Pts',(70.291413648541,218.763661470318,23.8932840823134)) ;
#78661=CARTESIAN_POINT('Ctrl Pts',(70.2721528749869,218.332286424837,23.8932840823134)) ;
#78662=CARTESIAN_POINT('Ctrl Pts',(70.2985336334945,219.704779877312,23.8713203435596)) ;
#78663=CARTESIAN_POINT('Ctrl Pts',(70.2964600615811,219.679932275696,23.8713203435596)) ;
#78664=CARTESIAN_POINT('Ctrl Pts',(70.2943864896676,219.655084674081,23.8713203435596)) ;
#78665=CARTESIAN_POINT('Ctrl Pts',(70.2923129177541,219.630237072465,23.8713203435596)) ;
#78666=CARTESIAN_POINT('Ctrl Pts',(70.2563342313308,219.199104680379,23.8713203435596)) ;
#78667=CARTESIAN_POINT('Ctrl Pts',(70.2285993496033,218.767285918537,23.8713203435596)) ;
#78668=CARTESIAN_POINT('Ctrl Pts',(70.2093020433682,218.335092697142,23.8713203435596)) ;
#78669=CARTESIAN_POINT('Ctrl Pts',(70.2716989748822,219.707019272295,23.8713203435596)) ;
#78670=CARTESIAN_POINT('Ctrl Pts',(70.2696254029687,219.68217167068,23.8713203435596)) ;
#78671=CARTESIAN_POINT('Ctrl Pts',(70.2675518310552,219.657324069064,23.8713203435596)) ;
#78672=CARTESIAN_POINT('Ctrl Pts',(70.2654782591418,219.632476467449,23.8713203435596)) ;
#78673=CARTESIAN_POINT('Ctrl Pts',(70.2294710222707,219.201001932498,23.8713203435596)) ;
#78674=CARTESIAN_POINT('Ctrl Pts',(70.201713852236,218.768837240123,23.8713203435596)) ;
#78675=CARTESIAN_POINT('Ctrl Pts',(70.1824009080094,218.33629382542,23.8713203435596)) ;
#78676=CARTESIAN_POINT('',(70.2716989748822,219.707019272295,23.8713203435596)) ;
#78677=CARTESIAN_POINT('',(70.3850625789433,219.622496965576,23.9913203435596)) ;
#78678=CARTESIAN_POINT('Ctrl Pts',(70.2716989748826,219.707019272295,23.8713203435596)) ;
#78679=CARTESIAN_POINT('Ctrl Pts',(70.2851494079172,219.696990818844,23.8713203435596)) ;
#78680=CARTESIAN_POINT('Ctrl Pts',(70.2987229692106,219.686870562696,23.8739545428452)) ;
#78681=CARTESIAN_POINT('Ctrl Pts',(70.3229190992498,219.668830268886,23.8835461747999)) ;
#78682=CARTESIAN_POINT('Ctrl Pts',(70.3361962896516,219.6589309827,23.8909151565592)) ;
#78683=CARTESIAN_POINT('Ctrl Pts',(70.3591097193747,219.641847052182,23.9136254788598)) ;
#78684=CARTESIAN_POINT('Ctrl Pts',(70.3679199332324,219.635278280804,23.9263737714492)) ;
#78685=CARTESIAN_POINT('Ctrl Pts',(70.377726918825,219.627966330455,23.9486436004895)) ;
#78686=CARTESIAN_POINT('Ctrl Pts',(70.380437698525,219.625945211286,23.9569014064467)) ;
#78687=CARTESIAN_POINT('Ctrl Pts',(70.3840992101215,219.623215239804,23.9739095905764)) ;
#78688=CARTESIAN_POINT('Ctrl Pts',(70.3850625789433,219.622496965577,23.98258579457)) ;
#78689=CARTESIAN_POINT('Ctrl Pts',(70.3850625789433,219.622496965577,23.9913203435596)) ;
#78690=CARTESIAN_POINT('',(70.3022814706893,218.330941191344,23.9913203435596)) ;
#78691=CARTESIAN_POINT('Origin',(103.767178705518,216.834469413397,23.9913203435596)) ;
#78692=CARTESIAN_POINT('',(70.1824009080094,218.33629382542,23.8713203435596)) ;
#78693=CARTESIAN_POINT('Origin',(70.1824009080094,218.33629382542,23.9913203435596)) ;
#78694=CARTESIAN_POINT('Ctrl Pts',(70.1824009080094,218.33629382542,23.8713203435596)) ;
#78695=CARTESIAN_POINT('Ctrl Pts',(70.201713852236,218.768837240123,23.8713203435596)) ;
#78696=CARTESIAN_POINT('Ctrl Pts',(70.2294710222707,219.201001932498,23.8713203435596)) ;
#78697=CARTESIAN_POINT('Ctrl Pts',(70.2675518310552,219.657324069064,23.8713203435596)) ;
#78698=CARTESIAN_POINT('Ctrl Pts',(70.2696254029687,219.68217167068,23.8713203435596)) ;
#78699=CARTESIAN_POINT('Ctrl Pts',(70.2716989748822,219.707019272295,23.8713203435596)) ;
#78700=CARTESIAN_POINT('Ctrl Pts',(70.3022814706893,218.330941191344,23.9913203435596)) ;
#78701=CARTESIAN_POINT('Ctrl Pts',(70.2676697182798,217.555757180025,23.9913203435596)) ;
#78702=CARTESIAN_POINT('Ctrl Pts',(70.2602736675229,216.779393400763,23.9913203435596)) ;
#78703=CARTESIAN_POINT('Ctrl Pts',(70.2813572214291,216.003852832276,23.9913203435596)) ;
#78704=CARTESIAN_POINT('Ctrl Pts',(70.3022814706893,218.330941191344,23.9554164275186)) ;
#78705=CARTESIAN_POINT('Ctrl Pts',(70.2676701188078,217.555766150471,23.9554164275186)) ;
#78706=CARTESIAN_POINT('Ctrl Pts',(70.2602739227663,216.779384011854,23.9554164275186)) ;
#78707=CARTESIAN_POINT('Ctrl Pts',(70.2813572214291,216.003852832276,23.9554164275186)) ;
#78708=CARTESIAN_POINT('Ctrl Pts',(70.2721528923875,218.33228642406,23.8932840614142)) ;
#78709=CARTESIAN_POINT('Ctrl Pts',(70.2375095501616,217.556394909683,23.8932840614142)) ;
#78710=CARTESIAN_POINT('Ctrl Pts',(70.2301060791862,216.779314330808,23.8932840614142)) ;
#78711=CARTESIAN_POINT('Ctrl Pts',(70.2512097642495,216.003033254856,23.8932840614142)) ;
#78712=CARTESIAN_POINT('Ctrl Pts',(70.2093020433682,218.335092697142,23.8713203435596)) ;
#78713=CARTESIAN_POINT('Ctrl Pts',(70.1745930291305,217.557730355953,23.8713203435596)) ;
#78714=CARTESIAN_POINT('Ctrl Pts',(70.1671739965509,216.779144060255,23.8713203435596)) ;
#78715=CARTESIAN_POINT('Ctrl Pts',(70.1883195322401,216.001323544686,23.8713203435596)) ;
#78716=CARTESIAN_POINT('Ctrl Pts',(70.1824009080094,218.33629382542,23.8713203435596)) ;
#78717=CARTESIAN_POINT('Ctrl Pts',(70.14766382781,217.558302903379,23.8713203435596)) ;
#78718=CARTESIAN_POINT('Ctrl Pts',(70.1402381191435,216.779070181469,23.8713203435596)) ;
#78719=CARTESIAN_POINT('Ctrl Pts',(70.1614015403524,216.000591762293,23.8713203435596)) ;
#78720=CARTESIAN_POINT('Origin',(99.3986297236392,223.018122277899,23.8713203435596)) ;
#78721=CARTESIAN_POINT('Origin',(99.1329946691538,222.962162901338,23.9913203435596)) ;
#78722=CARTESIAN_POINT('Ctrl Pts',(70.4779346423502,213.258471670562,23.8713203435596)) ;
#78723=CARTESIAN_POINT('Ctrl Pts',(70.4779346423502,213.258471670562,31.6713203435596)) ;
#78724=CARTESIAN_POINT('Ctrl Pts',(70.4761055561897,213.274084092013,23.8713203435596)) ;
#78725=CARTESIAN_POINT('Ctrl Pts',(70.4761055561897,213.274084092013,31.6713203435596)) ;
#78726=CARTESIAN_POINT('Ctrl Pts',(70.4123720009514,213.821196392358,23.8713203435596)) ;
#78727=CARTESIAN_POINT('Ctrl Pts',(70.4123720009514,213.821196392358,31.6713203435596)) ;
#78728=CARTESIAN_POINT('Ctrl Pts',(70.3612615606319,214.369323962879,23.8713203435596)) ;
#78729=CARTESIAN_POINT('Ctrl Pts',(70.3612615606319,214.369323962879,31.6713203435596)) ;
#78730=CARTESIAN_POINT('Ctrl Pts',(70.3225171301736,214.918446124758,23.8713203435596)) ;
#78731=CARTESIAN_POINT('Ctrl Pts',(70.3225171301736,214.918446124758,31.6713203435596)) ;
#78732=CARTESIAN_POINT('Ctrl Pts',(70.2959099128609,215.468544476001,23.8713203435596)) ;
#78733=CARTESIAN_POINT('Ctrl Pts',(70.2959099128609,215.468544476001,31.6713203435596)) ;
#78734=CARTESIAN_POINT('Ctrl Pts',(70.2813572214291,216.003852832275,23.8713203435596)) ;
#78735=CARTESIAN_POINT('Ctrl Pts',(70.2813572214291,216.003852832275,31.6713203435596)) ;
#78736=CARTESIAN_POINT('',(70.4779346423502,213.258471670562,23.8713203435596)) ;
#78737=CARTESIAN_POINT('',(70.2813572214291,216.003852832276,23.8713203435596)) ;
#78738=CARTESIAN_POINT('Ctrl Pts',(70.2813572214291,216.003852832276,23.8713203435596)) ;
#78739=CARTESIAN_POINT('Ctrl Pts',(70.2813572214291,216.003852832276,31.6713203435596)) ;
#78740=CARTESIAN_POINT('Ctrl Pts',(70.2788401464342,216.096441291563,23.8713203435596)) ;
#78741=CARTESIAN_POINT('Ctrl Pts',(70.2788401464342,216.096441291563,31.6713203435596)) ;
#78742=CARTESIAN_POINT('Ctrl Pts',(70.2679178621387,216.560643904903,23.8713203435596)) ;
#78743=CARTESIAN_POINT('Ctrl Pts',(70.2679178621387,216.560643904903,31.6713203435596)) ;
#78744=CARTESIAN_POINT('Ctrl Pts',(70.2654637030854,217.025527604889,23.8713203435596)) ;
#78745=CARTESIAN_POINT('Ctrl Pts',(70.2654637030854,217.025527604889,31.6713203435596)) ;
#78746=CARTESIAN_POINT('Ctrl Pts',(70.2713796878849,217.491084510933,23.8713203435596)) ;
#78747=CARTESIAN_POINT('Ctrl Pts',(70.2713796878849,217.491084510933,31.6713203435596)) ;
#78748=CARTESIAN_POINT('Ctrl Pts',(70.2855989071304,217.957309241547,23.8713203435596)) ;
#78749=CARTESIAN_POINT('Ctrl Pts',(70.2855989071304,217.957309241547,31.6713203435596)) ;
#78750=CARTESIAN_POINT('Ctrl Pts',(70.3022814706893,218.330941191344,23.8713203435596)) ;
#78751=CARTESIAN_POINT('Ctrl Pts',(70.3022814706893,218.330941191344,31.6713203435596)) ;
#78752=CARTESIAN_POINT('',(70.3022814706893,218.330941191344,23.8713203435596)) ;
#78753=CARTESIAN_POINT('Ctrl Pts',(70.3022814706893,218.330941191344,23.8713203435596)) ;
#78754=CARTESIAN_POINT('Ctrl Pts',(70.3022814706893,218.330941191344,31.6713203435596)) ;
#78755=CARTESIAN_POINT('Ctrl Pts',(70.3137968902541,218.588846917257,23.8713203435596)) ;
#78756=CARTESIAN_POINT('Ctrl Pts',(70.3137968902541,218.588846917257,31.6713203435596)) ;
#78757=CARTESIAN_POINT('Ctrl Pts',(70.3278377342262,218.846955761663,23.8713203435596)) ;
#78758=CARTESIAN_POINT('Ctrl Pts',(70.3278377342262,218.846955761663,31.6713203435596)) ;
#78759=CARTESIAN_POINT('Ctrl Pts',(70.3443973562324,219.105267189998,23.8713203435596)) ;
#78760=CARTESIAN_POINT('Ctrl Pts',(70.3443973562324,219.105267189998,31.6713203435596)) ;
#78761=CARTESIAN_POINT('Ctrl Pts',(70.3634723134982,219.363780925362,23.8713203435596)) ;
#78762=CARTESIAN_POINT('Ctrl Pts',(70.3634723134982,219.363780925362,31.6713203435596)) ;
#78763=CARTESIAN_POINT('Ctrl Pts',(70.3850625789433,219.622496965577,23.8713203435596)) ;
#78764=CARTESIAN_POINT('Ctrl Pts',(70.3850625789433,219.622496965577,31.6713203435596)) ;
#78765=CARTESIAN_POINT('',(70.3850625789433,219.622496965577,23.8713203435596)) ;
#78766=CARTESIAN_POINT('Origin',(70.3850625789433,219.622496965577,23.8713203435596)) ;
#78767=CARTESIAN_POINT('',(64.9830939940346,223.650128668,23.8713203435596)) ;
#78768=CARTESIAN_POINT('',(64.9830939940346,223.650128668,23.8713203435596)) ;
#78769=CARTESIAN_POINT('',(64.9830939940346,223.650128668,23.8713203435596)) ;
#78770=CARTESIAN_POINT('Origin',(60.9557289941889,214.062457729594,17.9913203435596)) ;
#78771=CARTESIAN_POINT('Origin',(60.9557289941889,214.062457729594,17.9913203435596)) ;
#78772=CARTESIAN_POINT('',(60.8531713625061,214.124762883342,17.9913203435596)) ;
#78773=CARTESIAN_POINT('Origin',(60.9557289941889,214.062457729594,17.9913203435596)) ;
#78774=CARTESIAN_POINT('Origin',(60.9557289941889,214.062457729594,17.9913203435596)) ;
#78775=CARTESIAN_POINT('Origin',(60.9557289910913,214.062457729895,17.9913203435596)) ;
#78776=CARTESIAN_POINT('Ctrl Pts',(60.9673257563026,214.181896061416,23.7513203435596)) ;
#78777=CARTESIAN_POINT('Ctrl Pts',(60.9673257563026,214.181896061416,16.8393203435596)) ;
#78778=CARTESIAN_POINT('Ctrl Pts',(60.9300677412812,214.185513596343,23.7513203435596)) ;
#78779=CARTESIAN_POINT('Ctrl Pts',(60.9300677412812,214.185513596343,16.8393203435596)) ;
#78780=CARTESIAN_POINT('Ctrl Pts',(60.8750422973704,214.163785096389,23.7513203435596)) ;
#78781=CARTESIAN_POINT('Ctrl Pts',(60.8750422973704,214.163785096389,16.8393203435596)) ;
#78782=CARTESIAN_POINT('Ctrl Pts',(60.8364976384102,214.097504784634,23.7513203435596)) ;
#78783=CARTESIAN_POINT('Ctrl Pts',(60.8364976384102,214.097504784634,16.8393203435596)) ;
#78784=CARTESIAN_POINT('Ctrl Pts',(60.8338841153326,214.059085002227,23.7513203435596)) ;
#78785=CARTESIAN_POINT('Ctrl Pts',(60.8338841153326,214.059085002227,16.8393203435596)) ;
#78786=CARTESIAN_POINT('Ctrl Pts',(60.8382191089243,214.038138460174,23.7513203435596)) ;
#78787=CARTESIAN_POINT('Ctrl Pts',(60.8382191089243,214.038138460174,16.8393203435596)) ;
#78788=CARTESIAN_POINT('Ctrl Pts',(61.1448474062677,212.657605881144,17.9913203435596)) ;
#78789=CARTESIAN_POINT('Ctrl Pts',(61.0358864187945,213.1162730929,17.9913203435596)) ;
#78790=CARTESIAN_POINT('Ctrl Pts',(60.9337505575544,213.576533739222,17.9913203435596)) ;
#78791=CARTESIAN_POINT('Ctrl Pts',(60.8382191077639,214.038138465781,17.9913203435596)) ;
#78792=CARTESIAN_POINT('Ctrl Pts',(61.1448474062677,212.657605881144,17.9554164275186)) ;
#78793=CARTESIAN_POINT('Ctrl Pts',(61.0358855397407,213.116276793244,17.9554164275186)) ;
#78794=CARTESIAN_POINT('Ctrl Pts',(60.9337512988544,213.576530157286,17.9554164275186)) ;
#78795=CARTESIAN_POINT('Ctrl Pts',(60.8382191077639,214.038138465781,17.9554164275186)) ;
#78796=CARTESIAN_POINT('Ctrl Pts',(61.1741891643601,212.664576309494,17.8932837582075)) ;
#78797=CARTESIAN_POINT('Ctrl Pts',(61.0652975082516,213.122951673457,17.8932837582075)) ;
#78798=CARTESIAN_POINT('Ctrl Pts',(60.9632246192255,213.582928155348,17.8932837582075)) ;
#78799=CARTESIAN_POINT('Ctrl Pts',(60.8677516360983,214.044250372973,17.8932837582075)) ;
#78800=CARTESIAN_POINT('Ctrl Pts',(61.2353993963615,212.679117412829,17.8713203435596)) ;
#78801=CARTESIAN_POINT('Ctrl Pts',(61.1266518731003,213.136886054948,17.8713203435596)) ;
#78802=CARTESIAN_POINT('Ctrl Pts',(61.0247112733278,213.596265593577,17.8713203435596)) ;
#78803=CARTESIAN_POINT('Ctrl Pts',(60.9293598364399,214.057000503894,17.8713203435596)) ;
#78804=CARTESIAN_POINT('Ctrl Pts',(61.2615982170329,212.685341204933,17.8713203435596)) ;
#78805=CARTESIAN_POINT('Ctrl Pts',(61.1529122911993,213.142850554979,17.8713203435596)) ;
#78806=CARTESIAN_POINT('Ctrl Pts',(61.0510284852321,213.601973819837,17.8713203435596)) ;
#78807=CARTESIAN_POINT('Ctrl Pts',(60.9557289930313,214.062457735187,17.8713203435596)) ;
#78808=CARTESIAN_POINT('Origin',(61.2615982170329,212.685341204933,17.9913203435596)) ;
#78809=CARTESIAN_POINT('Ctrl Pts',(65.2679705316376,202.055835489823,17.9913203435596)) ;
#78810=CARTESIAN_POINT('Ctrl Pts',(63.3524709375853,205.346379782453,17.9913203435596)) ;
#78811=CARTESIAN_POINT('Ctrl Pts',(62.0239099776425,208.957224782185,17.9913203435596)) ;
#78812=CARTESIAN_POINT('Ctrl Pts',(61.1448474062769,212.657605881106,17.9913203435596)) ;
#78813=CARTESIAN_POINT('Ctrl Pts',(65.2679705316376,202.055835489823,17.9554164275186)) ;
#78814=CARTESIAN_POINT('Ctrl Pts',(63.3524488993449,205.346417640882,17.9554164275186)) ;
#78815=CARTESIAN_POINT('Ctrl Pts',(62.0239170695688,208.957194928986,17.9554164275186)) ;
#78816=CARTESIAN_POINT('Ctrl Pts',(61.1448474062769,212.657605881106,17.9554164275186)) ;
#78817=CARTESIAN_POINT('Ctrl Pts',(65.2940343849798,202.071007843105,17.8932837406185)) ;
#78818=CARTESIAN_POINT('Ctrl Pts',(63.3802729567682,205.358566224537,17.8932837406185)) ;
#78819=CARTESIAN_POINT('Ctrl Pts',(62.0526923780858,208.966549742266,17.8932837406185)) ;
#78820=CARTESIAN_POINT('Ctrl Pts',(61.174189150107,212.664576306067,17.8932837406185)) ;
#78821=CARTESIAN_POINT('Ctrl Pts',(65.3484065753611,202.10265911394,17.8713203435596)) ;
#78822=CARTESIAN_POINT('Ctrl Pts',(63.4382586169361,205.384010090046,17.8713203435596)) ;
#78823=CARTESIAN_POINT('Ctrl Pts',(62.1127398064059,208.985985687741,17.8713203435596)) ;
#78824=CARTESIAN_POINT('Ctrl Pts',(61.2353993963707,212.67911741279,17.8713203435596)) ;
#78825=CARTESIAN_POINT('Ctrl Pts',(65.3716786148033,202.116206289769,17.8713203435596)) ;
#78826=CARTESIAN_POINT('Ctrl Pts',(63.4630749292305,205.394904434083,17.8713203435596)) ;
#78827=CARTESIAN_POINT('Ctrl Pts',(62.1384416786349,208.994301365774,17.8713203435596)) ;
#78828=CARTESIAN_POINT('Ctrl Pts',(61.2615982170421,212.685341204894,17.8713203435596)) ;
#78829=CARTESIAN_POINT('Origin',(65.3716786148033,202.116206289769,17.9913203435596)) ;
#78830=CARTESIAN_POINT('Ctrl Pts',(66.1952689412975,200.555835489821,17.9913203435596)) ;
#78831=CARTESIAN_POINT('Ctrl Pts',(65.8729833388596,201.047515223108,17.9913203435596)) ;
#78832=CARTESIAN_POINT('Ctrl Pts',(65.5637332147713,201.547759052751,17.9913203435596)) ;
#78833=CARTESIAN_POINT('Ctrl Pts',(65.2679705316394,202.05583548982,17.9913203435596)) ;
#78834=CARTESIAN_POINT('Ctrl Pts',(66.1952689412975,200.555835489821,17.9554164275186)) ;
#78835=CARTESIAN_POINT('Ctrl Pts',(65.872979631281,201.0475208794,17.9554164275186)) ;
#78836=CARTESIAN_POINT('Ctrl Pts',(65.5637366175855,201.547753207221,17.9554164275186)) ;
#78837=CARTESIAN_POINT('Ctrl Pts',(65.2679705316394,202.05583548982,17.9554164275186)) ;
#78838=CARTESIAN_POINT('Ctrl Pts',(66.2204915925578,200.572368400995,17.893283631872)) ;
#78839=CARTESIAN_POINT('Ctrl Pts',(65.8984984085001,201.063602020059,17.893283631872)) ;
#78840=CARTESIAN_POINT('Ctrl Pts',(65.5895286083177,201.563392400006,17.893283631872)) ;
#78841=CARTESIAN_POINT('Ctrl Pts',(65.2940343066537,202.071007797505,17.893283631872)) ;
#78842=CARTESIAN_POINT('Ctrl Pts',(66.2731091727483,200.60685810513,17.8713203435596)) ;
#78843=CARTESIAN_POINT('Ctrl Pts',(65.9517238967264,201.097164298152,17.8713203435596)) ;
#78844=CARTESIAN_POINT('Ctrl Pts',(65.6433429392842,201.596002170755,17.8713203435596)) ;
#78845=CARTESIAN_POINT('Ctrl Pts',(65.3484065753628,202.102659113937,17.8713203435596)) ;
#78846=CARTESIAN_POINT('Ctrl Pts',(66.2956301826422,200.621620147878,17.8713203435596)) ;
#78847=CARTESIAN_POINT('Ctrl Pts',(65.974504705631,201.111529990869,17.8713203435596)) ;
#78848=CARTESIAN_POINT('Ctrl Pts',(65.6663765353022,201.609958957032,17.8713203435596)) ;
#78849=CARTESIAN_POINT('Ctrl Pts',(65.371678614805,202.116206289766,17.8713203435596)) ;
#78850=CARTESIAN_POINT('Origin',(66.2956301826422,200.621620147878,17.9913203435596)) ;
#78851=CARTESIAN_POINT('Ctrl Pts',(77.1237619644425,189.518281677405,17.9913203435596)) ;
#78852=CARTESIAN_POINT('Ctrl Pts',(75.3192709150292,190.827610386593,17.9913203435596)) ;
#78853=CARTESIAN_POINT('Ctrl Pts',(71.2757417352347,194.115942691271,17.9913203435596)) ;
#78854=CARTESIAN_POINT('Ctrl Pts',(67.8274231206578,198.065816930128,17.9913203435596)) ;
#78855=CARTESIAN_POINT('Ctrl Pts',(66.1952689412979,200.55583548982,17.9913203435596)) ;
#78856=CARTESIAN_POINT('Ctrl Pts',(77.1237619644425,189.518281677405,17.9554164275186)) ;
#78857=CARTESIAN_POINT('Ctrl Pts',(75.3192591302046,190.827618937596,17.9554164275186)) ;
#78858=CARTESIAN_POINT('Ctrl Pts',(71.2757353479458,194.115940571234,17.9554164275186)) ;
#78859=CARTESIAN_POINT('Ctrl Pts',(67.8274418969853,198.065788284915,17.9554164275186)) ;
#78860=CARTESIAN_POINT('Ctrl Pts',(66.1952689412979,200.55583548982,17.9554164275186)) ;
#78861=CARTESIAN_POINT('Ctrl Pts',(77.1414733768851,189.542691197338,17.8932836220364)) ;
#78862=CARTESIAN_POINT('Ctrl Pts',(75.337911801841,190.851345485072,17.8932836220364)) ;
#78863=CARTESIAN_POINT('Ctrl Pts',(71.2966204784694,194.137907568835,17.8932836220364)) ;
#78864=CARTESIAN_POINT('Ctrl Pts',(67.8511648677532,198.084609097503,17.8932836220364)) ;
#78865=CARTESIAN_POINT('Ctrl Pts',(66.2204915857024,200.5723683965,17.8932836220364)) ;
#78866=CARTESIAN_POINT('Ctrl Pts',(77.1784215957542,189.59361250516,17.8713203435596)) ;
#78867=CARTESIAN_POINT('Ctrl Pts',(75.3767923032757,190.900864739369,17.8713203435596)) ;
#78868=CARTESIAN_POINT('Ctrl Pts',(71.340172504427,194.183727838921,17.8713203435596)) ;
#78869=CARTESIAN_POINT('Ctrl Pts',(67.9007038200928,198.123795579057,17.8713203435596)) ;
#78870=CARTESIAN_POINT('Ctrl Pts',(66.2731091727487,200.60685810513,17.8713203435596)) ;
#78871=CARTESIAN_POINT('Ctrl Pts',(77.1942359127805,189.615407485539,17.8713203435596)) ;
#78872=CARTESIAN_POINT('Ctrl Pts',(75.3934324114903,190.922060530236,17.8713203435596)) ;
#78873=CARTESIAN_POINT('Ctrl Pts',(71.3588126586277,194.203339283954,17.8713203435596)) ;
#78874=CARTESIAN_POINT('Ctrl Pts',(67.9219091272743,198.140564861203,17.8713203435596)) ;
#78875=CARTESIAN_POINT('Ctrl Pts',(66.2956301826426,200.621620147878,17.8713203435596)) ;
#78876=CARTESIAN_POINT('Origin',(77.1942359127805,189.615407485539,17.9913203435596)) ;
#78877=CARTESIAN_POINT('Ctrl Pts',(77.1942359127805,189.615407485539,17.8713203435596)) ;
#78878=CARTESIAN_POINT('Ctrl Pts',(77.3771291752412,189.482701147464,17.8713203435596)) ;
#78879=CARTESIAN_POINT('Ctrl Pts',(77.602534818386,189.409539758744,17.8713203435596)) ;
#78880=CARTESIAN_POINT('Ctrl Pts',(77.8285014478222,189.409539758744,17.8713203435596)) ;
#78881=CARTESIAN_POINT('Ctrl Pts',(77.1731501567454,189.5863475117,17.8713203435596)) ;
#78882=CARTESIAN_POINT('Ctrl Pts',(77.3621499339522,189.449210320354,17.8713203435596)) ;
#78883=CARTESIAN_POINT('Ctrl Pts',(77.5949901525182,189.373635842703,17.8713203435596)) ;
#78884=CARTESIAN_POINT('Ctrl Pts',(77.8285014478222,189.373635842703,17.8713203435596)) ;
#78885=CARTESIAN_POINT('Ctrl Pts',(77.1366606256317,189.536058358312,17.9014785774642)) ;
#78886=CARTESIAN_POINT('Ctrl Pts',(77.3361495975408,189.391310265396,17.9014785774642)) ;
#78887=CARTESIAN_POINT('Ctrl Pts',(77.5820306375505,189.311503042755,17.9014785774642)) ;
#78888=CARTESIAN_POINT('Ctrl Pts',(77.8285014478223,189.311503042755,17.9014785774642)) ;
#78889=CARTESIAN_POINT('Ctrl Pts',(77.1237619644425,189.518281677405,17.9643924065289)) ;
#78890=CARTESIAN_POINT('Ctrl Pts',(77.3269932166768,189.370818206616,17.9643924065289)) ;
#78891=CARTESIAN_POINT('Ctrl Pts',(77.5774070092107,189.289539758744,17.9643924065289)) ;
#78892=CARTESIAN_POINT('Ctrl Pts',(77.8285014478222,189.289539758744,17.9643924065289)) ;
#78893=CARTESIAN_POINT('Ctrl Pts',(77.1237619644425,189.518281677405,17.9913203435596)) ;
#78894=CARTESIAN_POINT('Ctrl Pts',(77.3269767005103,189.370830190655,17.9913203435596)) ;
#78895=CARTESIAN_POINT('Ctrl Pts',(77.5774274151154,189.289539758744,17.9913203435596)) ;
#78896=CARTESIAN_POINT('Ctrl Pts',(77.8285014478222,189.289539758744,17.9913203435596)) ;
#78897=CARTESIAN_POINT('',(77.8285014478222,189.289539758744,17.9913203435596)) ;
#78898=CARTESIAN_POINT('Origin',(77.8285014478222,189.409539758744,17.9913203435596)) ;
#78899=CARTESIAN_POINT('Origin',(77.7368311963088,190.20710947193,17.9913203435596)) ;
#78900=CARTESIAN_POINT('Origin',(71.6000791389318,189.409539758744,17.9913203435596)) ;
#78901=CARTESIAN_POINT('',(83.2194473860051,189.289539758744,17.9913203435596)) ;
#78902=CARTESIAN_POINT('Origin',(83.2194473860051,189.409539758744,17.9913203435596)) ;
#78903=CARTESIAN_POINT('',(71.6000791389318,189.289539758744,17.9913203435596)) ;
#78904=CARTESIAN_POINT('Ctrl Pts',(83.2194473860051,189.409539758744,17.8713203435596)) ;
#78905=CARTESIAN_POINT('Ctrl Pts',(83.3047606779792,189.409539758744,17.8713203435596)) ;
#78906=CARTESIAN_POINT('Ctrl Pts',(83.4319242412693,189.454563257398,17.8713203435596)) ;
#78907=CARTESIAN_POINT('Ctrl Pts',(83.5764307889551,189.615888430006,17.8713203435596)) ;
#78908=CARTESIAN_POINT('Ctrl Pts',(83.6266013556018,189.835500488137,17.8713203435596)) ;
#78909=CARTESIAN_POINT('Ctrl Pts',(83.5482147548371,189.998322839904,17.8713203435596)) ;
#78910=CARTESIAN_POINT('Ctrl Pts',(83.4878143389934,190.058573545737,17.8713203435596)) ;
#78911=CARTESIAN_POINT('Ctrl Pts',(83.2194473860051,189.373635842703,17.8713203435596)) ;
#78912=CARTESIAN_POINT('Ctrl Pts',(83.3128563436082,189.373635842703,17.8713203435596)) ;
#78913=CARTESIAN_POINT('Ctrl Pts',(83.452045237747,189.422831326517,17.8713203435596)) ;
#78914=CARTESIAN_POINT('Ctrl Pts',(83.6102461518883,189.599420760862,17.8713203435596)) ;
#78915=CARTESIAN_POINT('Ctrl Pts',(83.6651611847245,189.83983301376,17.8713203435596)) ;
#78916=CARTESIAN_POINT('Ctrl Pts',(83.5793027341283,190.018024833018,17.8713203435596)) ;
#78917=CARTESIAN_POINT('Ctrl Pts',(83.5131707193836,190.083992931264,17.8713203435596)) ;
#78918=CARTESIAN_POINT('Ctrl Pts',(83.2194473860052,189.311503153976,17.9014786701593)) ;
#78919=CARTESIAN_POINT('Ctrl Pts',(83.3267623139629,189.311503153976,17.9014786701593)) ;
#78920=CARTESIAN_POINT('Ctrl Pts',(83.4867304273842,189.368162111536,17.9014786701593)) ;
#78921=CARTESIAN_POINT('Ctrl Pts',(83.6685085212826,189.571102519156,17.9014786701593)) ;
#78922=CARTESIAN_POINT('Ctrl Pts',(83.7316216438234,189.847360366321,17.9014786701593)) ;
#78923=CARTESIAN_POINT('Ctrl Pts',(83.6330278294468,190.052192963681,17.9014786701593)) ;
#78924=CARTESIAN_POINT('Ctrl Pts',(83.5570506150538,190.127981859013,17.9014786701593)) ;
#78925=CARTESIAN_POINT('Ctrl Pts',(83.2194473860051,189.289539758744,17.9643924065289)) ;
#78926=CARTESIAN_POINT('Ctrl Pts',(83.3317236137326,189.289539758744,17.9643924065289)) ;
#78927=CARTESIAN_POINT('Ctrl Pts',(83.4990506182369,189.348729786032,17.9643924065289)) ;
#78928=CARTESIAN_POINT('Ctrl Pts',(83.6892163988353,189.561013301822,17.9643924065289)) ;
#78929=CARTESIAN_POINT('Ctrl Pts',(83.755232904682,189.850008116062,17.9643924065289)) ;
#78930=CARTESIAN_POINT('Ctrl Pts',(83.6520515313444,190.064238875503,17.9643924065289)) ;
#78931=CARTESIAN_POINT('Ctrl Pts',(83.5725617978318,190.143531583735,17.9643924065289)) ;
#78932=CARTESIAN_POINT('Ctrl Pts',(83.2194473860051,189.289539758744,17.9913203435596)) ;
#78933=CARTESIAN_POINT('Ctrl Pts',(83.33170171755,189.289539758744,17.9913203435596)) ;
#78934=CARTESIAN_POINT('Ctrl Pts',(83.4990221955632,189.348781204342,17.9913203435596)) ;
#78935=CARTESIAN_POINT('Ctrl Pts',(83.6891623898867,189.5610511683,17.9913203435596)) ;
#78936=CARTESIAN_POINT('Ctrl Pts',(83.7551762933692,189.850014402682,17.9913203435596)) ;
#78937=CARTESIAN_POINT('Ctrl Pts',(83.6520360292051,190.064254339218,17.9913203435596)) ;
#78938=CARTESIAN_POINT('Ctrl Pts',(83.5725617978318,190.143531583735,17.9913203435596)) ;
#78939=CARTESIAN_POINT('',(83.5725617978318,190.143531583735,17.9913203435596)) ;
#78940=CARTESIAN_POINT('Origin',(83.4878143389934,190.058573545737,17.9913203435596)) ;
#78941=CARTESIAN_POINT('Ctrl Pts',(83.5725617978318,190.143531583735,17.9913203435596)) ;
#78942=CARTESIAN_POINT('Ctrl Pts',(83.6520392110072,190.064251165302,17.9913203435596)) ;
#78943=CARTESIAN_POINT('Ctrl Pts',(83.7551748851088,189.850164868248,17.9913203435596)) ;
#78944=CARTESIAN_POINT('Ctrl Pts',(83.6762811453293,189.502581007553,17.9913203435596)) ;
#78945=CARTESIAN_POINT('Ctrl Pts',(83.4441273250624,189.317541444415,17.9913203435596)) ;
#78946=CARTESIAN_POINT('Ctrl Pts',(83.2755767988648,189.289539758744,17.9913203435596)) ;
#78947=CARTESIAN_POINT('Ctrl Pts',(83.2194473860051,189.289539758744,17.9913203435596)) ;
#78948=CARTESIAN_POINT('Ctrl Pts',(74.1761041106884,202.05583548982,17.9913203435596)) ;
#78949=CARTESIAN_POINT('Ctrl Pts',(75.2361074248711,200.159916764409,17.9913203435596)) ;
#78950=CARTESIAN_POINT('Ctrl Pts',(78.1041044154073,195.960565221311,17.9913203435596)) ;
#78951=CARTESIAN_POINT('Ctrl Pts',(81.5183138237629,192.192687846391,17.9913203435596)) ;
#78952=CARTESIAN_POINT('Ctrl Pts',(83.5725617978318,190.143531583735,17.9913203435596)) ;
#78953=CARTESIAN_POINT('Ctrl Pts',(74.1761041106884,202.05583548982,17.9554164275186)) ;
#78954=CARTESIAN_POINT('Ctrl Pts',(75.2360961966516,200.159936847168,17.9554164275186)) ;
#78955=CARTESIAN_POINT('Ctrl Pts',(78.1040924841332,195.960587192884,17.9554164275186)) ;
#78956=CARTESIAN_POINT('Ctrl Pts',(81.5183233608015,192.192678332992,17.9554164275186)) ;
#78957=CARTESIAN_POINT('Ctrl Pts',(83.5725617978318,190.143531583735,17.9554164275186)) ;
#78958=CARTESIAN_POINT('Ctrl Pts',(74.1497806371692,202.041118103047,17.8932837799342)) ;
#78959=CARTESIAN_POINT('Ctrl Pts',(75.2106695260217,200.143615441457,17.8932837799342)) ;
#78960=CARTESIAN_POINT('Ctrl Pts',(78.0806203331662,195.941491968631,17.8932837799342)) ;
#78961=CARTESIAN_POINT('Ctrl Pts',(81.4962629295466,192.172086546055,17.8932837799342)) ;
#78962=CARTESIAN_POINT('Ctrl Pts',(83.5512630940976,190.122179957315,17.8932837799342)) ;
#78963=CARTESIAN_POINT('Ctrl Pts',(74.0948669375562,202.010415993931,17.8713203435596)) ;
#78964=CARTESIAN_POINT('Ctrl Pts',(75.1575968459697,200.109620490316,17.8713203435596)) ;
#78965=CARTESIAN_POINT('Ctrl Pts',(78.0316231323412,195.901715537708,17.8713203435596)) ;
#78966=CARTESIAN_POINT('Ctrl Pts',(81.4502677323176,192.129104525146,17.8713203435596)) ;
#78967=CARTESIAN_POINT('Ctrl Pts',(83.506831624286,190.077638084882,17.8713203435596)) ;
#78968=CARTESIAN_POINT('Ctrl Pts',(74.071363112532,201.997275065426,17.8713203435596)) ;
#78969=CARTESIAN_POINT('Ctrl Pts',(75.1348798094609,200.095072314249,17.8713203435596)) ;
#78970=CARTESIAN_POINT('Ctrl Pts',(78.0106503827396,195.884693008864,17.8713203435596)) ;
#78971=CARTESIAN_POINT('Ctrl Pts',(81.4305821636459,192.110706612955,17.8713203435596)) ;
#78972=CARTESIAN_POINT('Ctrl Pts',(83.4878143389934,190.058573545737,17.8713203435596)) ;
#78973=CARTESIAN_POINT('',(74.1761041106884,202.05583548982,17.9913203435596)) ;
#78974=CARTESIAN_POINT('Origin',(74.071363112532,201.997275065426,17.9913203435596)) ;
#78975=CARTESIAN_POINT('Ctrl Pts',(74.1761041106884,202.05583548982,17.9913203435596)) ;
#78976=CARTESIAN_POINT('Ctrl Pts',(74.2838092722993,201.863194363147,17.9913203435596)) ;
#78977=CARTESIAN_POINT('Ctrl Pts',(74.7358054436199,201.068974645156,17.9913203435596)) ;
#78978=CARTESIAN_POINT('Ctrl Pts',(75.5850166034805,199.677432982293,17.9913203435596)) ;
#78979=CARTESIAN_POINT('Ctrl Pts',(76.933494947875,197.696777376424,17.9913203435596)) ;
#78980=CARTESIAN_POINT('Ctrl Pts',(78.784019206408,195.312002858836,17.9913203435596)) ;
#78981=CARTESIAN_POINT('Ctrl Pts',(80.6886895533707,193.132887074724,17.9913203435596)) ;
#78982=CARTESIAN_POINT('Ctrl Pts',(82.1803361041117,191.549821741792,17.9913203435596)) ;
#78983=CARTESIAN_POINT('Ctrl Pts',(83.16020700552,190.554864302944,17.9913203435596)) ;
#78984=CARTESIAN_POINT('Ctrl Pts',(83.5725617978318,190.143531583735,17.9913203435596)) ;
#78985=CARTESIAN_POINT('Ctrl Pts',(70.5067868147823,213.020459099211,17.9913203435596)) ;
#78986=CARTESIAN_POINT('Ctrl Pts',(70.7134450664337,211.371105542151,17.9913203435596)) ;
#78987=CARTESIAN_POINT('Ctrl Pts',(71.5202034275434,207.561661620558,17.9913203435596)) ;
#78988=CARTESIAN_POINT('Ctrl Pts',(73.0937605573685,203.991711899461,17.9913203435596)) ;
#78989=CARTESIAN_POINT('Ctrl Pts',(74.1761041106882,202.05583548982,17.9913203435596)) ;
#78990=CARTESIAN_POINT('Ctrl Pts',(70.5067868147823,213.020459099211,17.9554164275186)) ;
#78991=CARTESIAN_POINT('Ctrl Pts',(70.7134424086352,211.371126754222,17.9554164275186)) ;
#78992=CARTESIAN_POINT('Ctrl Pts',(71.5202054125703,207.561684097306,17.9554164275186)) ;
#78993=CARTESIAN_POINT('Ctrl Pts',(73.0937720222297,203.991691393444,17.9554164275186)) ;
#78994=CARTESIAN_POINT('Ctrl Pts',(74.1761041106882,202.05583548982,17.9554164275186)) ;
#78995=CARTESIAN_POINT('Ctrl Pts',(70.4768623382484,213.016709666608,17.8932838954934)) ;
#78996=CARTESIAN_POINT('Ctrl Pts',(70.6837302116549,211.365683104068,17.8932838954934)) ;
#78997=CARTESIAN_POINT('Ctrl Pts',(71.4913439175855,207.552164797002,17.8932838954934)) ;
#78998=CARTESIAN_POINT('Ctrl Pts',(73.0665327610701,203.978611784322,17.8932838954934)) ;
#78999=CARTESIAN_POINT('Ctrl Pts',(74.149780553105,202.041118056048,17.8932838954934)) ;
#79000=CARTESIAN_POINT('Ctrl Pts',(70.4144368399205,213.00888796926,17.8713203435596)) ;
#79001=CARTESIAN_POINT('Ctrl Pts',(70.6217404956101,211.354383398689,17.8713203435596)) ;
#79002=CARTESIAN_POINT('Ctrl Pts',(71.4311411755023,207.532366228087,17.8713203435596)) ;
#79003=CARTESIAN_POINT('Ctrl Pts',(73.0097393253103,203.951271962955,17.8713203435596)) ;
#79004=CARTESIAN_POINT('Ctrl Pts',(74.0948669375559,202.010415993931,17.8713203435596)) ;
#79005=CARTESIAN_POINT('Ctrl Pts',(70.3877178199639,213.005540169192,17.8713203435596)) ;
#79006=CARTESIAN_POINT('Ctrl Pts',(70.5952077140308,211.34954921747,17.8713203435596)) ;
#79007=CARTESIAN_POINT('Ctrl Pts',(71.4053737386935,207.523894544389,17.8713203435596)) ;
#79008=CARTESIAN_POINT('Ctrl Pts',(72.9854321297061,203.939567940643,17.8713203435596)) ;
#79009=CARTESIAN_POINT('Ctrl Pts',(74.0713631125318,201.997275065426,17.8713203435596)) ;
#79010=CARTESIAN_POINT('Origin',(70.3877178199639,213.005540169192,17.9913203435596)) ;
#79011=CARTESIAN_POINT('Ctrl Pts',(70.5067868147823,213.020459099211,17.9913203435596)) ;
#79012=CARTESIAN_POINT('Ctrl Pts',(70.7134450664337,211.371105542151,17.9913203435596)) ;
#79013=CARTESIAN_POINT('Ctrl Pts',(71.5202034275434,207.561661620558,17.9913203435596)) ;
#79014=CARTESIAN_POINT('Ctrl Pts',(73.0937605573685,203.991711899461,17.9913203435596)) ;
#79015=CARTESIAN_POINT('Ctrl Pts',(74.1761041106882,202.05583548982,17.9913203435596)) ;
#79016=CARTESIAN_POINT('Ctrl Pts',(70.3877178199639,213.005540169192,17.8713203435596)) ;
#79017=CARTESIAN_POINT('Ctrl Pts',(70.3834041808396,213.039967616326,17.8713203435596)) ;
#79018=CARTESIAN_POINT('Ctrl Pts',(70.3494702400649,213.117382991064,17.8713203435596)) ;
#79019=CARTESIAN_POINT('Ctrl Pts',(70.2725551198838,213.157848509207,17.8713203435596)) ;
#79020=CARTESIAN_POINT('Ctrl Pts',(70.2265094709067,213.162319271896,17.8713203435596)) ;
#79021=CARTESIAN_POINT('Ctrl Pts',(70.423343179906,213.010003902616,17.8713203435596)) ;
#79022=CARTESIAN_POINT('Ctrl Pts',(70.4181653875406,213.05132821552,17.8713203435596)) ;
#79023=CARTESIAN_POINT('Ctrl Pts',(70.3774821996608,213.144204826472,17.8713203435596)) ;
#79024=CARTESIAN_POINT('Ctrl Pts',(70.2852492082989,213.192688744648,17.8713203435596)) ;
#79025=CARTESIAN_POINT('Ctrl Pts',(70.2299792140174,213.198055137211,17.8713203435596)) ;
#79026=CARTESIAN_POINT('Ctrl Pts',(70.4849936629844,213.017728493254,17.9014788019101)) ;
#79027=CARTESIAN_POINT('Ctrl Pts',(70.4783315097396,213.070899591259,17.9014788019101)) ;
#79028=CARTESIAN_POINT('Ctrl Pts',(70.425910882421,213.190474327809,17.9014788019101)) ;
#79029=CARTESIAN_POINT('Ctrl Pts',(70.307098386221,213.252992031279,17.9014788019101)) ;
#79030=CARTESIAN_POINT('Ctrl Pts',(70.2359836821624,213.259896852312,17.9014788019101)) ;
#79031=CARTESIAN_POINT('Ctrl Pts',(70.5067868147823,213.020459099211,17.9643924065289)) ;
#79032=CARTESIAN_POINT('Ctrl Pts',(70.4995950789841,213.077856831581,17.9643924065289)) ;
#79033=CARTESIAN_POINT('Ctrl Pts',(70.4430506906804,213.206894672446,17.9643924065289)) ;
#79034=CARTESIAN_POINT('Ctrl Pts',(70.3148739302152,213.274303910178,17.9643924065289)) ;
#79035=CARTESIAN_POINT('Ctrl Pts',(70.2381062330204,213.281757603718,17.9643924065289)) ;
#79036=CARTESIAN_POINT('Ctrl Pts',(70.5067868147823,213.020459099211,17.9913203435596)) ;
#79037=CARTESIAN_POINT('Ctrl Pts',(70.4995974162418,213.077838177768,17.9913203435596)) ;
#79038=CARTESIAN_POINT('Ctrl Pts',(70.4430408482841,213.206863802331,17.9913203435596)) ;
#79039=CARTESIAN_POINT('Ctrl Pts',(70.3148489813156,213.27430633257,17.9913203435596)) ;
#79040=CARTESIAN_POINT('Ctrl Pts',(70.2381062330204,213.281757603718,17.9913203435596)) ;
#79041=CARTESIAN_POINT('Origin',(70.2265094709067,213.162319271896,17.9913203435596)) ;
#79042=CARTESIAN_POINT('Origin',(67.5325794977657,213.423884085911,17.9913203435596)) ;
#79043=CARTESIAN_POINT('Origin',(77.4412221473412,189.289539758744,23.8713203435596)) ;
#79044=CARTESIAN_POINT('',(77.8285014478222,189.289539758744,17.9913203435596)) ;
#79045=CARTESIAN_POINT('',(83.2194473860052,189.289539758744,30.2513203435596)) ;
#79046=CARTESIAN_POINT('Ctrl Pts',(83.5725617978318,190.143531583735,17.9913203435596)) ;
#79047=CARTESIAN_POINT('Ctrl Pts',(83.5725617978318,190.143531583735,32.7033203435596)) ;
#79048=CARTESIAN_POINT('Ctrl Pts',(83.6520392110072,190.064251165302,17.9913203435596)) ;
#79049=CARTESIAN_POINT('Ctrl Pts',(83.6520392110072,190.064251165302,32.7033203435596)) ;
#79050=CARTESIAN_POINT('Ctrl Pts',(83.7551748851088,189.850164868248,17.9913203435596)) ;
#79051=CARTESIAN_POINT('Ctrl Pts',(83.7551748851088,189.850164868248,32.7033203435596)) ;
#79052=CARTESIAN_POINT('Ctrl Pts',(83.6762811453293,189.502581007553,17.9913203435596)) ;
#79053=CARTESIAN_POINT('Ctrl Pts',(83.6762811453293,189.502581007553,32.7033203435596)) ;
#79054=CARTESIAN_POINT('Ctrl Pts',(83.4441273250624,189.317541444415,17.9913203435596)) ;
#79055=CARTESIAN_POINT('Ctrl Pts',(83.4441273250624,189.317541444415,32.7033203435596)) ;
#79056=CARTESIAN_POINT('Ctrl Pts',(83.2755767988648,189.289539758744,17.9913203435596)) ;
#79057=CARTESIAN_POINT('Ctrl Pts',(83.2755767988648,189.289539758744,32.7033203435596)) ;
#79058=CARTESIAN_POINT('Ctrl Pts',(83.2194473860051,189.289539758744,17.9913203435596)) ;
#79059=CARTESIAN_POINT('Ctrl Pts',(83.2194473860051,189.289539758744,32.7033203435596)) ;
#79060=CARTESIAN_POINT('',(83.5725617978318,190.143531583735,17.9913203435596)) ;
#79061=CARTESIAN_POINT('Ctrl Pts',(84.4412221473412,189.289539758744,17.8713203435596)) ;
#79062=CARTESIAN_POINT('Ctrl Pts',(84.4412221473412,189.289539758744,32.8713203435596)) ;
#79063=CARTESIAN_POINT('Ctrl Pts',(83.8416464716194,189.870585945118,17.8713203435596)) ;
#79064=CARTESIAN_POINT('Ctrl Pts',(83.8416464716194,189.870585945118,32.8713203435596)) ;
#79065=CARTESIAN_POINT('Ctrl Pts',(82.6693997344123,191.034842241154,17.8713203435596)) ;
#79066=CARTESIAN_POINT('Ctrl Pts',(82.6693997344123,191.034842241154,32.8713203435596)) ;
#79067=CARTESIAN_POINT('Ctrl Pts',(80.9917381958488,192.787718030768,17.8713203435596)) ;
#79068=CARTESIAN_POINT('Ctrl Pts',(80.9917381958488,192.787718030768,32.8713203435596)) ;
#79069=CARTESIAN_POINT('Ctrl Pts',(78.9189744912756,195.138085698398,17.8713203435596)) ;
#79070=CARTESIAN_POINT('Ctrl Pts',(78.9189744912756,195.138085698398,32.8713203435596)) ;
#79071=CARTESIAN_POINT('Ctrl Pts',(76.933494947875,197.696777376424,17.8713203435596)) ;
#79072=CARTESIAN_POINT('Ctrl Pts',(76.933494947875,197.696777376424,32.8713203435596)) ;
#79073=CARTESIAN_POINT('Ctrl Pts',(75.5850166034805,199.677432982293,17.8713203435596)) ;
#79074=CARTESIAN_POINT('Ctrl Pts',(75.5850166034805,199.677432982293,32.8713203435596)) ;
#79075=CARTESIAN_POINT('Ctrl Pts',(74.7358054436199,201.068974645156,17.8713203435596)) ;
#79076=CARTESIAN_POINT('Ctrl Pts',(74.7358054436199,201.068974645156,32.8713203435596)) ;
#79077=CARTESIAN_POINT('Ctrl Pts',(74.2838092722993,201.863194363147,17.8713203435596)) ;
#79078=CARTESIAN_POINT('Ctrl Pts',(74.2838092722993,201.863194363147,32.8713203435596)) ;
#79079=CARTESIAN_POINT('Ctrl Pts',(74.1761041106884,202.05583548982,17.8713203435596)) ;
#79080=CARTESIAN_POINT('Ctrl Pts',(74.1761041106884,202.05583548982,32.8713203435596)) ;
#79081=CARTESIAN_POINT('',(74.1761041106884,202.05583548982,23.8713203435596)) ;
#79082=CARTESIAN_POINT('Ctrl Pts',(74.1761041106882,202.05583548982,17.8713203435596)) ;
#79083=CARTESIAN_POINT('Ctrl Pts',(74.1761041106882,202.05583548982,32.8713203435596)) ;
#79084=CARTESIAN_POINT('Ctrl Pts',(73.9471261103511,202.465384849466,17.8713203435596)) ;
#79085=CARTESIAN_POINT('Ctrl Pts',(73.9471261103511,202.465384849466,32.8713203435596)) ;
#79086=CARTESIAN_POINT('Ctrl Pts',(73.4020528825475,203.478780571653,17.8713203435596)) ;
#79087=CARTESIAN_POINT('Ctrl Pts',(73.4020528825475,203.478780571653,32.8713203435596)) ;
#79088=CARTESIAN_POINT('Ctrl Pts',(72.6149447082149,205.101979283954,17.8713203435596)) ;
#79089=CARTESIAN_POINT('Ctrl Pts',(72.6149447082149,205.101979283954,32.8713203435596)) ;
#79090=CARTESIAN_POINT('Ctrl Pts',(71.7263234125876,207.330523545477,17.8713203435596)) ;
#79091=CARTESIAN_POINT('Ctrl Pts',(71.7263234125876,207.330523545477,32.8713203435596)) ;
#79092=CARTESIAN_POINT('Ctrl Pts',(71.0883402872662,209.579226496892,17.8713203435596)) ;
#79093=CARTESIAN_POINT('Ctrl Pts',(71.0883402872662,209.579226496892,32.8713203435596)) ;
#79094=CARTESIAN_POINT('Ctrl Pts',(70.7249576044374,211.422049476544,17.8713203435596)) ;
#79095=CARTESIAN_POINT('Ctrl Pts',(70.7249576044374,211.422049476544,32.8713203435596)) ;
#79096=CARTESIAN_POINT('Ctrl Pts',(70.5491399848247,212.650688483389,17.8713203435596)) ;
#79097=CARTESIAN_POINT('Ctrl Pts',(70.5491399848247,212.650688483389,32.8713203435596)) ;
#79098=CARTESIAN_POINT('Ctrl Pts',(70.4779346423502,213.258471670562,17.8713203435596)) ;
#79099=CARTESIAN_POINT('Ctrl Pts',(70.4779346423502,213.258471670562,32.8713203435596)) ;
#79100=CARTESIAN_POINT('Origin',(69.1686691234544,219.464553538579,23.8713203435596)) ;
#79101=CARTESIAN_POINT('',(68.8712529610467,219.761969700987,23.8713203435596)) ;
#79102=CARTESIAN_POINT('',(70.8292893218811,217.803933340152,23.8713203435596)) ;
#79103=CARTESIAN_POINT('',(68.8712529610467,219.761969700987,23.8713203435596)) ;
#79104=CARTESIAN_POINT('Ctrl Pts',(62.0562434701708,214.076168533126,23.8713203435596)) ;
#79105=CARTESIAN_POINT('Ctrl Pts',(62.0562434701708,214.076168533126,31.6713203435596)) ;
#79106=CARTESIAN_POINT('Ctrl Pts',(61.9621987792398,214.520814350555,23.8713203435596)) ;
#79107=CARTESIAN_POINT('Ctrl Pts',(61.9621987792398,214.520814350555,31.6713203435596)) ;
#79108=CARTESIAN_POINT('Ctrl Pts',(61.8739898282105,214.96907079501,23.8713203435596)) ;
#79109=CARTESIAN_POINT('Ctrl Pts',(61.8739898282105,214.96907079501,31.6713203435596)) ;
#79110=CARTESIAN_POINT('Ctrl Pts',(61.7916108526749,215.420902931566,23.8713203435596)) ;
#79111=CARTESIAN_POINT('Ctrl Pts',(61.7916108526749,215.420902931566,31.6713203435596)) ;
#79112=CARTESIAN_POINT('',(61.9703773266185,214.491161471122,30.2513203435596)) ;
#79113=CARTESIAN_POINT('Ctrl Pts',(61.9703773266185,214.491161471122,26.4913203435596)) ;
#79114=CARTESIAN_POINT('Ctrl Pts',(61.9703773266185,214.491161471122,31.0033203435596)) ;
#79115=CARTESIAN_POINT('Ctrl Pts',(61.8515957900547,215.078199641461,26.4913203435596)) ;
#79116=CARTESIAN_POINT('Ctrl Pts',(61.8515957900547,215.078199641461,31.0033203435596)) ;
#79117=CARTESIAN_POINT('Ctrl Pts',(61.7916108526749,215.677118589864,26.4913203435596)) ;
#79118=CARTESIAN_POINT('Ctrl Pts',(61.7916108526749,215.677118589864,31.0033203435596)) ;
#79119=CARTESIAN_POINT('Ctrl Pts',(61.7916108526749,216.276053366666,26.4913203435596)) ;
#79120=CARTESIAN_POINT('Ctrl Pts',(61.7916108526749,216.276053366666,31.0033203435596)) ;
#79121=CARTESIAN_POINT('',(61.7916108526749,216.276053366666,26.4913203435596)) ;
#79122=CARTESIAN_POINT('Ctrl Pts',(69.2315751790255,211.872432002476,23.4913203435596)) ;
#79123=CARTESIAN_POINT('Ctrl Pts',(69.2315751790255,211.872432002476,31.6033203435596)) ;
#79124=CARTESIAN_POINT('Ctrl Pts',(69.305984945383,211.865207250202,23.4913203435596)) ;
#79125=CARTESIAN_POINT('Ctrl Pts',(69.305984945383,211.865207250202,31.6033203435596)) ;
#79126=CARTESIAN_POINT('Ctrl Pts',(69.4305433706759,211.801563422573,23.4913203435596)) ;
#79127=CARTESIAN_POINT('Ctrl Pts',(69.4305433706759,211.801563422573,31.6033203435596)) ;
#79128=CARTESIAN_POINT('Ctrl Pts',(69.4892247478019,211.678623976047,23.4913203435596)) ;
#79129=CARTESIAN_POINT('Ctrl Pts',(69.4892247478019,211.678623976047,31.6033203435596)) ;
#79130=CARTESIAN_POINT('Ctrl Pts',(69.4984736650468,211.623322295552,23.4913203435596)) ;
#79131=CARTESIAN_POINT('Ctrl Pts',(69.4984736650468,211.623322295552,31.6033203435596)) ;
#79132=CARTESIAN_POINT('',(69.2315751790255,211.872432002476,30.2513203435596)) ;
#79133=CARTESIAN_POINT('',(69.4984736650468,211.623322295552,23.4913203435596)) ;
#79134=CARTESIAN_POINT('Origin',(62.4092970952969,212.53483522599,23.8713203435596)) ;
#79135=CARTESIAN_POINT('Ctrl Pts',(72.3111547045756,202.05583548982,30.2513203435596)) ;
#79136=CARTESIAN_POINT('Ctrl Pts',(72.3111547045756,202.05583548982,22.1393203435596)) ;
#79137=CARTESIAN_POINT('Ctrl Pts',(72.3696846119161,202.05583548982,30.2513203435596)) ;
#79138=CARTESIAN_POINT('Ctrl Pts',(72.3696846119161,202.05583548982,22.1393203435596)) ;
#79139=CARTESIAN_POINT('Ctrl Pts',(72.4861965697617,202.091073258586,30.2513203435596)) ;
#79140=CARTESIAN_POINT('Ctrl Pts',(72.4861965697617,202.091073258586,22.1393203435596)) ;
#79141=CARTESIAN_POINT('Ctrl Pts',(72.6234348552125,202.255646958551,30.2513203435596)) ;
#79142=CARTESIAN_POINT('Ctrl Pts',(72.6234348552125,202.255646958551,22.1393203435596)) ;
#79143=CARTESIAN_POINT('Ctrl Pts',(72.6179307032035,202.415805684798,30.2513203435596)) ;
#79144=CARTESIAN_POINT('Ctrl Pts',(72.6179307032035,202.415805684798,22.1393203435596)) ;
#79145=CARTESIAN_POINT('Ctrl Pts',(72.5775641491992,202.49377028534,30.2513203435596)) ;
#79146=CARTESIAN_POINT('Ctrl Pts',(72.5775641491992,202.49377028534,22.1393203435596)) ;
#79147=CARTESIAN_POINT('',(72.5775641491992,202.49377028534,30.2513203435596)) ;
#79148=CARTESIAN_POINT('Ctrl Pts',(73.7436956568153,200.410454788892,30.2513203435596)) ;
#79149=CARTESIAN_POINT('Ctrl Pts',(73.7436956568153,200.410454788892,22.1393203435596)) ;
#79150=CARTESIAN_POINT('Ctrl Pts',(73.6906445023934,200.49866288572,30.2513203435596)) ;
#79151=CARTESIAN_POINT('Ctrl Pts',(73.6906445023934,200.49866288572,22.1393203435596)) ;
#79152=CARTESIAN_POINT('Ctrl Pts',(73.5895427859729,200.55583548982,30.2513203435596)) ;
#79153=CARTESIAN_POINT('Ctrl Pts',(73.5895427859729,200.55583548982,22.1393203435596)) ;
#79154=CARTESIAN_POINT('Ctrl Pts',(73.4866103162092,200.55583548982,30.2513203435596)) ;
#79155=CARTESIAN_POINT('Ctrl Pts',(73.4866103162092,200.55583548982,22.1393203435596)) ;
#79156=CARTESIAN_POINT('',(73.4866103162092,200.55583548982,30.2513203435596)) ;
#79157=CARTESIAN_POINT('Ctrl Pts',(77.8285014478222,189.289539758744,17.9913203435596)) ;
#79158=CARTESIAN_POINT('Ctrl Pts',(77.8285014478222,189.289539758744,32.7033203435596)) ;
#79159=CARTESIAN_POINT('Ctrl Pts',(77.5774223547909,189.289539758744,17.9913203435596)) ;
#79160=CARTESIAN_POINT('Ctrl Pts',(77.5774223547909,189.289539758744,32.7033203435596)) ;
#79161=CARTESIAN_POINT('Ctrl Pts',(77.3269807962441,189.370827218813,17.9913203435596)) ;
#79162=CARTESIAN_POINT('Ctrl Pts',(77.3269807962441,189.370827218813,32.7033203435596)) ;
#79163=CARTESIAN_POINT('Ctrl Pts',(77.1237619644425,189.518281677405,17.9913203435596)) ;
#79164=CARTESIAN_POINT('Ctrl Pts',(77.1237619644425,189.518281677405,32.7033203435596)) ;
#79165=CARTESIAN_POINT('Ctrl Pts',(73.6566785252795,200.55583548982,17.854339447693)) ;
#79166=CARTESIAN_POINT('Ctrl Pts',(73.6566785252795,200.55583548982,32.8747165227329)) ;
#79167=CARTESIAN_POINT('Ctrl Pts',(75.7001422864503,197.125245060908,17.854339447693)) ;
#79168=CARTESIAN_POINT('Ctrl Pts',(75.7001422864503,197.125245060908,32.8747165227329)) ;
#79169=CARTESIAN_POINT('Ctrl Pts',(78.3842768400396,193.78102322923,17.854339447693)) ;
#79170=CARTESIAN_POINT('Ctrl Pts',(78.3842768400396,193.78102322923,32.8747165227329)) ;
#79171=CARTESIAN_POINT('Ctrl Pts',(81.5507230003364,190.489539758744,17.854339447693)) ;
#79172=CARTESIAN_POINT('Ctrl Pts',(81.5507230003364,190.489539758744,32.8747165227329)) ;
#79173=CARTESIAN_POINT('Origin',(67.6417475736039,200.55583548982,23.8713203435596)) ;
#79174=CARTESIAN_POINT('Ctrl Pts',(69.4614223697787,211.850115187154,17.854339447693)) ;
#79175=CARTESIAN_POINT('Ctrl Pts',(69.4614223697787,211.850115187154,32.8747165227329)) ;
#79176=CARTESIAN_POINT('Ctrl Pts',(69.905975823669,209.06303762573,17.854339447693)) ;
#79177=CARTESIAN_POINT('Ctrl Pts',(69.905975823669,209.06303762573,32.8747165227329)) ;
#79178=CARTESIAN_POINT('Ctrl Pts',(70.7494560159525,206.30693385077,17.854339447693)) ;
#79179=CARTESIAN_POINT('Ctrl Pts',(70.7494560159525,206.30693385077,32.8747165227329)) ;
#79180=CARTESIAN_POINT('Ctrl Pts',(72.0309081730459,203.597341394065,17.854339447693)) ;
#79181=CARTESIAN_POINT('Ctrl Pts',(72.0309081730459,203.597341394065,32.8747165227329)) ;
#79182=CARTESIAN_POINT('Ctrl Pts',(72.2749463865981,203.081329852839,17.854339447693)) ;
#79183=CARTESIAN_POINT('Ctrl Pts',(72.2749463865981,203.081329852839,32.8747165227329)) ;
#79184=CARTESIAN_POINT('Ctrl Pts',(72.5341913976221,202.567520362575,17.854339447693)) ;
#79185=CARTESIAN_POINT('Ctrl Pts',(72.5341913976221,202.567520362575,32.8747165227329)) ;
#79186=CARTESIAN_POINT('Ctrl Pts',(72.8081914673101,202.05583548982,17.854339447693)) ;
#79187=CARTESIAN_POINT('Ctrl Pts',(72.8081914673101,202.05583548982,32.8747165227329)) ;
#79188=CARTESIAN_POINT('Origin',(61.7916108526749,215.420902931566,23.8713203435596)) ;
#79189=CARTESIAN_POINT('',(61.7916108526749,217.432246240363,23.8713203435596)) ;
#79190=CARTESIAN_POINT('Origin',(69.6705101448823,217.61928420644,23.8713203435596)) ;
#79191=CARTESIAN_POINT('Origin',(64.1568347953872,220.146231446812,23.8713203435596)) ;
#79192=CARTESIAN_POINT('',(69.1892193809281,219.722291984294,23.8713203435596)) ;
#79193=CARTESIAN_POINT('Origin',(67.7485452644419,219.902067758924,23.8713203435596)) ;
#79194=CARTESIAN_POINT('',(67.7485452644419,219.902067758924,23.8713203435596)) ;
#79195=CARTESIAN_POINT('Origin',(64.1568347953872,220.146231446812,23.8713203435596)) ;
#79196=CARTESIAN_POINT('Origin',(64.1568347953872,220.146231446812,23.8713203435596)) ;
#117127=UNCERTAINTY_MEASURE_WITH_UNIT(LENGTH_MEASURE(0.01),#117171,
'DISTANCE_ACCURACY_VALUE',
'Maximum model space distance between geometric entities at asserted c
onnectivities') ;
#117147=UNCERTAINTY_MEASURE_WITH_UNIT(LENGTH_MEASURE(0.01),#117171,
'DISTANCE_ACCURACY_VALUE',
'Maximum model space distance between geometric entities at asserted c
onnectivities') ;
#117150=(
GEOMETRIC_REPRESENTATION_CONTEXT(3)
GLOBAL_UNCERTAINTY_ASSIGNED_CONTEXT((#117127))
GLOBAL_UNIT_ASSIGNED_CONTEXT((#117171,#117173,#117174))
REPRESENTATION_CONTEXT('','3D')
) ;
#117170=(
GEOMETRIC_REPRESENTATION_CONTEXT(3)
GLOBAL_UNCERTAINTY_ASSIGNED_CONTEXT((#117147))
GLOBAL_UNIT_ASSIGNED_CONTEXT((#117171,#117173,#117174))
REPRESENTATION_CONTEXT('','3D')
) ;
#117171=(
LENGTH_UNIT()
NAMED_UNIT(*)
SI_UNIT(.MILLI.,.METRE.)
) ;
#117173=(
NAMED_UNIT(*)
PLANE_ANGLE_UNIT()
SI_UNIT($,.RADIAN.)
) ;
#117174=(
NAMED_UNIT(*)
SI_UNIT($,.STERADIAN.)
SOLID_ANGLE_UNIT()
) ;
#117177=SHAPE_DEFINITION_REPRESENTATION(#117199,#117242) ;
#117199=PRODUCT_DEFINITION_SHAPE('',$,#117265) ;
#117242=SHAPE_REPRESENTATION('',(#49866),#117150) ;
#117262=PRODUCT_DEFINITION_CONTEXT('part definition',#117330,'design') ;
#117265=PRODUCT_DEFINITION('Clamp_Handle','Clamp_Handle',#117287,#117262) ;
#117287=PRODUCT_DEFINITION_FORMATION('',$,#117334) ;
#117330=APPLICATION_CONTEXT(
'Core Data for Automotive Mechanical Design Process') ;
#117331=PRODUCT_CONTEXT('part definition',#117330,'mechanical') ;
#117334=PRODUCT('Clamp_Handle','Clamp_Handle',$,(#117331)) ;
#117355=PRESENTATION_STYLE_ASSIGNMENT((#117357)) ;
#117357=SURFACE_STYLE_USAGE(.BOTH.,#117359) ;
#117359=SURFACE_SIDE_STYLE('',(#117361)) ;
#117361=SURFACE_STYLE_FILL_AREA(#117363) ;
#117363=FILL_AREA_STYLE('Opaque(160,160,160)',(#117365)) ;
#117365=FILL_AREA_STYLE_COLOUR('Opaque(160,160,160)',#117367) ;
#117367=COLOUR_RGB('Opaque(160,160,160)', 0.09019608, 0.27058824, 0.51372549) ;
ENDSEC;
END-ISO-10303-21;
